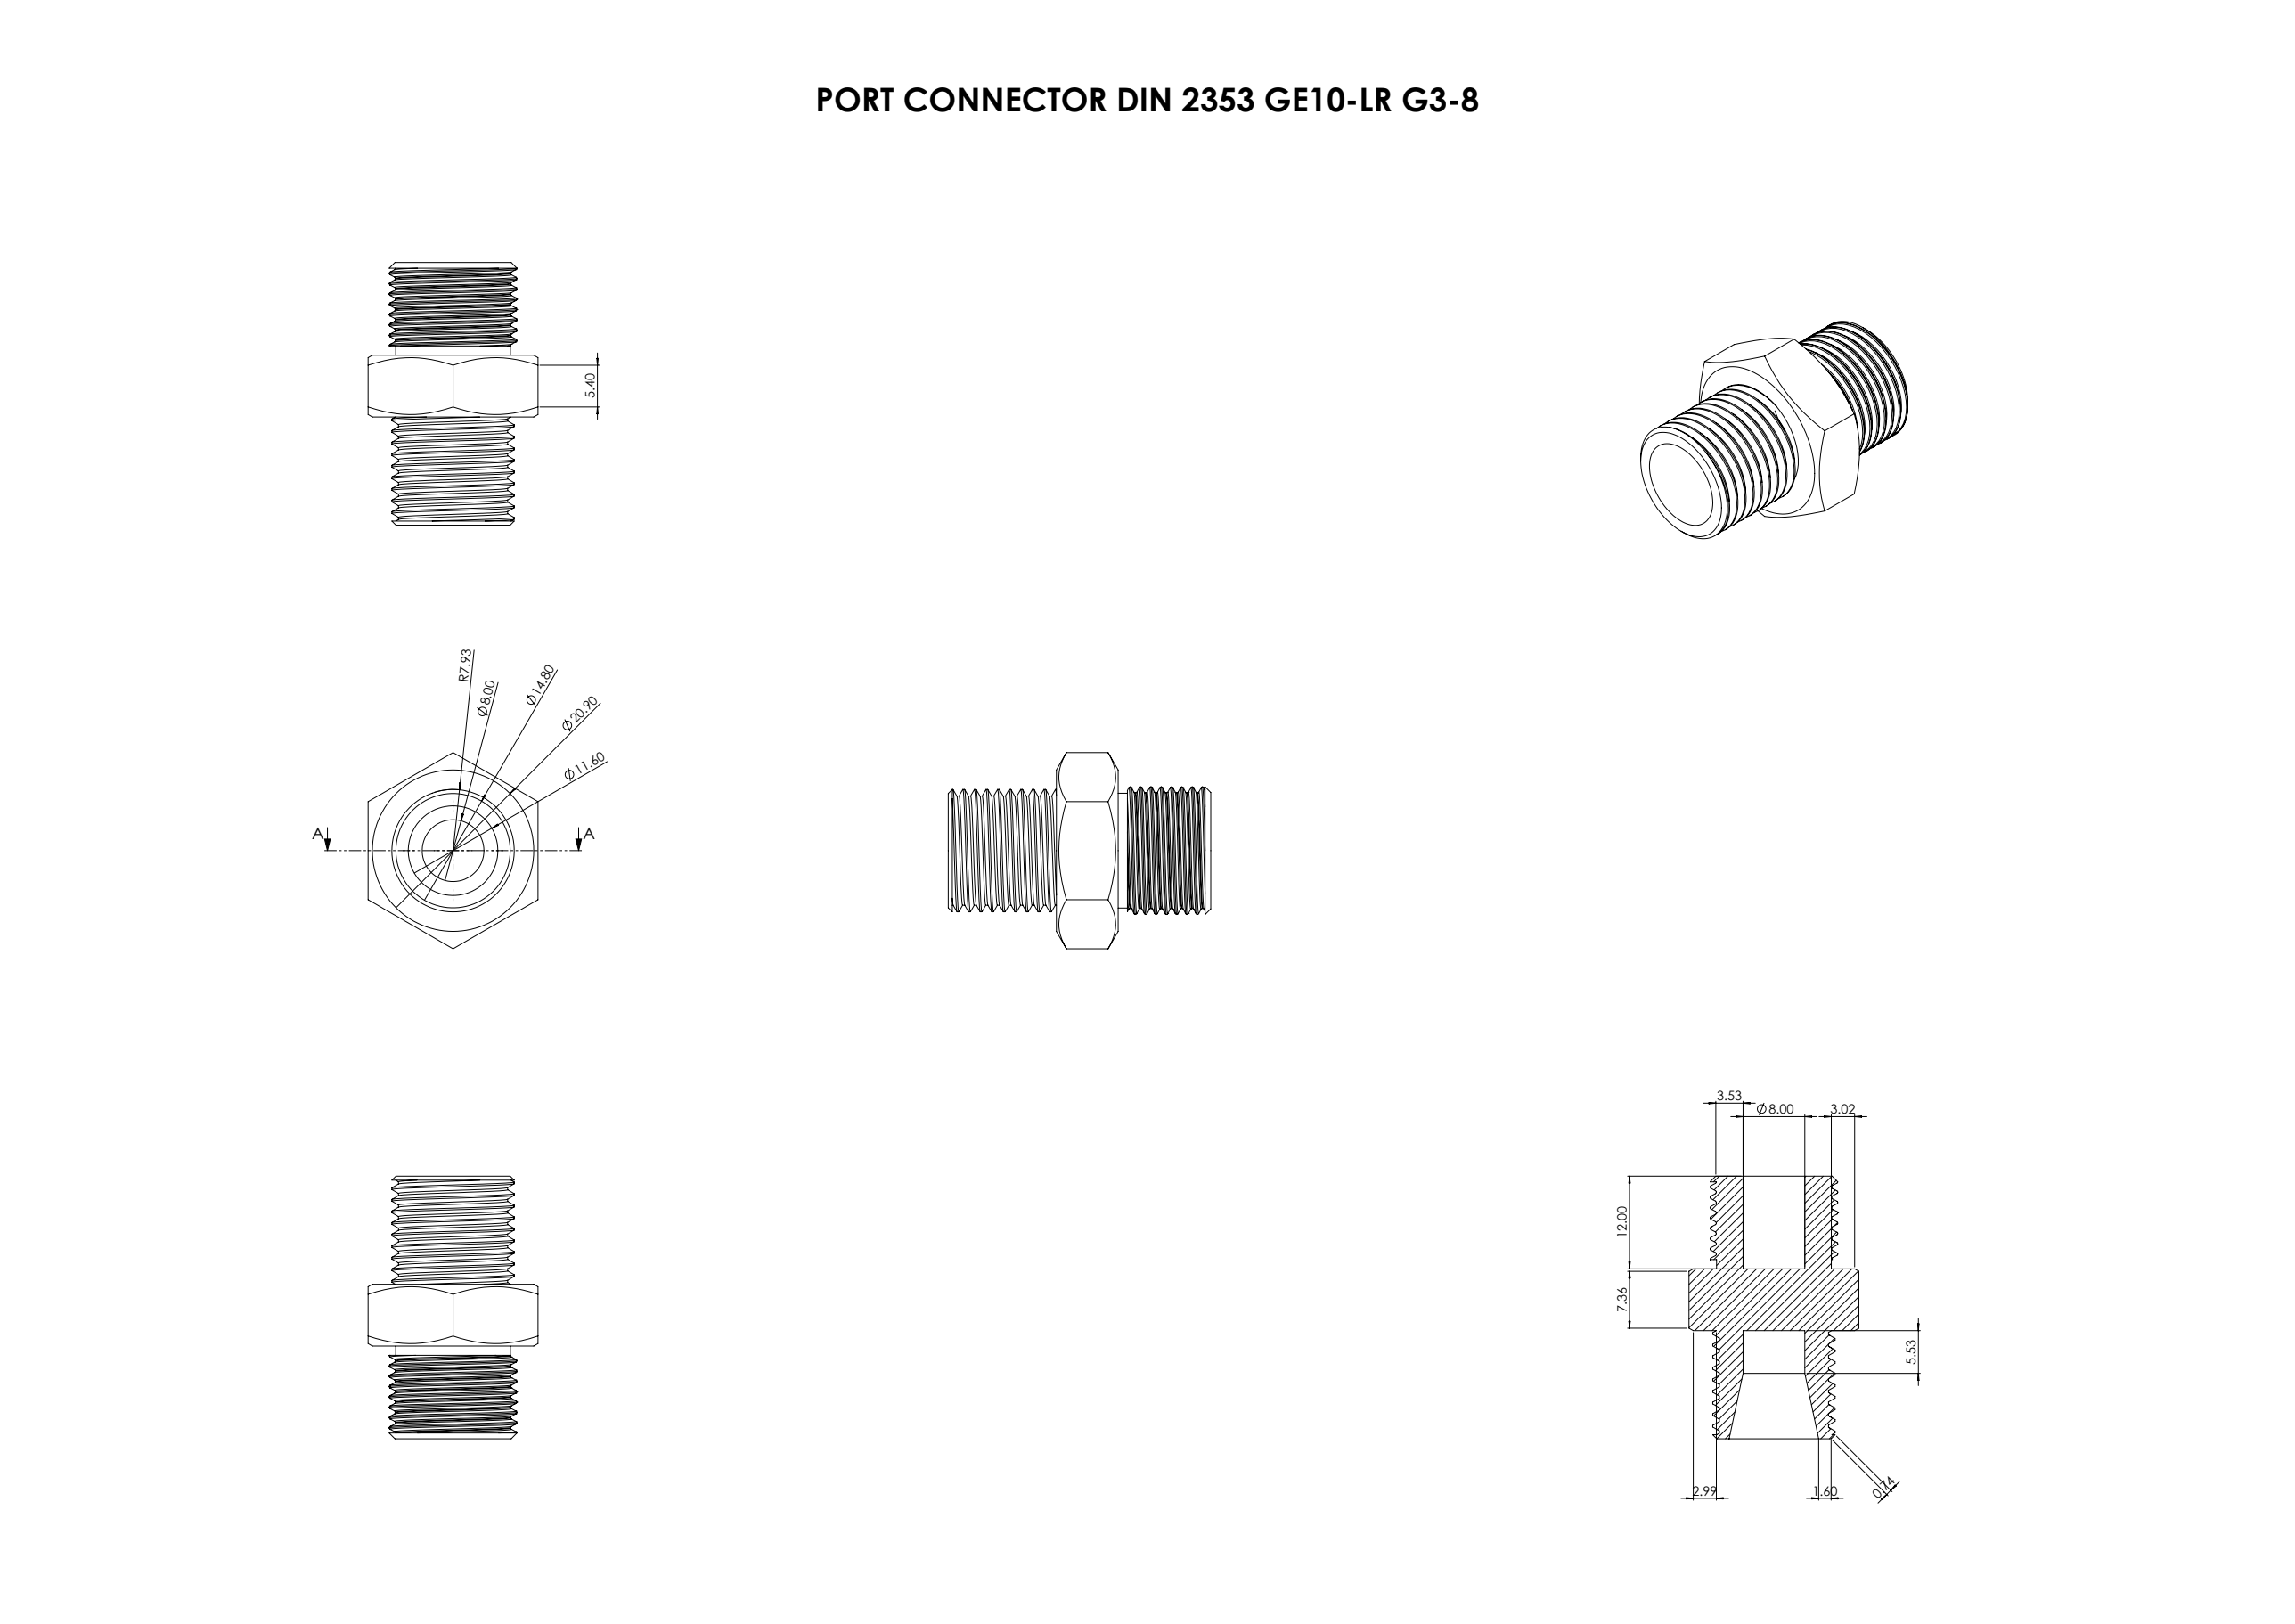
ISO-10303-21;
HEADER;
/* Generated by software containing ST-Developer
 * from STEP Tools, Inc. (www.steptools.com) 
 */

FILE_DESCRIPTION(
/* description */ (''),
/* implementation_level */ '2;1');

FILE_NAME(
/* name */ '20_Port_Connector_DIN_2353_GE10-LR_G3-8.step',
/* time_stamp */ '2026-10-23T00:52:27+05:00',
/* author */ (''),
/* organization */ (''),
/* preprocessor_version */ 'ST-DEVELOPER v20.2',
/* originating_system */ 'Autodesk Translation Framework v15.15.0.0',
/* authorisation */ '');

FILE_SCHEMA (('AUTOMOTIVE_DESIGN { 1 0 10303 214 3 1 1 }'));
ENDSEC;

DATA;
#10=MECHANICAL_DESIGN_GEOMETRIC_PRESENTATION_REPRESENTATION('',(#1574),#59204);
#561=B_SPLINE_SURFACE_WITH_KNOTS('',3,3,((#53988,#53989,#53990,#53991,#53992,
#53993,#53994,#53995,#53996,#53997,#53998,#53999,#54000,#54001,#54002,#54003,
#54004,#54005,#54006,#54007,#54008,#54009,#54010,#54011,#54012,#54013,#54014,
#54015,#54016,#54017,#54018,#54019,#54020,#54021,#54022,#54023,#54024,#54025,
#54026,#54027,#54028,#54029,#54030,#54031,#54032,#54033,#54034,#54035,#54036,
#54037,#54038,#54039,#54040,#54041,#54042,#54043,#54044,#54045,#54046,#54047,
#54048,#54049,#54050,#54051,#54052,#54053,#54054,#54055,#54056,#54057,#54058,
#54059,#54060,#54061,#54062,#54063,#54064,#54065,#54066,#54067,#54068,#54069,
#54070,#54071,#54072,#54073,#54074,#54075,#54076,#54077,#54078,#54079,#54080,
#54081,#54082,#54083,#54084,#54085,#54086,#54087,#54088,#54089,#54090,#54091,
#54092,#54093,#54094,#54095,#54096,#54097,#54098,#54099,#54100,#54101,#54102,
#54103,#54104,#54105,#54106,#54107,#54108),(#54109,#54110,#54111,#54112,
#54113,#54114,#54115,#54116,#54117,#54118,#54119,#54120,#54121,#54122,#54123,
#54124,#54125,#54126,#54127,#54128,#54129,#54130,#54131,#54132,#54133,#54134,
#54135,#54136,#54137,#54138,#54139,#54140,#54141,#54142,#54143,#54144,#54145,
#54146,#54147,#54148,#54149,#54150,#54151,#54152,#54153,#54154,#54155,#54156,
#54157,#54158,#54159,#54160,#54161,#54162,#54163,#54164,#54165,#54166,#54167,
#54168,#54169,#54170,#54171,#54172,#54173,#54174,#54175,#54176,#54177,#54178,
#54179,#54180,#54181,#54182,#54183,#54184,#54185,#54186,#54187,#54188,#54189,
#54190,#54191,#54192,#54193,#54194,#54195,#54196,#54197,#54198,#54199,#54200,
#54201,#54202,#54203,#54204,#54205,#54206,#54207,#54208,#54209,#54210,#54211,
#54212,#54213,#54214,#54215,#54216,#54217,#54218,#54219,#54220,#54221,#54222,
#54223,#54224,#54225,#54226,#54227,#54228,#54229),(#54230,#54231,#54232,
#54233,#54234,#54235,#54236,#54237,#54238,#54239,#54240,#54241,#54242,#54243,
#54244,#54245,#54246,#54247,#54248,#54249,#54250,#54251,#54252,#54253,#54254,
#54255,#54256,#54257,#54258,#54259,#54260,#54261,#54262,#54263,#54264,#54265,
#54266,#54267,#54268,#54269,#54270,#54271,#54272,#54273,#54274,#54275,#54276,
#54277,#54278,#54279,#54280,#54281,#54282,#54283,#54284,#54285,#54286,#54287,
#54288,#54289,#54290,#54291,#54292,#54293,#54294,#54295,#54296,#54297,#54298,
#54299,#54300,#54301,#54302,#54303,#54304,#54305,#54306,#54307,#54308,#54309,
#54310,#54311,#54312,#54313,#54314,#54315,#54316,#54317,#54318,#54319,#54320,
#54321,#54322,#54323,#54324,#54325,#54326,#54327,#54328,#54329,#54330,#54331,
#54332,#54333,#54334,#54335,#54336,#54337,#54338,#54339,#54340,#54341,#54342,
#54343,#54344,#54345,#54346,#54347,#54348,#54349,#54350),(#54351,#54352,
#54353,#54354,#54355,#54356,#54357,#54358,#54359,#54360,#54361,#54362,#54363,
#54364,#54365,#54366,#54367,#54368,#54369,#54370,#54371,#54372,#54373,#54374,
#54375,#54376,#54377,#54378,#54379,#54380,#54381,#54382,#54383,#54384,#54385,
#54386,#54387,#54388,#54389,#54390,#54391,#54392,#54393,#54394,#54395,#54396,
#54397,#54398,#54399,#54400,#54401,#54402,#54403,#54404,#54405,#54406,#54407,
#54408,#54409,#54410,#54411,#54412,#54413,#54414,#54415,#54416,#54417,#54418,
#54419,#54420,#54421,#54422,#54423,#54424,#54425,#54426,#54427,#54428,#54429,
#54430,#54431,#54432,#54433,#54434,#54435,#54436,#54437,#54438,#54439,#54440,
#54441,#54442,#54443,#54444,#54445,#54446,#54447,#54448,#54449,#54450,#54451,
#54452,#54453,#54454,#54455,#54456,#54457,#54458,#54459,#54460,#54461,#54462,
#54463,#54464,#54465,#54466,#54467,#54468,#54469,#54470,#54471)),
 .UNSPECIFIED.,.F.,.F.,.F.,(4,4),(4,1,1,1,1,1,1,1,1,1,1,1,1,1,1,1,1,1,1,
1,1,1,1,1,1,1,1,1,1,1,1,1,1,1,1,1,1,1,1,1,1,1,1,1,1,1,1,1,1,1,1,1,1,1,1,
1,1,1,1,1,1,1,1,1,1,1,1,1,1,1,1,1,1,1,1,1,1,1,1,1,1,1,1,1,1,1,1,1,1,1,1,
1,1,1,1,1,1,1,1,1,1,1,1,1,1,1,1,1,1,1,1,1,1,1,1,1,1,1,4),(0.,0.0989001011121828),
(8.30505915324875,8.80095158446445,9.29684401568014,9.79273644689584,10.2886288781115,
10.7845213093272,11.2804137405429,11.7763061717586,12.2721986029743,12.76809103419,
13.2639834654057,13.7598758966214,14.2557683278371,14.7516607590528,15.2475531902685,
15.7434456214842,16.2393380526999,16.7352304839156,17.2311229151313,17.727015346347,
18.2229077775627,18.7188002087784,19.2146926399941,19.7105850712098,20.2064775024255,
20.7023699336412,21.1982623648568,21.6941547960725,22.1900472272882,22.6859396585039,
23.1818320897196,23.6777245209353,24.173616952151,24.6695093833667,25.1654018145824,
25.6612942457981,26.1571866770138,26.6530791082295,27.1489715394452,27.6448639706609,
28.1407564018766,28.6366488330923,29.132541264308,29.6284336955237,30.1243261267394,
30.6202185579551,31.1161109891708,31.6120034203865,32.1078958516022,32.6037882828178,
33.0996807140335,33.5955731452492,34.0914655764649,34.5873580076806,35.0832504388963,
35.579142870112,36.0750353013277,36.5709277325434,37.0668201637591,37.5627125949748,
38.0586050261905,38.5544974574062,39.0503898886219,39.5462823198376,40.0421747510533,
40.538067182269,41.0339596134847,41.5298520447004,42.0257444759161,42.5216369071318,
43.0175293383475,43.5134217695632,44.0093142007789,44.5052066319946,45.0010990632102,
45.4969914944259,45.9928839256416,46.4887763568573,46.984668788073,47.4805612192887,
47.9764536505044,48.4723460817201,48.9682385129358,49.4641309441515,49.9600233753672,
50.4559158065829,50.9518082377986,51.4477006690143,51.94359310023,52.4394855314457,
52.9353779626614,53.4312703938771,53.9271628250928,54.4230552563085,54.9189476875242,
55.4148401187399,55.9107325499556,56.4066249811712,56.9025174123869,57.3984098436026,
57.8943022748183,58.390194706034,58.8860871372497,59.3819795684654,59.8778719996811,
60.3737644308968,60.8696568621125,61.3655492933282,61.8614417245439,62.3573341557596,
62.8532265869753,63.349119018191,63.8450114494067,64.3409038806224,64.8367963118381,
65.3326887430538,65.8285811742695,66.3244736054852,66.8203660367009),
 .UNSPECIFIED.);
#562=B_SPLINE_SURFACE_WITH_KNOTS('',3,3,((#54612,#54613,#54614,#54615,#54616,
#54617,#54618,#54619,#54620,#54621,#54622,#54623,#54624,#54625,#54626,#54627,
#54628,#54629,#54630,#54631,#54632,#54633,#54634,#54635,#54636,#54637,#54638,
#54639,#54640,#54641,#54642,#54643,#54644,#54645,#54646,#54647,#54648,#54649,
#54650,#54651,#54652,#54653,#54654,#54655,#54656,#54657,#54658,#54659,#54660,
#54661,#54662,#54663,#54664,#54665,#54666,#54667,#54668,#54669,#54670,#54671,
#54672,#54673,#54674,#54675,#54676,#54677,#54678,#54679,#54680,#54681,#54682,
#54683,#54684,#54685,#54686,#54687,#54688,#54689,#54690,#54691,#54692,#54693,
#54694,#54695,#54696,#54697,#54698,#54699,#54700,#54701,#54702,#54703,#54704,
#54705,#54706,#54707,#54708,#54709,#54710,#54711,#54712,#54713,#54714,#54715,
#54716,#54717,#54718,#54719,#54720,#54721,#54722,#54723,#54724,#54725,#54726,
#54727,#54728,#54729,#54730,#54731,#54732),(#54733,#54734,#54735,#54736,
#54737,#54738,#54739,#54740,#54741,#54742,#54743,#54744,#54745,#54746,#54747,
#54748,#54749,#54750,#54751,#54752,#54753,#54754,#54755,#54756,#54757,#54758,
#54759,#54760,#54761,#54762,#54763,#54764,#54765,#54766,#54767,#54768,#54769,
#54770,#54771,#54772,#54773,#54774,#54775,#54776,#54777,#54778,#54779,#54780,
#54781,#54782,#54783,#54784,#54785,#54786,#54787,#54788,#54789,#54790,#54791,
#54792,#54793,#54794,#54795,#54796,#54797,#54798,#54799,#54800,#54801,#54802,
#54803,#54804,#54805,#54806,#54807,#54808,#54809,#54810,#54811,#54812,#54813,
#54814,#54815,#54816,#54817,#54818,#54819,#54820,#54821,#54822,#54823,#54824,
#54825,#54826,#54827,#54828,#54829,#54830,#54831,#54832,#54833,#54834,#54835,
#54836,#54837,#54838,#54839,#54840,#54841,#54842,#54843,#54844,#54845,#54846,
#54847,#54848,#54849,#54850,#54851,#54852,#54853),(#54854,#54855,#54856,
#54857,#54858,#54859,#54860,#54861,#54862,#54863,#54864,#54865,#54866,#54867,
#54868,#54869,#54870,#54871,#54872,#54873,#54874,#54875,#54876,#54877,#54878,
#54879,#54880,#54881,#54882,#54883,#54884,#54885,#54886,#54887,#54888,#54889,
#54890,#54891,#54892,#54893,#54894,#54895,#54896,#54897,#54898,#54899,#54900,
#54901,#54902,#54903,#54904,#54905,#54906,#54907,#54908,#54909,#54910,#54911,
#54912,#54913,#54914,#54915,#54916,#54917,#54918,#54919,#54920,#54921,#54922,
#54923,#54924,#54925,#54926,#54927,#54928,#54929,#54930,#54931,#54932,#54933,
#54934,#54935,#54936,#54937,#54938,#54939,#54940,#54941,#54942,#54943,#54944,
#54945,#54946,#54947,#54948,#54949,#54950,#54951,#54952,#54953,#54954,#54955,
#54956,#54957,#54958,#54959,#54960,#54961,#54962,#54963,#54964,#54965,#54966,
#54967,#54968,#54969,#54970,#54971,#54972,#54973,#54974),(#54975,#54976,
#54977,#54978,#54979,#54980,#54981,#54982,#54983,#54984,#54985,#54986,#54987,
#54988,#54989,#54990,#54991,#54992,#54993,#54994,#54995,#54996,#54997,#54998,
#54999,#55000,#55001,#55002,#55003,#55004,#55005,#55006,#55007,#55008,#55009,
#55010,#55011,#55012,#55013,#55014,#55015,#55016,#55017,#55018,#55019,#55020,
#55021,#55022,#55023,#55024,#55025,#55026,#55027,#55028,#55029,#55030,#55031,
#55032,#55033,#55034,#55035,#55036,#55037,#55038,#55039,#55040,#55041,#55042,
#55043,#55044,#55045,#55046,#55047,#55048,#55049,#55050,#55051,#55052,#55053,
#55054,#55055,#55056,#55057,#55058,#55059,#55060,#55061,#55062,#55063,#55064,
#55065,#55066,#55067,#55068,#55069,#55070,#55071,#55072,#55073,#55074,#55075,
#55076,#55077,#55078,#55079,#55080,#55081,#55082,#55083,#55084,#55085,#55086,
#55087,#55088,#55089,#55090,#55091,#55092,#55093,#55094,#55095)),
 .UNSPECIFIED.,.F.,.F.,.F.,(4,4),(4,1,1,1,1,1,1,1,1,1,1,1,1,1,1,1,1,1,1,
1,1,1,1,1,1,1,1,1,1,1,1,1,1,1,1,1,1,1,1,1,1,1,1,1,1,1,1,1,1,1,1,1,1,1,1,
1,1,1,1,1,1,1,1,1,1,1,1,1,1,1,1,1,1,1,1,1,1,1,1,1,1,1,1,1,1,1,1,1,1,1,1,
1,1,1,1,1,1,1,1,1,1,1,1,1,1,1,1,1,1,1,1,1,1,1,1,1,1,1,4),(0.,0.0989001011121828),
(11.6147305479242,12.1106229791399,12.6065154103556,13.1024078415713,13.598300272787,
14.0941927040027,14.5900851352184,15.0859775664341,15.5818699976498,16.0777624288655,
16.5736548600812,17.0695472912969,17.5654397225126,18.0613321537283,18.557224584944,
19.0531170161597,19.5490094473754,20.0449018785911,20.5407943098068,21.0366867410225,
21.5325791722382,22.0284716034539,22.5243640346695,23.0202564658852,23.5161488971009,
24.0120413283166,24.5079337595323,25.003826190748,25.4997186219637,25.9956110531794,
26.4915034843951,26.9873959156108,27.4832883468265,27.9791807780422,28.4750732092579,
28.9709656404736,29.4668580716893,29.962750502905,30.4586429341207,30.9545353653364,
31.4504277965521,31.9463202277678,32.4422126589835,32.9381050901992,33.4339975214149,
33.9298899526305,34.4257823838462,34.9216748150619,35.4175672462776,35.9134596774933,
36.409352108709,36.9052445399247,37.4011369711404,37.8970294023561,38.3929218335718,
38.8888142647875,39.3847066960032,39.8805991272189,40.3764915584346,40.8723839896503,
41.368276420866,41.8641688520817,42.3600612832974,42.8559537145131,43.3518461457288,
43.8477385769445,44.3436310081602,44.8395234393758,45.3354158705915,45.8313083018072,
46.3272007330229,46.8230931642386,47.3189855954543,47.81487802667,48.3107704578857,
48.8066628891014,49.3025553203171,49.7984477515328,50.2943401827485,50.7902326139642,
51.2861250451799,51.7820174763956,52.2779099076113,52.773802338827,53.2696947700427,
53.7655872012584,54.2614796324741,54.7573720636898,55.2532644949055,55.7491569261211,
56.2450493573368,56.7409417885525,57.2368342197682,57.7327266509839,58.2286190821996,
58.7245115134153,59.220403944631,59.7162963758467,60.2121888070624,60.7080812382781,
61.2039736694938,61.6998661007095,62.1957585319252,62.6916509631409,63.1875433943566,
63.6834358255723,64.179328256788,64.6752206880037,65.1711131192194,65.6670055504351,
66.1628979816508,66.6587904128665,67.1546828440821,67.6505752752978,68.1464677065135,
68.6423601377292,69.1382525689449,69.6341450001606,70.1300374313763),
 .UNSPECIFIED.);
#563=B_SPLINE_SURFACE_WITH_KNOTS('',3,3,((#55202,#55203,#55204,#55205,#55206,
#55207,#55208,#55209,#55210,#55211,#55212,#55213,#55214,#55215,#55216,#55217,
#55218,#55219,#55220,#55221,#55222,#55223,#55224,#55225,#55226,#55227,#55228,
#55229,#55230,#55231,#55232,#55233,#55234,#55235,#55236,#55237,#55238,#55239,
#55240,#55241,#55242,#55243,#55244,#55245,#55246,#55247,#55248,#55249,#55250,
#55251,#55252,#55253,#55254,#55255,#55256,#55257,#55258,#55259,#55260,#55261,
#55262,#55263,#55264,#55265,#55266,#55267,#55268,#55269,#55270,#55271,#55272,
#55273,#55274,#55275,#55276,#55277,#55278,#55279,#55280,#55281,#55282,#55283,
#55284,#55285,#55286,#55287,#55288,#55289,#55290,#55291,#55292,#55293,#55294,
#55295,#55296,#55297,#55298,#55299,#55300,#55301,#55302),(#55303,#55304,
#55305,#55306,#55307,#55308,#55309,#55310,#55311,#55312,#55313,#55314,#55315,
#55316,#55317,#55318,#55319,#55320,#55321,#55322,#55323,#55324,#55325,#55326,
#55327,#55328,#55329,#55330,#55331,#55332,#55333,#55334,#55335,#55336,#55337,
#55338,#55339,#55340,#55341,#55342,#55343,#55344,#55345,#55346,#55347,#55348,
#55349,#55350,#55351,#55352,#55353,#55354,#55355,#55356,#55357,#55358,#55359,
#55360,#55361,#55362,#55363,#55364,#55365,#55366,#55367,#55368,#55369,#55370,
#55371,#55372,#55373,#55374,#55375,#55376,#55377,#55378,#55379,#55380,#55381,
#55382,#55383,#55384,#55385,#55386,#55387,#55388,#55389,#55390,#55391,#55392,
#55393,#55394,#55395,#55396,#55397,#55398,#55399,#55400,#55401,#55402,#55403),
(#55404,#55405,#55406,#55407,#55408,#55409,#55410,#55411,#55412,#55413,
#55414,#55415,#55416,#55417,#55418,#55419,#55420,#55421,#55422,#55423,#55424,
#55425,#55426,#55427,#55428,#55429,#55430,#55431,#55432,#55433,#55434,#55435,
#55436,#55437,#55438,#55439,#55440,#55441,#55442,#55443,#55444,#55445,#55446,
#55447,#55448,#55449,#55450,#55451,#55452,#55453,#55454,#55455,#55456,#55457,
#55458,#55459,#55460,#55461,#55462,#55463,#55464,#55465,#55466,#55467,#55468,
#55469,#55470,#55471,#55472,#55473,#55474,#55475,#55476,#55477,#55478,#55479,
#55480,#55481,#55482,#55483,#55484,#55485,#55486,#55487,#55488,#55489,#55490,
#55491,#55492,#55493,#55494,#55495,#55496,#55497,#55498,#55499,#55500,#55501,
#55502,#55503,#55504),(#55505,#55506,#55507,#55508,#55509,#55510,#55511,
#55512,#55513,#55514,#55515,#55516,#55517,#55518,#55519,#55520,#55521,#55522,
#55523,#55524,#55525,#55526,#55527,#55528,#55529,#55530,#55531,#55532,#55533,
#55534,#55535,#55536,#55537,#55538,#55539,#55540,#55541,#55542,#55543,#55544,
#55545,#55546,#55547,#55548,#55549,#55550,#55551,#55552,#55553,#55554,#55555,
#55556,#55557,#55558,#55559,#55560,#55561,#55562,#55563,#55564,#55565,#55566,
#55567,#55568,#55569,#55570,#55571,#55572,#55573,#55574,#55575,#55576,#55577,
#55578,#55579,#55580,#55581,#55582,#55583,#55584,#55585,#55586,#55587,#55588,
#55589,#55590,#55591,#55592,#55593,#55594,#55595,#55596,#55597,#55598,#55599,
#55600,#55601,#55602,#55603,#55604,#55605),(#55606,#55607,#55608,#55609,
#55610,#55611,#55612,#55613,#55614,#55615,#55616,#55617,#55618,#55619,#55620,
#55621,#55622,#55623,#55624,#55625,#55626,#55627,#55628,#55629,#55630,#55631,
#55632,#55633,#55634,#55635,#55636,#55637,#55638,#55639,#55640,#55641,#55642,
#55643,#55644,#55645,#55646,#55647,#55648,#55649,#55650,#55651,#55652,#55653,
#55654,#55655,#55656,#55657,#55658,#55659,#55660,#55661,#55662,#55663,#55664,
#55665,#55666,#55667,#55668,#55669,#55670,#55671,#55672,#55673,#55674,#55675,
#55676,#55677,#55678,#55679,#55680,#55681,#55682,#55683,#55684,#55685,#55686,
#55687,#55688,#55689,#55690,#55691,#55692,#55693,#55694,#55695,#55696,#55697,
#55698,#55699,#55700,#55701,#55702,#55703,#55704,#55705,#55706)),
 .UNSPECIFIED.,.F.,.F.,.F.,(4,1,4),(4,1,1,1,1,1,1,1,1,1,1,1,1,1,1,1,1,1,
1,1,1,1,1,1,1,1,1,1,1,1,1,1,1,1,1,1,1,1,1,1,1,1,1,1,1,1,1,1,1,1,1,1,1,1,
1,1,1,1,1,1,1,1,1,1,1,1,1,1,1,1,1,1,1,1,1,1,1,1,1,1,1,1,1,1,1,1,1,1,1,1,
1,1,1,1,1,1,1,1,4),(0.,0.467498906784196,1.09083078249646),(6.28318530717955,
6.77358368901883,7.26398207085812,7.7543804526974,8.24477883453668,8.73517721637597,
9.22557559821525,9.71597398005454,10.2063723618938,10.6967707437331,11.1871691255724,
11.6775675074117,12.167965889251,12.6583642710902,13.1487626529295,13.6391610347688,
14.1295594166081,14.6199577984474,15.1103561802867,15.6007545621259,16.0911529439652,
16.5815513258045,17.0719497076438,17.5623480894831,18.0527464713224,18.5431448531616,
19.0335432350009,19.5239416168402,20.0143399986795,20.5047383805188,20.9951367623581,
21.4855351441973,21.9759335260366,22.4663319078759,22.9567302897152,23.4471286715545,
23.9375270533938,24.427925435233,24.9183238170723,25.4087221989116,25.8991205807509,
26.3895189625902,26.8799173444295,27.3703157262687,27.860714108108,28.3511124899473,
28.8415108717866,29.3319092536259,29.8223076354652,30.3127060173044,30.8031043991437,
31.293502780983,31.7839011628223,32.2742995446616,32.7646979265009,33.2550963083402,
33.7454946901794,34.2358930720187,34.726291453858,35.2166898356973,35.7070882175366,
36.1974865993759,36.6878849812151,37.1782833630544,37.6686817448937,38.159080126733,
38.6494785085723,39.1398768904116,39.6302752722508,40.1206736540901,40.6110720359294,
41.1014704177687,41.591868799608,42.0822671814473,42.5726655632865,43.0630639451258,
43.5534623269651,44.0438607088044,44.5342590906437,45.024657472483,45.5150558543222,
46.0054542361615,46.4958526180008,46.9862509998401,47.4766493816794,47.9670477635187,
48.457446145358,48.9478445271972,49.4382429090365,49.9286412908758,50.4190396727151,
50.9094380545544,51.3998364363937,51.8902348182329,52.3806332000722,52.8710315819115,
53.3614299637508,53.8518283455901,54.3422267274294),.UNSPECIFIED.);
#564=B_SPLINE_SURFACE_WITH_KNOTS('',3,3,((#56119,#56120,#56121,#56122,#56123,
#56124,#56125,#56126,#56127,#56128,#56129,#56130,#56131,#56132,#56133,#56134,
#56135,#56136,#56137,#56138,#56139,#56140,#56141,#56142,#56143,#56144,#56145,
#56146,#56147,#56148,#56149,#56150,#56151,#56152,#56153,#56154,#56155,#56156,
#56157,#56158,#56159,#56160,#56161,#56162,#56163,#56164,#56165,#56166,#56167,
#56168,#56169,#56170,#56171,#56172,#56173,#56174,#56175,#56176,#56177,#56178,
#56179,#56180,#56181,#56182,#56183,#56184,#56185,#56186,#56187,#56188,#56189,
#56190,#56191,#56192,#56193,#56194,#56195,#56196,#56197,#56198,#56199,#56200,
#56201,#56202,#56203,#56204,#56205,#56206,#56207,#56208,#56209,#56210,#56211,
#56212,#56213,#56214,#56215,#56216,#56217,#56218,#56219),(#56220,#56221,
#56222,#56223,#56224,#56225,#56226,#56227,#56228,#56229,#56230,#56231,#56232,
#56233,#56234,#56235,#56236,#56237,#56238,#56239,#56240,#56241,#56242,#56243,
#56244,#56245,#56246,#56247,#56248,#56249,#56250,#56251,#56252,#56253,#56254,
#56255,#56256,#56257,#56258,#56259,#56260,#56261,#56262,#56263,#56264,#56265,
#56266,#56267,#56268,#56269,#56270,#56271,#56272,#56273,#56274,#56275,#56276,
#56277,#56278,#56279,#56280,#56281,#56282,#56283,#56284,#56285,#56286,#56287,
#56288,#56289,#56290,#56291,#56292,#56293,#56294,#56295,#56296,#56297,#56298,
#56299,#56300,#56301,#56302,#56303,#56304,#56305,#56306,#56307,#56308,#56309,
#56310,#56311,#56312,#56313,#56314,#56315,#56316,#56317,#56318,#56319,#56320),
(#56321,#56322,#56323,#56324,#56325,#56326,#56327,#56328,#56329,#56330,
#56331,#56332,#56333,#56334,#56335,#56336,#56337,#56338,#56339,#56340,#56341,
#56342,#56343,#56344,#56345,#56346,#56347,#56348,#56349,#56350,#56351,#56352,
#56353,#56354,#56355,#56356,#56357,#56358,#56359,#56360,#56361,#56362,#56363,
#56364,#56365,#56366,#56367,#56368,#56369,#56370,#56371,#56372,#56373,#56374,
#56375,#56376,#56377,#56378,#56379,#56380,#56381,#56382,#56383,#56384,#56385,
#56386,#56387,#56388,#56389,#56390,#56391,#56392,#56393,#56394,#56395,#56396,
#56397,#56398,#56399,#56400,#56401,#56402,#56403,#56404,#56405,#56406,#56407,
#56408,#56409,#56410,#56411,#56412,#56413,#56414,#56415,#56416,#56417,#56418,
#56419,#56420,#56421),(#56422,#56423,#56424,#56425,#56426,#56427,#56428,
#56429,#56430,#56431,#56432,#56433,#56434,#56435,#56436,#56437,#56438,#56439,
#56440,#56441,#56442,#56443,#56444,#56445,#56446,#56447,#56448,#56449,#56450,
#56451,#56452,#56453,#56454,#56455,#56456,#56457,#56458,#56459,#56460,#56461,
#56462,#56463,#56464,#56465,#56466,#56467,#56468,#56469,#56470,#56471,#56472,
#56473,#56474,#56475,#56476,#56477,#56478,#56479,#56480,#56481,#56482,#56483,
#56484,#56485,#56486,#56487,#56488,#56489,#56490,#56491,#56492,#56493,#56494,
#56495,#56496,#56497,#56498,#56499,#56500,#56501,#56502,#56503,#56504,#56505,
#56506,#56507,#56508,#56509,#56510,#56511,#56512,#56513,#56514,#56515,#56516,
#56517,#56518,#56519,#56520,#56521,#56522)),.UNSPECIFIED.,.F.,.F.,.F.,(4,
4),(4,1,1,1,1,1,1,1,1,1,1,1,1,1,1,1,1,1,1,1,1,1,1,1,1,1,1,1,1,1,1,1,1,1,
1,1,1,1,1,1,1,1,1,1,1,1,1,1,1,1,1,1,1,1,1,1,1,1,1,1,1,1,1,1,1,1,1,1,1,1,
1,1,1,1,1,1,1,1,1,1,1,1,1,1,1,1,1,1,1,1,1,1,1,1,1,1,1,1,4),(0.,0.0671853436149873),
(7.04827039213812,7.54574010072061,8.0432098093031,8.54067951788559,9.03814922646808,
9.53561893505058,10.0330886436331,10.5305583522156,11.028028060798,11.5254977693805,
12.022967477963,12.5204371865455,13.017906895128,13.5153766037105,14.012846312293,
14.5103160208755,15.007785729458,15.5052554380405,16.002725146623,16.5001948552054,
16.9976645637879,17.4951342723704,17.9926039809529,18.4900736895354,18.9875433981179,
19.4850131067004,19.9824828152829,20.4799525238654,20.9774222324479,21.4748919410303,
21.9723616496128,22.4698313581953,22.9673010667778,23.4647707753603,23.9622404839428,
24.4597101925253,24.9571799011078,25.4546496096903,25.9521193182728,26.4495890268552,
26.9470587354377,27.4445284440202,27.9419981526027,28.4394678611852,28.9369375697677,
29.4344072783502,29.9318769869327,30.4293466955152,30.9268164040977,31.4242861126801,
31.9217558212626,32.4192255298451,32.9166952384276,33.4141649470101,33.9116346555926,
34.4091043641751,34.9065740727576,35.4040437813401,35.9015134899226,36.3989831985051,
36.8964529070875,37.39392261567,37.8913923242525,38.388862032835,38.8863317414175,
39.38380145,39.8812711585825,40.378740867165,40.8762105757475,41.37368028433,
41.8711499929124,42.3686197014949,42.8660894100774,43.3635591186599,43.8610288272424,
44.3584985358249,44.8559682444074,45.3534379529899,45.8509076615724,46.3483773701549,
46.8458470787373,47.3433167873198,47.8407864959023,48.3382562044848,48.8357259130673,
49.3331956216498,49.8306653302323,50.3281350388148,50.8256047473973,51.3230744559798,
51.8205441645622,52.3180138731447,52.8154835817272,53.3129532903097,53.8104229988922,
54.3078927074747,54.8053624160572,55.3028321246397,55.8003018332222),
 .UNSPECIFIED.);
#565=B_SPLINE_SURFACE_WITH_KNOTS('',3,3,((#56725,#56726,#56727,#56728,#56729,
#56730,#56731,#56732,#56733,#56734,#56735,#56736,#56737,#56738,#56739,#56740,
#56741,#56742,#56743,#56744,#56745,#56746,#56747,#56748,#56749,#56750,#56751,
#56752,#56753,#56754,#56755,#56756,#56757,#56758,#56759,#56760,#56761,#56762,
#56763,#56764,#56765,#56766,#56767,#56768,#56769,#56770,#56771,#56772,#56773,
#56774,#56775,#56776,#56777,#56778,#56779,#56780,#56781,#56782,#56783,#56784,
#56785,#56786,#56787,#56788,#56789,#56790,#56791,#56792,#56793,#56794,#56795,
#56796,#56797,#56798,#56799,#56800,#56801,#56802,#56803,#56804,#56805,#56806,
#56807,#56808,#56809,#56810,#56811,#56812,#56813,#56814,#56815,#56816,#56817,
#56818,#56819,#56820,#56821,#56822,#56823,#56824,#56825),(#56826,#56827,
#56828,#56829,#56830,#56831,#56832,#56833,#56834,#56835,#56836,#56837,#56838,
#56839,#56840,#56841,#56842,#56843,#56844,#56845,#56846,#56847,#56848,#56849,
#56850,#56851,#56852,#56853,#56854,#56855,#56856,#56857,#56858,#56859,#56860,
#56861,#56862,#56863,#56864,#56865,#56866,#56867,#56868,#56869,#56870,#56871,
#56872,#56873,#56874,#56875,#56876,#56877,#56878,#56879,#56880,#56881,#56882,
#56883,#56884,#56885,#56886,#56887,#56888,#56889,#56890,#56891,#56892,#56893,
#56894,#56895,#56896,#56897,#56898,#56899,#56900,#56901,#56902,#56903,#56904,
#56905,#56906,#56907,#56908,#56909,#56910,#56911,#56912,#56913,#56914,#56915,
#56916,#56917,#56918,#56919,#56920,#56921,#56922,#56923,#56924,#56925,#56926),
(#56927,#56928,#56929,#56930,#56931,#56932,#56933,#56934,#56935,#56936,
#56937,#56938,#56939,#56940,#56941,#56942,#56943,#56944,#56945,#56946,#56947,
#56948,#56949,#56950,#56951,#56952,#56953,#56954,#56955,#56956,#56957,#56958,
#56959,#56960,#56961,#56962,#56963,#56964,#56965,#56966,#56967,#56968,#56969,
#56970,#56971,#56972,#56973,#56974,#56975,#56976,#56977,#56978,#56979,#56980,
#56981,#56982,#56983,#56984,#56985,#56986,#56987,#56988,#56989,#56990,#56991,
#56992,#56993,#56994,#56995,#56996,#56997,#56998,#56999,#57000,#57001,#57002,
#57003,#57004,#57005,#57006,#57007,#57008,#57009,#57010,#57011,#57012,#57013,
#57014,#57015,#57016,#57017,#57018,#57019,#57020,#57021,#57022,#57023,#57024,
#57025,#57026,#57027),(#57028,#57029,#57030,#57031,#57032,#57033,#57034,
#57035,#57036,#57037,#57038,#57039,#57040,#57041,#57042,#57043,#57044,#57045,
#57046,#57047,#57048,#57049,#57050,#57051,#57052,#57053,#57054,#57055,#57056,
#57057,#57058,#57059,#57060,#57061,#57062,#57063,#57064,#57065,#57066,#57067,
#57068,#57069,#57070,#57071,#57072,#57073,#57074,#57075,#57076,#57077,#57078,
#57079,#57080,#57081,#57082,#57083,#57084,#57085,#57086,#57087,#57088,#57089,
#57090,#57091,#57092,#57093,#57094,#57095,#57096,#57097,#57098,#57099,#57100,
#57101,#57102,#57103,#57104,#57105,#57106,#57107,#57108,#57109,#57110,#57111,
#57112,#57113,#57114,#57115,#57116,#57117,#57118,#57119,#57120,#57121,#57122,
#57123,#57124,#57125,#57126,#57127,#57128),(#57129,#57130,#57131,#57132,
#57133,#57134,#57135,#57136,#57137,#57138,#57139,#57140,#57141,#57142,#57143,
#57144,#57145,#57146,#57147,#57148,#57149,#57150,#57151,#57152,#57153,#57154,
#57155,#57156,#57157,#57158,#57159,#57160,#57161,#57162,#57163,#57164,#57165,
#57166,#57167,#57168,#57169,#57170,#57171,#57172,#57173,#57174,#57175,#57176,
#57177,#57178,#57179,#57180,#57181,#57182,#57183,#57184,#57185,#57186,#57187,
#57188,#57189,#57190,#57191,#57192,#57193,#57194,#57195,#57196,#57197,#57198,
#57199,#57200,#57201,#57202,#57203,#57204,#57205,#57206,#57207,#57208,#57209,
#57210,#57211,#57212,#57213,#57214,#57215,#57216,#57217,#57218,#57219,#57220,
#57221,#57222,#57223,#57224,#57225,#57226,#57227,#57228,#57229)),
 .UNSPECIFIED.,.F.,.F.,.F.,(4,1,4),(4,1,1,1,1,1,1,1,1,1,1,1,1,1,1,1,1,1,
1,1,1,1,1,1,1,1,1,1,1,1,1,1,1,1,1,1,1,1,1,1,1,1,1,1,1,1,1,1,1,1,1,1,1,1,
1,1,1,1,1,1,1,1,1,1,1,1,1,1,1,1,1,1,1,1,1,1,1,1,1,1,1,1,1,1,1,1,1,1,1,1,
1,1,1,1,1,1,1,1,4),(0.,0.467498906784196,1.09083078249646),(8.50634549793093,
8.99674387977021,9.4871422616095,9.97754064344878,10.4679390252881,10.9583374071273,
11.4487357889666,11.9391341708059,12.4295325526452,12.9199309344845,13.4103293163238,
13.9007276981631,14.3911260800023,14.8815244618416,15.3719228436809,15.8623212255202,
16.3527196073595,16.8431179891988,17.333516371038,17.8239147528773,18.3143131347166,
18.8047115165559,19.2951098983952,19.7855082802345,20.2759066620737,20.766305043913,
21.2567034257523,21.7471018075916,22.2375001894309,22.7278985712702,23.2182969531094,
23.7086953349487,24.199093716788,24.6894920986273,25.1798904804666,25.6702888623059,
26.1606872441451,26.6510856259844,27.1414840078237,27.631882389663,28.1222807715023,
28.6126791533416,29.1030775351808,29.5934759170201,30.0838742988594,30.5742726806987,
31.064671062538,31.5550694443773,32.0454678262166,32.5358662080558,33.0262645898951,
33.5166629717344,34.0070613535737,34.497459735413,34.9878581172523,35.4782564990915,
35.9686548809308,36.4590532627701,36.9494516446094,37.4398500264487,37.930248408288,
38.4206467901272,38.9110451719665,39.4014435538058,39.8918419356451,40.3822403174844,
40.8726386993237,41.3630370811629,41.8534354630022,42.3438338448415,42.8342322266808,
43.3246306085201,43.8150289903594,44.3054273721986,44.7958257540379,45.2862241358772,
45.7766225177165,46.2670208995558,46.7574192813951,47.2478176632343,47.7382160450736,
48.2286144269129,48.7190128087522,49.2094111905915,49.6998095724308,50.1902079542701,
50.6806063361093,51.1710047179486,51.6614030997879,52.1518014816272,52.6421998634665,
53.1325982453058,53.622996627145,54.1133950089843,54.6037933908236,55.0941917726629,
55.5845901545022,56.0749885363415,56.5653869181807),.UNSPECIFIED.);
#566=B_SPLINE_SURFACE_WITH_KNOTS('',3,3,((#57322,#57323,#57324,#57325,#57326,
#57327,#57328,#57329,#57330,#57331,#57332,#57333,#57334,#57335,#57336,#57337,
#57338,#57339,#57340,#57341,#57342,#57343,#57344,#57345,#57346,#57347,#57348,
#57349,#57350,#57351,#57352,#57353,#57354,#57355,#57356,#57357,#57358,#57359,
#57360,#57361,#57362,#57363,#57364,#57365,#57366,#57367,#57368,#57369,#57370,
#57371,#57372,#57373,#57374,#57375,#57376,#57377,#57378,#57379,#57380,#57381,
#57382,#57383,#57384,#57385,#57386,#57387,#57388,#57389,#57390,#57391,#57392,
#57393,#57394,#57395,#57396,#57397,#57398,#57399,#57400,#57401,#57402,#57403,
#57404,#57405,#57406,#57407,#57408,#57409,#57410,#57411,#57412,#57413,#57414,
#57415,#57416,#57417,#57418,#57419,#57420,#57421,#57422),(#57423,#57424,
#57425,#57426,#57427,#57428,#57429,#57430,#57431,#57432,#57433,#57434,#57435,
#57436,#57437,#57438,#57439,#57440,#57441,#57442,#57443,#57444,#57445,#57446,
#57447,#57448,#57449,#57450,#57451,#57452,#57453,#57454,#57455,#57456,#57457,
#57458,#57459,#57460,#57461,#57462,#57463,#57464,#57465,#57466,#57467,#57468,
#57469,#57470,#57471,#57472,#57473,#57474,#57475,#57476,#57477,#57478,#57479,
#57480,#57481,#57482,#57483,#57484,#57485,#57486,#57487,#57488,#57489,#57490,
#57491,#57492,#57493,#57494,#57495,#57496,#57497,#57498,#57499,#57500,#57501,
#57502,#57503,#57504,#57505,#57506,#57507,#57508,#57509,#57510,#57511,#57512,
#57513,#57514,#57515,#57516,#57517,#57518,#57519,#57520,#57521,#57522,#57523),
(#57524,#57525,#57526,#57527,#57528,#57529,#57530,#57531,#57532,#57533,
#57534,#57535,#57536,#57537,#57538,#57539,#57540,#57541,#57542,#57543,#57544,
#57545,#57546,#57547,#57548,#57549,#57550,#57551,#57552,#57553,#57554,#57555,
#57556,#57557,#57558,#57559,#57560,#57561,#57562,#57563,#57564,#57565,#57566,
#57567,#57568,#57569,#57570,#57571,#57572,#57573,#57574,#57575,#57576,#57577,
#57578,#57579,#57580,#57581,#57582,#57583,#57584,#57585,#57586,#57587,#57588,
#57589,#57590,#57591,#57592,#57593,#57594,#57595,#57596,#57597,#57598,#57599,
#57600,#57601,#57602,#57603,#57604,#57605,#57606,#57607,#57608,#57609,#57610,
#57611,#57612,#57613,#57614,#57615,#57616,#57617,#57618,#57619,#57620,#57621,
#57622,#57623,#57624),(#57625,#57626,#57627,#57628,#57629,#57630,#57631,
#57632,#57633,#57634,#57635,#57636,#57637,#57638,#57639,#57640,#57641,#57642,
#57643,#57644,#57645,#57646,#57647,#57648,#57649,#57650,#57651,#57652,#57653,
#57654,#57655,#57656,#57657,#57658,#57659,#57660,#57661,#57662,#57663,#57664,
#57665,#57666,#57667,#57668,#57669,#57670,#57671,#57672,#57673,#57674,#57675,
#57676,#57677,#57678,#57679,#57680,#57681,#57682,#57683,#57684,#57685,#57686,
#57687,#57688,#57689,#57690,#57691,#57692,#57693,#57694,#57695,#57696,#57697,
#57698,#57699,#57700,#57701,#57702,#57703,#57704,#57705,#57706,#57707,#57708,
#57709,#57710,#57711,#57712,#57713,#57714,#57715,#57716,#57717,#57718,#57719,
#57720,#57721,#57722,#57723,#57724,#57725),(#57726,#57727,#57728,#57729,
#57730,#57731,#57732,#57733,#57734,#57735,#57736,#57737,#57738,#57739,#57740,
#57741,#57742,#57743,#57744,#57745,#57746,#57747,#57748,#57749,#57750,#57751,
#57752,#57753,#57754,#57755,#57756,#57757,#57758,#57759,#57760,#57761,#57762,
#57763,#57764,#57765,#57766,#57767,#57768,#57769,#57770,#57771,#57772,#57773,
#57774,#57775,#57776,#57777,#57778,#57779,#57780,#57781,#57782,#57783,#57784,
#57785,#57786,#57787,#57788,#57789,#57790,#57791,#57792,#57793,#57794,#57795,
#57796,#57797,#57798,#57799,#57800,#57801,#57802,#57803,#57804,#57805,#57806,
#57807,#57808,#57809,#57810,#57811,#57812,#57813,#57814,#57815,#57816,#57817,
#57818,#57819,#57820,#57821,#57822,#57823,#57824,#57825,#57826)),
 .UNSPECIFIED.,.F.,.F.,.F.,(4,1,4),(4,1,1,1,1,1,1,1,1,1,1,1,1,1,1,1,1,1,
1,1,1,1,1,1,1,1,1,1,1,1,1,1,1,1,1,1,1,1,1,1,1,1,1,1,1,1,1,1,1,1,1,1,1,1,
1,1,1,1,1,1,1,1,1,1,1,1,1,1,1,1,1,1,1,1,1,1,1,1,1,1,1,1,1,1,1,1,1,1,1,1,
1,1,1,1,1,1,1,1,4),(-1.09083078249646,-0.623331875712262,0.),(9.57812533864917,
10.0685237204885,10.5589221023277,11.049320484167,11.5397188660063,12.0301172478456,
12.5205156296849,13.0109140115242,13.5013123933634,13.9917107752027,14.482109157042,
14.9725075388813,15.4629059207206,15.9533043025599,16.4437026843991,16.9341010662384,
17.4244994480777,17.914897829917,18.4052962117563,18.8956945935956,19.3860929754348,
19.8764913572741,20.3668897391134,20.8572881209527,21.347686502792,21.8380848846313,
22.3284832664706,22.8188816483098,23.3092800301491,23.7996784119884,24.2900767938277,
24.780475175667,25.2708735575063,25.7612719393455,26.2516703211848,26.7420687030241,
27.2324670848634,27.7228654667027,28.213263848542,28.7036622303812,29.1940606122205,
29.6844589940598,30.1748573758991,30.6652557577384,31.1556541395777,31.6460525214169,
32.1364509032562,32.6268492850955,33.1172476669348,33.6076460487741,34.0980444306134,
34.5884428124527,35.0788411942919,35.5692395761312,36.0596379579705,36.5500363398098,
37.0404347216491,37.5308331034883,38.0212314853276,38.5116298671669,39.0020282490062,
39.4924266308455,39.9828250126848,40.4732233945241,40.9636217763633,41.4540201582026,
41.9444185400419,42.4348169218812,42.9252153037205,43.4156136855598,43.906012067399,
44.3964104492383,44.8868088310776,45.3772072129169,45.8676055947562,46.3580039765955,
46.8484023584347,47.338800740274,47.8291991221133,48.3195975039526,48.8099958857919,
49.3003942676312,49.7907926494704,50.2811910313097,50.771589413149,51.2619877949883,
51.7523861768276,52.2427845586669,52.7331829405062,53.2235813223454,53.7139797041847,
54.204378086024,54.6947764678633,55.1851748497026,55.6755732315419,56.1659716133811,
56.6563699952204,57.1467683770597,57.637166758899),.UNSPECIFIED.);
#567=B_SPLINE_SURFACE_WITH_KNOTS('',3,3,((#57934,#57935,#57936,#57937,#57938,
#57939,#57940,#57941,#57942,#57943,#57944,#57945,#57946,#57947,#57948,#57949,
#57950,#57951,#57952,#57953,#57954,#57955,#57956,#57957,#57958,#57959,#57960,
#57961,#57962,#57963,#57964,#57965,#57966,#57967,#57968,#57969,#57970,#57971,
#57972,#57973,#57974,#57975,#57976,#57977,#57978,#57979,#57980,#57981,#57982,
#57983,#57984,#57985,#57986,#57987,#57988,#57989,#57990,#57991,#57992,#57993,
#57994,#57995,#57996,#57997,#57998,#57999,#58000,#58001,#58002,#58003,#58004,
#58005,#58006,#58007,#58008,#58009,#58010,#58011,#58012,#58013,#58014,#58015,
#58016,#58017,#58018,#58019,#58020,#58021,#58022,#58023,#58024,#58025,#58026,
#58027,#58028,#58029,#58030,#58031,#58032,#58033,#58034),(#58035,#58036,
#58037,#58038,#58039,#58040,#58041,#58042,#58043,#58044,#58045,#58046,#58047,
#58048,#58049,#58050,#58051,#58052,#58053,#58054,#58055,#58056,#58057,#58058,
#58059,#58060,#58061,#58062,#58063,#58064,#58065,#58066,#58067,#58068,#58069,
#58070,#58071,#58072,#58073,#58074,#58075,#58076,#58077,#58078,#58079,#58080,
#58081,#58082,#58083,#58084,#58085,#58086,#58087,#58088,#58089,#58090,#58091,
#58092,#58093,#58094,#58095,#58096,#58097,#58098,#58099,#58100,#58101,#58102,
#58103,#58104,#58105,#58106,#58107,#58108,#58109,#58110,#58111,#58112,#58113,
#58114,#58115,#58116,#58117,#58118,#58119,#58120,#58121,#58122,#58123,#58124,
#58125,#58126,#58127,#58128,#58129,#58130,#58131,#58132,#58133,#58134,#58135),
(#58136,#58137,#58138,#58139,#58140,#58141,#58142,#58143,#58144,#58145,
#58146,#58147,#58148,#58149,#58150,#58151,#58152,#58153,#58154,#58155,#58156,
#58157,#58158,#58159,#58160,#58161,#58162,#58163,#58164,#58165,#58166,#58167,
#58168,#58169,#58170,#58171,#58172,#58173,#58174,#58175,#58176,#58177,#58178,
#58179,#58180,#58181,#58182,#58183,#58184,#58185,#58186,#58187,#58188,#58189,
#58190,#58191,#58192,#58193,#58194,#58195,#58196,#58197,#58198,#58199,#58200,
#58201,#58202,#58203,#58204,#58205,#58206,#58207,#58208,#58209,#58210,#58211,
#58212,#58213,#58214,#58215,#58216,#58217,#58218,#58219,#58220,#58221,#58222,
#58223,#58224,#58225,#58226,#58227,#58228,#58229,#58230,#58231,#58232,#58233,
#58234,#58235,#58236),(#58237,#58238,#58239,#58240,#58241,#58242,#58243,
#58244,#58245,#58246,#58247,#58248,#58249,#58250,#58251,#58252,#58253,#58254,
#58255,#58256,#58257,#58258,#58259,#58260,#58261,#58262,#58263,#58264,#58265,
#58266,#58267,#58268,#58269,#58270,#58271,#58272,#58273,#58274,#58275,#58276,
#58277,#58278,#58279,#58280,#58281,#58282,#58283,#58284,#58285,#58286,#58287,
#58288,#58289,#58290,#58291,#58292,#58293,#58294,#58295,#58296,#58297,#58298,
#58299,#58300,#58301,#58302,#58303,#58304,#58305,#58306,#58307,#58308,#58309,
#58310,#58311,#58312,#58313,#58314,#58315,#58316,#58317,#58318,#58319,#58320,
#58321,#58322,#58323,#58324,#58325,#58326,#58327,#58328,#58329,#58330,#58331,
#58332,#58333,#58334,#58335,#58336,#58337)),.UNSPECIFIED.,.F.,.F.,.F.,(4,
4),(4,1,1,1,1,1,1,1,1,1,1,1,1,1,1,1,1,1,1,1,1,1,1,1,1,1,1,1,1,1,1,1,1,1,
1,1,1,1,1,1,1,1,1,1,1,1,1,1,1,1,1,1,1,1,1,1,1,1,1,1,1,1,1,1,1,1,1,1,1,1,
1,1,1,1,1,1,1,1,1,1,1,1,1,1,1,1,1,1,1,1,1,1,1,1,1,1,1,1,4),(0.,0.0671853436149873),
(10.3432104236078,10.8406801321902,11.3381498407727,11.8356195493552,12.3330892579377,
12.8305589665202,13.3280286751027,13.8254983836852,14.3229680922677,14.8204378008502,
15.3179075094327,15.8153772180151,16.3128469265976,16.8103166351801,17.3077863437626,
17.8052560523451,18.3027257609276,18.8001954695101,19.2976651780926,19.7951348866751,
20.2926045952576,20.79007430384,21.2875440124225,21.785013721005,22.2824834295875,
22.77995313817,23.2774228467525,23.774892555335,24.2723622639175,24.7698319725,
25.2673016810825,25.7647713896649,26.2622410982474,26.7597108068299,27.2571805154124,
27.7546502239949,28.2521199325774,28.7495896411599,29.2470593497424,29.7445290583249,
30.2419987669074,30.7394684754899,31.2369381840723,31.7344078926548,32.2318776012373,
32.7293473098198,33.2268170184023,33.7242867269848,34.2217564355673,34.7192261441498,
35.2166958527323,35.7141655613148,36.2116352698972,36.7091049784797,37.2065746870622,
37.7040443956447,38.2015141042272,38.6989838128097,39.1964535213922,39.6939232299747,
40.1913929385572,40.6888626471397,41.1863323557221,41.6838020643046,42.1812717728871,
42.6787414814696,43.1762111900521,43.6736808986346,44.1711506072171,44.6686203157996,
45.1660900243821,45.6635597329646,46.1610294415471,46.6584991501295,47.155968858712,
47.6534385672945,48.150908275877,48.6483779844595,49.145847693042,49.6433174016245,
50.140787110207,50.6382568187895,51.135726527372,51.6331962359544,52.1306659445369,
52.6281356531194,53.1256053617019,53.6230750702844,54.1205447788669,54.6180144874494,
55.1154841960319,55.6129539046144,56.1104236131969,56.6078933217793,57.1053630303618,
57.6028327389443,58.1003024475268,58.5977721561093,59.0952418646918),
 .UNSPECIFIED.);
#568=B_SPLINE_SURFACE_WITH_KNOTS('',3,3,((#58490,#58491,#58492,#58493,#58494,
#58495,#58496,#58497,#58498,#58499,#58500,#58501,#58502,#58503,#58504,#58505,
#58506,#58507,#58508,#58509,#58510,#58511,#58512,#58513,#58514,#58515,#58516,
#58517,#58518,#58519,#58520,#58521,#58522,#58523,#58524,#58525,#58526,#58527,
#58528,#58529,#58530,#58531,#58532,#58533,#58534,#58535,#58536,#58537,#58538,
#58539,#58540,#58541,#58542,#58543,#58544,#58545,#58546,#58547,#58548,#58549,
#58550,#58551,#58552,#58553,#58554,#58555,#58556,#58557,#58558,#58559,#58560,
#58561,#58562,#58563,#58564,#58565,#58566,#58567,#58568,#58569,#58570,#58571,
#58572,#58573,#58574,#58575,#58576,#58577,#58578,#58579,#58580,#58581,#58582,
#58583,#58584,#58585,#58586,#58587,#58588,#58589,#58590),(#58591,#58592,
#58593,#58594,#58595,#58596,#58597,#58598,#58599,#58600,#58601,#58602,#58603,
#58604,#58605,#58606,#58607,#58608,#58609,#58610,#58611,#58612,#58613,#58614,
#58615,#58616,#58617,#58618,#58619,#58620,#58621,#58622,#58623,#58624,#58625,
#58626,#58627,#58628,#58629,#58630,#58631,#58632,#58633,#58634,#58635,#58636,
#58637,#58638,#58639,#58640,#58641,#58642,#58643,#58644,#58645,#58646,#58647,
#58648,#58649,#58650,#58651,#58652,#58653,#58654,#58655,#58656,#58657,#58658,
#58659,#58660,#58661,#58662,#58663,#58664,#58665,#58666,#58667,#58668,#58669,
#58670,#58671,#58672,#58673,#58674,#58675,#58676,#58677,#58678,#58679,#58680,
#58681,#58682,#58683,#58684,#58685,#58686,#58687,#58688,#58689,#58690,#58691),
(#58692,#58693,#58694,#58695,#58696,#58697,#58698,#58699,#58700,#58701,
#58702,#58703,#58704,#58705,#58706,#58707,#58708,#58709,#58710,#58711,#58712,
#58713,#58714,#58715,#58716,#58717,#58718,#58719,#58720,#58721,#58722,#58723,
#58724,#58725,#58726,#58727,#58728,#58729,#58730,#58731,#58732,#58733,#58734,
#58735,#58736,#58737,#58738,#58739,#58740,#58741,#58742,#58743,#58744,#58745,
#58746,#58747,#58748,#58749,#58750,#58751,#58752,#58753,#58754,#58755,#58756,
#58757,#58758,#58759,#58760,#58761,#58762,#58763,#58764,#58765,#58766,#58767,
#58768,#58769,#58770,#58771,#58772,#58773,#58774,#58775,#58776,#58777,#58778,
#58779,#58780,#58781,#58782,#58783,#58784,#58785,#58786,#58787,#58788,#58789,
#58790,#58791,#58792),(#58793,#58794,#58795,#58796,#58797,#58798,#58799,
#58800,#58801,#58802,#58803,#58804,#58805,#58806,#58807,#58808,#58809,#58810,
#58811,#58812,#58813,#58814,#58815,#58816,#58817,#58818,#58819,#58820,#58821,
#58822,#58823,#58824,#58825,#58826,#58827,#58828,#58829,#58830,#58831,#58832,
#58833,#58834,#58835,#58836,#58837,#58838,#58839,#58840,#58841,#58842,#58843,
#58844,#58845,#58846,#58847,#58848,#58849,#58850,#58851,#58852,#58853,#58854,
#58855,#58856,#58857,#58858,#58859,#58860,#58861,#58862,#58863,#58864,#58865,
#58866,#58867,#58868,#58869,#58870,#58871,#58872,#58873,#58874,#58875,#58876,
#58877,#58878,#58879,#58880,#58881,#58882,#58883,#58884,#58885,#58886,#58887,
#58888,#58889,#58890,#58891,#58892,#58893),(#58894,#58895,#58896,#58897,
#58898,#58899,#58900,#58901,#58902,#58903,#58904,#58905,#58906,#58907,#58908,
#58909,#58910,#58911,#58912,#58913,#58914,#58915,#58916,#58917,#58918,#58919,
#58920,#58921,#58922,#58923,#58924,#58925,#58926,#58927,#58928,#58929,#58930,
#58931,#58932,#58933,#58934,#58935,#58936,#58937,#58938,#58939,#58940,#58941,
#58942,#58943,#58944,#58945,#58946,#58947,#58948,#58949,#58950,#58951,#58952,
#58953,#58954,#58955,#58956,#58957,#58958,#58959,#58960,#58961,#58962,#58963,
#58964,#58965,#58966,#58967,#58968,#58969,#58970,#58971,#58972,#58973,#58974,
#58975,#58976,#58977,#58978,#58979,#58980,#58981,#58982,#58983,#58984,#58985,
#58986,#58987,#58988,#58989,#58990,#58991,#58992,#58993,#58994)),
 .UNSPECIFIED.,.F.,.F.,.F.,(4,1,4),(4,1,1,1,1,1,1,1,1,1,1,1,1,1,1,1,1,1,
1,1,1,1,1,1,1,1,1,1,1,1,1,1,1,1,1,1,1,1,1,1,1,1,1,1,1,1,1,1,1,1,1,1,1,1,
1,1,1,1,1,1,1,1,1,1,1,1,1,1,1,1,1,1,1,1,1,1,1,1,1,1,1,1,1,1,1,1,1,1,1,1,
1,1,1,1,1,1,1,1,4),(-1.09083078249646,-0.623331875712262,0.),(11.8012855294006,
12.2916839112398,12.7820822930791,13.2724806749184,13.7628790567577,14.253277438597,
14.7436758204363,15.2340742022755,15.7244725841148,16.2148709659541,16.7052693477934,
17.1956677296327,17.686066111472,18.1764644933112,18.6668628751505,19.1572612569898,
19.6476596388291,20.1380580206684,20.6284564025077,21.118854784347,21.6092531661862,
22.0996515480255,22.5900499298648,23.0804483117041,23.5708466935434,24.0612450753827,
24.5516434572219,25.0420418390612,25.5324402209005,26.0228386027398,26.5132369845791,
27.0036353664184,27.4940337482576,27.9844321300969,28.4748305119362,28.9652288937755,
29.4556272756148,29.9460256574541,30.4364240392933,30.9268224211326,31.4172208029719,
31.9076191848112,32.3980175666505,32.8884159484898,33.378814330329,33.8692127121683,
34.3596110940076,34.8500094758469,35.3404078576862,35.8308062395255,36.3212046213647,
36.811603003204,37.3020013850433,37.7923997668826,38.2827981487219,38.7731965305612,
39.2635949124004,39.7539932942397,40.244391676079,40.7347900579183,41.2251884397576,
41.7155868215969,42.2059852034361,42.6963835852754,43.1867819671147,43.677180348954,
44.1675787307933,44.6579771126326,45.1483754944719,45.6387738763111,46.1291722581504,
46.6195706399897,47.109969021829,47.6003674036683,48.0907657855076,48.5811641673468,
49.0715625491861,49.5619609310254,50.0523593128647,50.542757694704,51.0331560765433,
51.5235544583825,52.0139528402218,52.5043512220611,52.9947496039004,53.4851479857397,
53.975546367579,54.4659447494182,54.9563431312575,55.4467415130968,55.9371398949361,
56.4275382767754,56.9179366586147,57.4083350404539,57.8987334222932,58.3891318041325,
58.8795301859718,59.3699285678111,59.8603269496504),.UNSPECIFIED.);
#1374=B_SPLINE_CURVE_WITH_KNOTS('',3,(#52488,#52489,#52490,#52491,#52492,
#52493,#52494,#52495,#52496,#52497,#52498),.UNSPECIFIED.,.F.,.F.,(4,1,1,
1,1,1,1,1,4),(53.4070751110265,53.7139797041847,54.204378086024,54.6947764678633,
55.1851748497026,55.6755732315419,56.1659716133811,56.6563699952204,56.8720816739404),
 .UNSPECIFIED.);
#1375=B_SPLINE_CURVE_WITH_KNOTS('',3,(#52501,#52502,#52503,#52504,#52505,
#52506,#52507,#52508,#52509,#52510),.UNSPECIFIED.,.F.,.F.,(4,1,1,1,1,1,
1,4),(53.4070751110265,53.622996627145,54.1133950089843,54.6037933908236,
55.0941917726629,55.5845901545022,56.0749885363415,56.5653869181807),
 .UNSPECIFIED.);
#1376=B_SPLINE_CURVE_WITH_KNOTS('',3,(#52515,#52516,#52517,#52518,#52519,
#52520,#52521,#52522,#52523,#52524,#52525,#52526,#52527,#52528,#52529,#52530,
#52531),.UNSPECIFIED.,.F.,.F.,(4,1,1,1,1,1,1,1,1,1,1,1,1,1,4),(47.1238898038469,
47.338800740274,47.8291991221133,48.3195975039526,48.8099958857919,49.3003942676312,
49.7907926494704,50.2811910313097,50.771589413149,51.2619877949883,51.7523861768276,
52.2427845586669,52.7331829405062,53.2235813223454,53.4070751110265),
 .UNSPECIFIED.);
#1377=B_SPLINE_CURVE_WITH_KNOTS('',3,(#52532,#52533,#52534,#52535,#52536,
#52537,#52538,#52539,#52540,#52541,#52542,#52543,#52544,#52545,#52546,#52547,
#52548),.UNSPECIFIED.,.F.,.F.,(4,1,1,1,1,1,1,1,1,1,1,1,1,1,4),(47.1238898038469,
47.2478176632343,47.7382160450736,48.2286144269129,48.7190128087522,49.2094111905915,
49.6998095724308,50.1902079542701,50.6806063361093,51.1710047179486,51.6614030997879,
52.1518014816272,52.6421998634665,53.1325982453058,53.4070751110265),
 .UNSPECIFIED.);
#1378=B_SPLINE_CURVE_WITH_KNOTS('',3,(#52553,#52554,#52555,#52556,#52557,
#52558,#52559,#52560,#52561,#52562,#52563,#52564,#52565,#52566,#52567,#52568,
#52569),.UNSPECIFIED.,.F.,.F.,(4,1,1,1,1,1,1,1,1,1,1,1,1,1,4),(40.8407044966673,
40.9636217763633,41.4540201582026,41.9444185400419,42.4348169218812,42.9252153037205,
43.4156136855598,43.906012067399,44.3964104492383,44.8868088310776,45.3772072129169,
45.8676055947562,46.3580039765955,46.8484023584347,47.1238898038469),
 .UNSPECIFIED.);
#1379=B_SPLINE_CURVE_WITH_KNOTS('',3,(#52570,#52571,#52572,#52573,#52574,
#52575,#52576,#52577,#52578,#52579,#52580,#52581,#52582,#52583,#52584,#52585,
#52586),.UNSPECIFIED.,.F.,.F.,(4,1,1,1,1,1,1,1,1,1,1,1,1,1,4),(40.8407044966673,
40.8726386993237,41.3630370811629,41.8534354630022,42.3438338448415,42.8342322266808,
43.3246306085201,43.8150289903594,44.3054273721986,44.7958257540379,45.2862241358772,
45.7766225177165,46.2670208995558,46.7574192813951,47.1238898038469),
 .UNSPECIFIED.);
#1380=B_SPLINE_CURVE_WITH_KNOTS('',3,(#52591,#52592,#52593,#52594,#52595,
#52596,#52597,#52598,#52599,#52600,#52601,#52602,#52603,#52604,#52605,#52606,
#52607),.UNSPECIFIED.,.F.,.F.,(4,1,1,1,1,1,1,1,1,1,1,1,1,1,4),(34.5575191894877,
34.5884428124527,35.0788411942919,35.5692395761312,36.0596379579705,36.5500363398098,
37.0404347216491,37.5308331034883,38.0212314853276,38.5116298671669,39.0020282490062,
39.4924266308455,39.9828250126848,40.4732233945241,40.8407044966673),
 .UNSPECIFIED.);
#1381=B_SPLINE_CURVE_WITH_KNOTS('',3,(#52608,#52609,#52610,#52611,#52612,
#52613,#52614,#52615,#52616,#52617,#52618,#52619,#52620,#52621,#52622,#52623),
 .UNSPECIFIED.,.F.,.F.,(4,1,1,1,1,1,1,1,1,1,1,1,1,4),(34.5575191894877,
34.9878581172523,35.4782564990915,35.9686548809308,36.4590532627701,36.9494516446094,
37.4398500264487,37.930248408288,38.4206467901272,38.9110451719665,39.4014435538058,
39.8918419356451,40.3822403174844,40.8407044966673),.UNSPECIFIED.);
#1382=B_SPLINE_CURVE_WITH_KNOTS('',3,(#52628,#52629,#52630,#52631,#52632,
#52633,#52634,#52635,#52636,#52637,#52638,#52639,#52640,#52641,#52642,#52643),
 .UNSPECIFIED.,.F.,.F.,(4,1,1,1,1,1,1,1,1,1,1,1,1,4),(28.2743338823081,
28.7036622303812,29.1940606122205,29.6844589940598,30.1748573758991,30.6652557577384,
31.1556541395777,31.6460525214169,32.1364509032562,32.6268492850955,33.1172476669348,
33.6076460487741,34.0980444306134,34.5575191894877),.UNSPECIFIED.);
#1383=B_SPLINE_CURVE_WITH_KNOTS('',3,(#52644,#52645,#52646,#52647,#52648,
#52649,#52650,#52651,#52652,#52653,#52654,#52655,#52656,#52657,#52658,#52659,
#52660),.UNSPECIFIED.,.F.,.F.,(4,1,1,1,1,1,1,1,1,1,1,1,1,1,4),(28.2743338823081,
28.6126791533416,29.1030775351808,29.5934759170201,30.0838742988594,30.5742726806987,
31.064671062538,31.5550694443773,32.0454678262166,32.5358662080558,33.0262645898951,
33.5166629717344,34.0070613535737,34.497459735413,34.5575191894877),
 .UNSPECIFIED.);
#1384=B_SPLINE_CURVE_WITH_KNOTS('',3,(#52665,#52666,#52667,#52668,#52669,
#52670,#52671,#52672,#52673,#52674,#52675,#52676,#52677,#52678,#52679,#52680,
#52681),.UNSPECIFIED.,.F.,.F.,(4,1,1,1,1,1,1,1,1,1,1,1,1,1,4),(21.9911485751285,
22.3284832664706,22.8188816483098,23.3092800301491,23.7996784119884,24.2900767938277,
24.780475175667,25.2708735575063,25.7612719393455,26.2516703211848,26.7420687030241,
27.2324670848634,27.7228654667027,28.213263848542,28.2743338823081),
 .UNSPECIFIED.);
#1385=B_SPLINE_CURVE_WITH_KNOTS('',3,(#52682,#52683,#52684,#52685,#52686,
#52687,#52688,#52689,#52690,#52691,#52692,#52693,#52694,#52695,#52696,#52697,
#52698),.UNSPECIFIED.,.F.,.F.,(4,1,1,1,1,1,1,1,1,1,1,1,1,1,4),(21.9911485751285,
22.2375001894309,22.7278985712702,23.2182969531094,23.7086953349487,24.199093716788,
24.6894920986273,25.1798904804666,25.6702888623059,26.1606872441451,26.6510856259844,
27.1414840078237,27.631882389663,28.1222807715023,28.2743338823081),
 .UNSPECIFIED.);
#1386=B_SPLINE_CURVE_WITH_KNOTS('',3,(#52703,#52704,#52705,#52706,#52707,
#52708,#52709,#52710,#52711,#52712,#52713,#52714,#52715,#52716,#52717,#52718,
#52719),.UNSPECIFIED.,.F.,.F.,(4,1,1,1,1,1,1,1,1,1,1,1,1,1,4),(15.7079632679489,
15.9533043025599,16.4437026843991,16.9341010662384,17.4244994480777,17.914897829917,
18.4052962117563,18.8956945935956,19.3860929754348,19.8764913572741,20.3668897391134,
20.8572881209527,21.347686502792,21.8380848846313,21.9911485751285),
 .UNSPECIFIED.);
#1387=B_SPLINE_CURVE_WITH_KNOTS('',3,(#52720,#52721,#52722,#52723,#52724,
#52725,#52726,#52727,#52728,#52729,#52730,#52731,#52732,#52733,#52734,#52735,
#52736),.UNSPECIFIED.,.F.,.F.,(4,1,1,1,1,1,1,1,1,1,1,1,1,1,4),(15.7079632679489,
15.8623212255202,16.3527196073595,16.8431179891988,17.333516371038,17.8239147528773,
18.3143131347166,18.8047115165559,19.2951098983952,19.7855082802345,20.2759066620737,
20.766305043913,21.2567034257523,21.7471018075916,21.9911485751285),
 .UNSPECIFIED.);
#1388=B_SPLINE_CURVE_WITH_KNOTS('',3,(#52743,#52744,#52745,#52746,#52747,
#52748,#52749,#52750,#52751,#52752,#52753,#52754,#52755,#52756,#52757,#52758),
 .UNSPECIFIED.,.F.,.F.,(4,1,1,1,1,1,1,1,1,1,1,1,1,4),(9.57812533864917,
10.0685237204885,10.5589221023277,11.049320484167,11.5397188660063,12.0301172478456,
12.5205156296849,13.0109140115242,13.5013123933634,13.9917107752027,14.482109157042,
14.9725075388813,15.4629059207206,15.7079632679489),.UNSPECIFIED.);
#1389=B_SPLINE_CURVE_WITH_KNOTS('',3,(#52759,#52760,#52761,#52762,#52763,
#52764,#52765,#52766,#52767,#52768,#52769,#52770,#52771,#52772,#52773,#52774,
#52775),.UNSPECIFIED.,.F.,.F.,(4,1,1,1,1,1,1,1,1,1,1,1,1,1,4),(9.42477796076936,
9.4871422616095,9.97754064344878,10.4679390252881,10.9583374071273,11.4487357889666,
11.9391341708059,12.4295325526452,12.9199309344845,13.4103293163238,13.9007276981631,
14.3911260800023,14.8815244618416,15.3719228436809,15.7079632679489),
 .UNSPECIFIED.);
#1390=B_SPLINE_CURVE_WITH_KNOTS('',3,(#52781,#52782,#52783,#52784,#52785,
#52786,#52787,#52788,#52789,#52790,#52791,#52792,#52793,#52794,#52795,#52796),
 .UNSPECIFIED.,.F.,.F.,(4,3,3,3,3,4),(-4.09323272002469,-3.96713944972556,
-3.47124701850987,-2.97535458729417,-2.47946215607848,-2.07135887395548),
 .UNSPECIFIED.);
#1391=B_SPLINE_CURVE_WITH_KNOTS('',3,(#52799,#52800,#52801,#52802,#52803,
#52804,#52805,#52806,#52807,#52808),.UNSPECIFIED.,.F.,.F.,(4,3,3,4),(0.,
0.495892431215694,0.991784862431392,1.11971880752058),.UNSPECIFIED.);
#1392=B_SPLINE_CURVE_WITH_KNOTS('',3,(#52813,#52814,#52815,#52816,#52817,
#52818,#52819,#52820,#52821,#52822,#52823,#52824,#52825,#52826,#52827,#52828,
#52829,#52830,#52831,#52832,#52833,#52834,#52835,#52836,#52837,#52838,#52839,
#52840,#52841,#52842,#52843,#52844,#52845,#52846,#52847,#52848,#52849,#52850,
#52851,#52852),.UNSPECIFIED.,.F.,.F.,(4,3,3,3,3,3,3,3,3,3,3,3,3,4),(-10.3764180272043,
-9.91784862431391,-9.42195619309822,-8.92606376188252,-8.43017133066683,
-7.93427889945113,-7.43838646823544,-6.94249403701974,-6.44660160580404,
-5.95070917458835,-5.45481674337265,-4.95892431215696,-4.46303188094126,
-4.09323272002469),.UNSPECIFIED.);
#1393=B_SPLINE_CURVE_WITH_KNOTS('',3,(#52853,#52854,#52855,#52856,#52857,
#52858,#52859,#52860,#52861,#52862,#52863,#52864,#52865,#52866,#52867,#52868,
#52869,#52870,#52871,#52872,#52873,#52874,#52875,#52876,#52877,#52878,#52879,
#52880,#52881,#52882,#52883,#52884,#52885,#52886,#52887,#52888,#52889,#52890,
#52891,#52892),.UNSPECIFIED.,.F.,.F.,(4,3,3,3,3,3,3,3,3,3,3,3,3,4),(1.11971880752058,
1.48767729364709,1.98356972486278,2.47946215607848,2.97535458729418,3.47124701850987,
3.96713944972557,4.46303188094126,4.95892431215696,5.45481674337265,5.95070917458835,
6.44660160580405,6.94249403701974,7.40290411470016),.UNSPECIFIED.);
#1394=B_SPLINE_CURVE_WITH_KNOTS('',3,(#52897,#52898,#52899,#52900,#52901,
#52902,#52903,#52904,#52905,#52906,#52907,#52908,#52909,#52910,#52911,#52912,
#52913,#52914,#52915,#52916,#52917,#52918,#52919,#52920,#52921,#52922,#52923,
#52924,#52925,#52926,#52927,#52928,#52929,#52930,#52931,#52932,#52933,#52934,
#52935,#52936,#52937,#52938,#52939),.UNSPECIFIED.,.F.,.F.,(4,3,3,3,3,3,
3,3,3,3,3,3,3,3,4),(-16.6596033343839,-16.364450230118,-15.8685577989023,
-15.3726653676866,-14.8767729364709,-14.3808805052552,-13.8849880740395,
-13.3890956428238,-12.8932032116081,-12.3973107803924,-11.9014183491767,
-11.405525917961,-10.9096334867453,-10.4137410555296,-10.3764180272043),
 .UNSPECIFIED.);
#1395=B_SPLINE_CURVE_WITH_KNOTS('',3,(#52940,#52941,#52942,#52943,#52944,
#52945,#52946,#52947,#52948,#52949,#52950,#52951,#52952,#52953,#52954,#52955,
#52956,#52957,#52958,#52959,#52960,#52961,#52962,#52963,#52964,#52965,#52966,
#52967,#52968,#52969,#52970,#52971,#52972,#52973,#52974,#52975,#52976,#52977,
#52978,#52979,#52980,#52981,#52982),.UNSPECIFIED.,.F.,.F.,(4,3,3,3,3,3,
3,3,3,3,3,3,3,3,4),(7.40290411470016,7.43838646823544,7.93427889945113,
8.43017133066683,8.92606376188253,9.42195619309822,9.91784862431392,10.4137410555296,
10.9096334867453,11.405525917961,11.9014183491767,12.3973107803924,12.8932032116081,
13.3890956428238,13.6860894218797),.UNSPECIFIED.);
#1396=B_SPLINE_CURVE_WITH_KNOTS('',3,(#52987,#52988,#52989,#52990,#52991,
#52992,#52993,#52994,#52995,#52996,#52997,#52998,#52999,#53000,#53001,#53002,
#53003,#53004,#53005,#53006,#53007,#53008,#53009,#53010,#53011,#53012,#53013,
#53014,#53015,#53016,#53017,#53018,#53019,#53020,#53021,#53022,#53023,#53024,
#53025,#53026,#53027,#53028,#53029),.UNSPECIFIED.,.F.,.F.,(4,3,3,3,3,3,
3,3,3,3,3,3,3,3,4),(-22.9427886415634,-22.811051835922,-22.3151594047063,
-21.8192669734906,-21.3233745422749,-20.8274821110592,-20.3315896798435,
-19.8356972486278,-19.3398048174121,-18.8439123861964,-18.3480199549807,
-17.852127523765,-17.3562350925493,-16.8603426613336,-16.6596033343839),
 .UNSPECIFIED.);
#1397=B_SPLINE_CURVE_WITH_KNOTS('',3,(#53030,#53031,#53032,#53033,#53034,
#53035,#53036,#53037,#53038,#53039,#53040,#53041,#53042,#53043,#53044,#53045,
#53046,#53047,#53048,#53049,#53050,#53051,#53052,#53053,#53054,#53055,#53056,
#53057,#53058,#53059,#53060,#53061,#53062,#53063,#53064,#53065,#53066,#53067,
#53068,#53069,#53070,#53071,#53072),.UNSPECIFIED.,.F.,.F.,(4,3,3,3,3,3,
3,3,3,3,3,3,3,3,4),(13.6860894218797,13.8849880740395,14.3808805052552,
14.8767729364709,15.3726653676866,15.8685577989023,16.364450230118,16.8603426613337,
17.3562350925494,17.8521275237651,18.3480199549808,18.8439123861965,19.3398048174122,
19.8356972486278,19.9692747290593),.UNSPECIFIED.);
#1398=B_SPLINE_CURVE_WITH_KNOTS('',3,(#53077,#53078,#53079,#53080,#53081,
#53082,#53083,#53084,#53085,#53086,#53087,#53088,#53089,#53090,#53091,#53092,
#53093,#53094,#53095,#53096,#53097,#53098,#53099,#53100,#53101,#53102,#53103,
#53104,#53105,#53106,#53107,#53108,#53109,#53110,#53111,#53112,#53113,#53114,
#53115,#53116),.UNSPECIFIED.,.F.,.F.,(4,3,3,3,3,3,3,3,3,3,3,3,3,4),(-29.225973948743,
-28.7617610105103,-28.2658685792946,-27.7699761480789,-27.2740837168633,
-26.7781912856476,-26.2822988544319,-25.7864064232162,-25.2905139920005,
-24.7946215607848,-24.2987291295691,-23.8028366983534,-23.3069442671377,
-22.9427886415634),.UNSPECIFIED.);
#1399=B_SPLINE_CURVE_WITH_KNOTS('',3,(#53117,#53118,#53119,#53120,#53121,
#53122,#53123,#53124,#53125,#53126,#53127,#53128,#53129,#53130,#53131,#53132,
#53133,#53134,#53135,#53136,#53137,#53138,#53139,#53140,#53141,#53142,#53143,
#53144,#53145,#53146,#53147,#53148,#53149,#53150,#53151,#53152,#53153,#53154,
#53155,#53156),.UNSPECIFIED.,.F.,.F.,(4,3,3,3,3,3,3,3,3,3,3,3,3,4),(19.9692747290593,
20.3315896798435,20.8274821110592,21.3233745422749,21.8192669734906,22.3151594047063,
22.811051835922,23.3069442671377,23.8028366983534,24.2987291295691,24.7946215607848,
25.2905139920005,25.7864064232162,26.2524600362389),.UNSPECIFIED.);
#1400=B_SPLINE_CURVE_WITH_KNOTS('',3,(#53161,#53162,#53163,#53164,#53165,
#53166,#53167,#53168,#53169,#53170,#53171,#53172,#53173,#53174,#53175,#53176,
#53177,#53178,#53179,#53180,#53181,#53182,#53183,#53184,#53185,#53186,#53187,
#53188,#53189,#53190,#53191,#53192,#53193,#53194,#53195,#53196,#53197,#53198,
#53199,#53200,#53201,#53202,#53203),.UNSPECIFIED.,.F.,.F.,(4,3,3,3,3,3,
3,3,3,3,3,3,3,3,4),(-35.5091592559226,-35.2083626163144,-34.7124701850987,
-34.216577753883,-33.7206853226673,-33.2247928914516,-32.7289004602359,
-32.2330080290202,-31.7371155978045,-31.2412231665888,-30.7453307353731,
-30.2494383041574,-29.7535458729417,-29.2576534417261,-29.225973948743),
 .UNSPECIFIED.);
#1401=B_SPLINE_CURVE_WITH_KNOTS('',3,(#53204,#53205,#53206,#53207,#53208,
#53209,#53210,#53211,#53212,#53213,#53214,#53215,#53216,#53217,#53218,#53219,
#53220,#53221,#53222,#53223,#53224,#53225,#53226,#53227,#53228,#53229,#53230,
#53231,#53232,#53233,#53234,#53235,#53236,#53237,#53238,#53239,#53240,#53241,
#53242,#53243,#53244,#53245,#53246),.UNSPECIFIED.,.F.,.F.,(4,3,3,3,3,3,
3,3,3,3,3,3,3,3,4),(26.2524600362389,26.2822988544319,26.7781912856476,
27.2740837168633,27.769976148079,28.2658685792947,28.7617610105104,29.2576534417261,
29.7535458729418,30.2494383041575,30.7453307353731,31.2412231665888,31.7371155978045,
32.2330080290202,32.5356453434185),.UNSPECIFIED.);
#1402=B_SPLINE_CURVE_WITH_KNOTS('',3,(#53251,#53252,#53253,#53254,#53255,
#53256,#53257,#53258,#53259,#53260,#53261,#53262,#53263,#53264,#53265,#53266,
#53267,#53268,#53269,#53270,#53271,#53272,#53273,#53274,#53275,#53276,#53277,
#53278,#53279,#53280,#53281,#53282,#53283,#53284,#53285,#53286,#53287,#53288,
#53289,#53290,#53291,#53292,#53293),.UNSPECIFIED.,.F.,.F.,(4,3,3,3,3,3,
3,3,3,3,3,3,3,3,4),(-41.7923445631022,-41.6549642221184,-41.1590717909027,
-40.663179359687,-40.1672869284713,-39.6713944972556,-39.1755020660399,
-38.6796096348243,-38.1837172036086,-37.6878247723929,-37.1919323411772,
-36.6960399099615,-36.2001474787458,-35.7042550475301,-35.5091592559226),
 .UNSPECIFIED.);
#1403=B_SPLINE_CURVE_WITH_KNOTS('',3,(#53294,#53295,#53296,#53297,#53298,
#53299,#53300,#53301,#53302,#53303,#53304,#53305,#53306,#53307,#53308,#53309,
#53310,#53311,#53312,#53313,#53314,#53315,#53316,#53317,#53318,#53319,#53320,
#53321,#53322,#53323,#53324,#53325,#53326,#53327,#53328,#53329,#53330,#53331,
#53332,#53333,#53334,#53335,#53336),.UNSPECIFIED.,.F.,.F.,(4,3,3,3,3,3,
3,3,3,3,3,3,3,3,4),(32.5356453434185,32.7289004602359,33.2247928914516,
33.7206853226673,34.216577753883,34.7124701850987,35.2083626163144,35.7042550475301,
36.2001474787458,36.6960399099615,37.1919323411772,37.6878247723929,38.1837172036086,
38.6796096348243,38.8188306505981),.UNSPECIFIED.);
#1404=B_SPLINE_CURVE_WITH_KNOTS('',3,(#53341,#53342,#53343,#53344,#53345,
#53346,#53347,#53348,#53349,#53350,#53351,#53352,#53353,#53354,#53355,#53356,
#53357,#53358,#53359,#53360,#53361,#53362,#53363,#53364,#53365,#53366,#53367,
#53368,#53369,#53370,#53371,#53372,#53373,#53374,#53375,#53376,#53377,#53378,
#53379,#53380),.UNSPECIFIED.,.F.,.F.,(4,3,3,3,3,3,3,3,3,3,3,3,3,4),(-48.0755298702818,
-47.6056733967068,-47.1097809654911,-46.6138885342754,-46.1179961030597,
-45.622103671844,-45.1262112406283,-44.6303188094126,-44.1344263781969,
-43.6385339469812,-43.1426415157655,-42.6467490845498,-42.1508566533341,
-41.7923445631022),.UNSPECIFIED.);
#1405=B_SPLINE_CURVE_WITH_KNOTS('',3,(#53381,#53382,#53383,#53384,#53385,
#53386,#53387,#53388,#53389,#53390,#53391,#53392,#53393,#53394,#53395,#53396,
#53397,#53398,#53399,#53400,#53401,#53402,#53403,#53404,#53405,#53406,#53407,
#53408,#53409,#53410,#53411,#53412,#53413,#53414,#53415,#53416,#53417,#53418,
#53419,#53420),.UNSPECIFIED.,.F.,.F.,(4,3,3,3,3,3,3,3,3,3,3,3,3,4),(38.8188306505981,
39.17550206604,39.6713944972557,40.1672869284714,40.6631793596871,41.1590717909028,
41.6549642221185,42.1508566533342,42.6467490845498,43.1426415157655,43.6385339469812,
44.1344263781969,44.6303188094126,45.1020159577777),.UNSPECIFIED.);
#1406=B_SPLINE_CURVE_WITH_KNOTS('',3,(#53425,#53426,#53427,#53428,#53429,
#53430,#53431,#53432,#53433,#53434,#53435,#53436,#53437,#53438,#53439,#53440,
#53441,#53442,#53443,#53444,#53445,#53446,#53447,#53448,#53449,#53450,#53451,
#53452,#53453,#53454,#53455,#53456,#53457,#53458,#53459,#53460,#53461,#53462,
#53463,#53464,#53465,#53466,#53467),.UNSPECIFIED.,.F.,.F.,(4,3,3,3,3,3,
3,3,3,3,3,3,3,3,4),(-54.3587151774614,-54.0522750025108,-53.5563825712951,
-53.0604901400794,-52.5645977088637,-52.068705277648,-51.5728128464323,
-51.0769204152166,-50.5810279840009,-50.0851355527853,-49.5892431215696,
-49.0933506903539,-48.5974582591382,-48.1015658279225,-48.0755298702818),
 .UNSPECIFIED.);
#1407=B_SPLINE_CURVE_WITH_KNOTS('',3,(#53468,#53469,#53470,#53471,#53472,
#53473,#53474,#53475,#53476,#53477,#53478,#53479,#53480,#53481,#53482,#53483,
#53484,#53485,#53486,#53487,#53488,#53489,#53490,#53491,#53492,#53493,#53494,
#53495,#53496,#53497,#53498,#53499,#53500,#53501,#53502,#53503,#53504,#53505,
#53506,#53507,#53508,#53509,#53510),.UNSPECIFIED.,.F.,.F.,(4,3,3,3,3,3,
3,3,3,3,3,3,3,3,4),(45.1020159577777,45.1262112406283,45.622103671844,46.1179961030597,
46.6138885342754,47.1097809654911,47.6056733967068,48.1015658279225,48.5974582591382,
49.0933506903539,49.5892431215696,50.0851355527853,50.581027984001,51.0769204152167,
51.3852012649573),.UNSPECIFIED.);
#1408=B_SPLINE_CURVE_WITH_KNOTS('',3,(#53516,#53517,#53518,#53519,#53520,
#53521,#53522,#53523),.UNSPECIFIED.,.F.,.F.,(4,1,1,1,1,4),(65.9734457253856,
66.1628979816508,66.6587904128665,67.1546828440821,67.6505752752978,68.0586785574208),
 .UNSPECIFIED.);
#1409=B_SPLINE_CURVE_WITH_KNOTS('',3,(#53526,#53527,#53528,#53529,#53530),
 .UNSPECIFIED.,.F.,.F.,(4,1,4),(65.9734457253857,66.3244736054852,66.8203660367009),
 .UNSPECIFIED.);
#1410=B_SPLINE_CURVE_WITH_KNOTS('',3,(#53535,#53536,#53537,#53538,#53539,
#53540,#53541,#53542,#53543,#53544,#53545,#53546,#53547,#53548,#53549,#53550,
#53551),.UNSPECIFIED.,.F.,.F.,(4,1,1,1,1,1,1,1,1,1,1,1,1,1,4),(59.6902604182061,
59.7162963758467,60.2121888070624,60.7080812382781,61.2039736694938,61.6998661007095,
62.1957585319252,62.6916509631409,63.1875433943566,63.6834358255723,64.179328256788,
64.6752206880037,65.1711131192194,65.6670055504351,65.9734457253856),
 .UNSPECIFIED.);
#1411=B_SPLINE_CURVE_WITH_KNOTS('',3,(#53552,#53553,#53554,#53555,#53556,
#53557,#53558,#53559,#53560,#53561,#53562,#53563,#53564,#53565,#53566,#53567,
#53568),.UNSPECIFIED.,.F.,.F.,(4,1,1,1,1,1,1,1,1,1,1,1,1,1,4),(59.6902604182061,
59.8778719996811,60.3737644308968,60.8696568621125,61.3655492933282,61.8614417245439,
62.3573341557596,62.8532265869753,63.349119018191,63.8450114494067,64.3409038806224,
64.8367963118381,65.3326887430538,65.8285811742695,65.9734457253857),
 .UNSPECIFIED.);
#1412=B_SPLINE_CURVE_WITH_KNOTS('',3,(#53573,#53574,#53575,#53576,#53577,
#53578,#53579,#53580,#53581,#53582,#53583,#53584,#53585,#53586,#53587,#53588),
 .UNSPECIFIED.,.F.,.F.,(4,1,1,1,1,1,1,1,1,1,1,1,1,4),(53.4070751110265,
53.7655872012584,54.2614796324741,54.7573720636898,55.2532644949055,55.7491569261211,
56.2450493573368,56.7409417885525,57.2368342197682,57.7327266509839,58.2286190821996,
58.7245115134153,59.220403944631,59.6902604182061),.UNSPECIFIED.);
#1413=B_SPLINE_CURVE_WITH_KNOTS('',3,(#53589,#53590,#53591,#53592,#53593,
#53594,#53595,#53596,#53597,#53598,#53599,#53600,#53601,#53602,#53603,#53604,
#53605),.UNSPECIFIED.,.F.,.F.,(4,1,1,1,1,1,1,1,1,1,1,1,1,1,4),(53.4070751110265,
53.4312703938771,53.9271628250928,54.4230552563085,54.9189476875242,55.4148401187399,
55.9107325499556,56.4066249811712,56.9025174123869,57.3984098436026,57.8943022748183,
58.390194706034,58.8860871372497,59.3819795684654,59.6902604182061),
 .UNSPECIFIED.);
#1414=B_SPLINE_CURVE_WITH_KNOTS('',3,(#53610,#53611,#53612,#53613,#53614,
#53615,#53616,#53617,#53618,#53619,#53620,#53621,#53622,#53623,#53624,#53625,
#53626),.UNSPECIFIED.,.F.,.F.,(4,1,1,1,1,1,1,1,1,1,1,1,1,1,4),(47.1238898038469,
47.3189855954543,47.81487802667,48.3107704578857,48.8066628891014,49.3025553203171,
49.7984477515328,50.2943401827485,50.7902326139642,51.2861250451799,51.7820174763956,
52.2779099076113,52.773802338827,53.2696947700427,53.4070751110265),
 .UNSPECIFIED.);
#1415=B_SPLINE_CURVE_WITH_KNOTS('',3,(#53627,#53628,#53629,#53630,#53631,
#53632,#53633,#53634,#53635,#53636,#53637,#53638,#53639,#53640,#53641,#53642),
 .UNSPECIFIED.,.F.,.F.,(4,1,1,1,1,1,1,1,1,1,1,1,1,4),(47.1238898038469,
47.4805612192887,47.9764536505044,48.4723460817201,48.9682385129358,49.4641309441515,
49.9600233753672,50.4559158065829,50.9518082377986,51.4477006690143,51.94359310023,
52.4394855314457,52.9353779626614,53.4070751110265),.UNSPECIFIED.);
#1416=B_SPLINE_CURVE_WITH_KNOTS('',3,(#53647,#53648,#53649,#53650,#53651,
#53652,#53653,#53654,#53655,#53656,#53657,#53658,#53659,#53660,#53661,#53662,
#53663),.UNSPECIFIED.,.F.,.F.,(4,1,1,1,1,1,1,1,1,1,1,1,1,1,4),(40.8407044966673,
40.8723839896503,41.368276420866,41.8641688520817,42.3600612832974,42.8559537145131,
43.3518461457288,43.8477385769445,44.3436310081602,44.8395234393758,45.3354158705915,
45.8313083018072,46.3272007330229,46.8230931642386,47.1238898038469),
 .UNSPECIFIED.);
#1417=B_SPLINE_CURVE_WITH_KNOTS('',3,(#53664,#53665,#53666,#53667,#53668,
#53669,#53670,#53671,#53672,#53673,#53674,#53675,#53676,#53677,#53678,#53679,
#53680),.UNSPECIFIED.,.F.,.F.,(4,1,1,1,1,1,1,1,1,1,1,1,1,1,4),(40.8407044966673,
41.0339596134847,41.5298520447004,42.0257444759161,42.5216369071318,43.0175293383475,
43.5134217695632,44.0093142007789,44.5052066319946,45.0010990632102,45.4969914944259,
45.9928839256416,46.4887763568573,46.984668788073,47.1238898038469),
 .UNSPECIFIED.);
#1418=B_SPLINE_CURVE_WITH_KNOTS('',3,(#53685,#53686,#53687,#53688,#53689,
#53690,#53691,#53692,#53693,#53694,#53695,#53696,#53697,#53698,#53699,#53700),
 .UNSPECIFIED.,.F.,.F.,(4,1,1,1,1,1,1,1,1,1,1,1,1,4),(34.5575191894877,
34.9216748150619,35.4175672462776,35.9134596774933,36.409352108709,36.9052445399247,
37.4011369711404,37.8970294023561,38.3929218335718,38.8888142647875,39.3847066960032,
39.8805991272189,40.3764915584346,40.8407044966673),.UNSPECIFIED.);
#1419=B_SPLINE_CURVE_WITH_KNOTS('',3,(#53701,#53702,#53703,#53704,#53705,
#53706,#53707,#53708,#53709,#53710,#53711,#53712,#53713,#53714,#53715,#53716,
#53717),.UNSPECIFIED.,.F.,.F.,(4,1,1,1,1,1,1,1,1,1,1,1,1,1,4),(34.5575191894877,
34.5873580076806,35.0832504388963,35.579142870112,36.0750353013277,36.5709277325434,
37.0668201637591,37.5627125949748,38.0586050261905,38.5544974574062,39.0503898886219,
39.5462823198376,40.0421747510533,40.538067182269,40.8407044966673),
 .UNSPECIFIED.);
#1420=B_SPLINE_CURVE_WITH_KNOTS('',3,(#53722,#53723,#53724,#53725,#53726,
#53727,#53728,#53729,#53730,#53731,#53732,#53733,#53734,#53735,#53736,#53737,
#53738),.UNSPECIFIED.,.F.,.F.,(4,1,1,1,1,1,1,1,1,1,1,1,1,1,4),(28.2743338823081,
28.4750732092579,28.9709656404736,29.4668580716893,29.962750502905,30.4586429341207,
30.9545353653364,31.4504277965521,31.9463202277678,32.4422126589835,32.9381050901992,
33.4339975214149,33.9298899526305,34.4257823838462,34.5575191894877),
 .UNSPECIFIED.);
#1421=B_SPLINE_CURVE_WITH_KNOTS('',3,(#53739,#53740,#53741,#53742,#53743,
#53744,#53745,#53746,#53747,#53748,#53749,#53750,#53751,#53752,#53753,#53754),
 .UNSPECIFIED.,.F.,.F.,(4,1,1,1,1,1,1,1,1,1,1,1,1,4),(28.2743338823081,
28.6366488330923,29.132541264308,29.6284336955237,30.1243261267394,30.6202185579551,
31.1161109891708,31.6120034203865,32.1078958516022,32.6037882828178,33.0996807140335,
33.5955731452492,34.0914655764649,34.5575191894877),.UNSPECIFIED.);
#1422=B_SPLINE_CURVE_WITH_KNOTS('',3,(#53759,#53760,#53761,#53762,#53763,
#53764,#53765,#53766,#53767,#53768,#53769,#53770,#53771,#53772,#53773,#53774,
#53775),.UNSPECIFIED.,.F.,.F.,(4,1,1,1,1,1,1,1,1,1,1,1,1,1,4),(21.9911485751285,
22.0284716034539,22.5243640346695,23.0202564658852,23.5161488971009,24.0120413283166,
24.5079337595323,25.003826190748,25.4997186219637,25.9956110531794,26.4915034843951,
26.9873959156108,27.4832883468265,27.9791807780422,28.2743338823081),
 .UNSPECIFIED.);
#1423=B_SPLINE_CURVE_WITH_KNOTS('',3,(#53776,#53777,#53778,#53779,#53780,
#53781,#53782,#53783,#53784,#53785,#53786,#53787,#53788,#53789,#53790,#53791,
#53792),.UNSPECIFIED.,.F.,.F.,(4,1,1,1,1,1,1,1,1,1,1,1,1,1,4),(21.9911485751285,
22.1900472272882,22.6859396585039,23.1818320897196,23.6777245209353,24.173616952151,
24.6695093833667,25.1654018145824,25.6612942457981,26.1571866770138,26.6530791082295,
27.1489715394452,27.6448639706609,28.1407564018766,28.2743338823081),
 .UNSPECIFIED.);
#1424=B_SPLINE_CURVE_WITH_KNOTS('',3,(#53797,#53798,#53799,#53800,#53801,
#53802,#53803,#53804,#53805,#53806,#53807,#53808,#53809,#53810,#53811,#53812),
 .UNSPECIFIED.,.F.,.F.,(4,1,1,1,1,1,1,1,1,1,1,1,1,4),(15.7079632679489,
16.0777624288655,16.5736548600812,17.0695472912969,17.5654397225126,18.0613321537283,
18.557224584944,19.0531170161597,19.5490094473754,20.0449018785911,20.5407943098068,
21.0366867410225,21.5325791722382,21.9911485751285),.UNSPECIFIED.);
#1425=B_SPLINE_CURVE_WITH_KNOTS('',3,(#53813,#53814,#53815,#53816,#53817,
#53818,#53819,#53820,#53821,#53822,#53823,#53824,#53825,#53826,#53827,#53828,
#53829),.UNSPECIFIED.,.F.,.F.,(4,1,1,1,1,1,1,1,1,1,1,1,1,1,4),(15.7079632679489,
15.7434456214842,16.2393380526999,16.7352304839156,17.2311229151313,17.727015346347,
18.2229077775627,18.7188002087784,19.2146926399941,19.7105850712098,20.2064775024255,
20.7023699336412,21.1982623648568,21.6941547960725,21.9911485751285),
 .UNSPECIFIED.);
#1426=B_SPLINE_CURVE_WITH_KNOTS('',3,(#53832,#53833,#53834,#53835,#53836,
#53837,#53838,#53839,#53840,#53841,#53842,#53843,#53844,#53845,#53846,#53847,
#53848,#53849,#53850,#53851,#53852,#53853,#53854,#53855,#53856,#53857,#53858,
#53859,#53860,#53861,#53862,#53863,#53864,#53865,#53866,#53867,#53868,#53869,
#53870,#53871,#53872,#53873,#53874,#53875,#53876,#53877,#53878,#53879,#53880,
#53881,#53882,#53883,#53884,#53885,#53886,#53887,#53888,#53889,#53890,#53891,
#53892,#53893,#53894,#53895,#53896,#53897,#53898,#53899,#53900,#53901,#53902,
#53903,#53904,#53905,#53906,#53907),.UNSPECIFIED.,.F.,.F.,(4,3,3,3,3,3,
3,3,3,3,3,3,3,3,3,3,3,3,3,3,3,3,3,3,3,4),(-1.56128884155279,-1.49877186936406,
-1.40897117371964,-1.3789451251186,-1.34973794742057,-1.24465351710347,
-1.19072852613426,-1.16409839319326,-1.13956908678638,-1.0343472120063,
-0.958854548039817,-0.923551939224775,-0.900234537445069,-0.87856017707745,
-0.769660548406124,-0.674675099932122,-0.618451862218184,-0.590493256446276,
-0.481235354793128,-0.389718754510115,-0.339912463836043,-0.311813120045921,
-0.289600014462053,-0.179535399263025,-0.0689290207122846,0.),
 .UNSPECIFIED.);
#1427=B_SPLINE_CURVE_WITH_KNOTS('',3,(#53912,#53913,#53914,#53915,#53916,
#53917,#53918,#53919,#53920,#53921,#53922,#53923,#53924,#53925,#53926,#53927,
#53928,#53929,#53930,#53931,#53932,#53933,#53934,#53935,#53936,#53937,#53938,
#53939,#53940,#53941,#53942,#53943,#53944,#53945,#53946,#53947,#53948,#53949,
#53950,#53951,#53952,#53953,#53954,#53955,#53956,#53957,#53958,#53959,#53960,
#53961,#53962,#53963,#53964,#53965,#53966,#53967,#53968,#53969,#53970,#53971,
#53972,#53973,#53974,#53975,#53976,#53977,#53978,#53979,#53980,#53981,#53982,
#53983,#53984,#53985,#53986,#53987),.UNSPECIFIED.,.F.,.F.,(4,3,3,3,3,3,
3,3,3,3,3,3,3,3,3,3,3,3,3,3,3,3,3,3,3,4),(-1.55754822368995,-1.48810779253287,
-1.39149025036148,-1.35765137174339,-1.33135607863307,-1.21649685124019,
-1.16749625285341,-1.1349192461529,-1.10163762384731,-0.993163332584848,
-0.919274261648977,-0.861029472187144,-0.839159851919032,-0.732654366492018,
-0.724432241811757,-0.63260971160265,-0.577457931216515,-0.548301984883685,
-0.443554340183684,-0.35714212097533,-0.309118804342202,-0.283551498142216,
-0.26428345496014,-0.160948967379259,-0.0591655876679145,0.),
 .UNSPECIFIED.);
#1428=B_SPLINE_CURVE_WITH_KNOTS('',3,(#54472,#54473,#54474,#54475,#54476,
#54477,#54478,#54479,#54480,#54481,#54482,#54483,#54484,#54485,#54486,#54487,
#54488,#54489,#54490,#54491,#54492,#54493,#54494,#54495,#54496,#54497,#54498,
#54499,#54500,#54501,#54502,#54503,#54504,#54505),.UNSPECIFIED.,.F.,.F.,
(4,3,3,3,3,3,3,3,3,3,3,4),(51.3852012649573,51.5728128464324,52.0687052776481,
52.5645977088638,53.0604901400795,53.5563825712952,54.0522750025108,54.5481674337265,
55.0440598649422,55.5399522961579,56.0358447273736,56.4439480094966),
 .UNSPECIFIED.);
#1429=B_SPLINE_CURVE_WITH_KNOTS('',3,(#54507,#54508,#54509,#54510,#54511,
#54512,#54513,#54514,#54515,#54516,#54517,#54518,#54519,#54520,#54521,#54522,
#54523,#54524,#54525,#54526,#54527,#54528,#54529,#54530,#54531,#54532,#54533,
#54534,#54535,#54536,#54537,#54538,#54539,#54540,#54541,#54542,#54543,#54544,
#54545,#54546,#54547,#54548,#54549,#54550,#54551,#54552,#54553,#54554,#54555,
#54556,#54557,#54558,#54559,#54560,#54561,#54562,#54563,#54564,#54565,#54566,
#54567,#54568,#54569,#54570,#54571,#54572,#54573,#54574,#54575,#54576,#54577,
#54578,#54579,#54580,#54581,#54582),.UNSPECIFIED.,.F.,.F.,(4,3,3,3,3,3,
3,3,3,3,3,3,3,3,3,3,3,3,3,3,3,3,3,3,3,4),(-1.56128884155278,-1.49877186936405,
-1.40897117371963,-1.37894512088796,-1.34973794578355,-1.24465351628496,
-1.19072853582439,-1.16409839418051,-1.13956908678636,-1.03434721514391,
-0.958854555599736,-0.923551951909299,-0.900234570307523,-0.878560184924177,
-0.76966054840611,-0.674675099932109,-0.618451846751326,-0.590493252166945,
-0.481235352814289,-0.389718754510105,-0.339912466184574,-0.311813126525562,
-0.289600022326692,-0.179535354639491,-0.0689290178359763,0.),
 .UNSPECIFIED.);
#1430=B_SPLINE_CURVE_WITH_KNOTS('',3,(#54583,#54584,#54585,#54586,#54587,
#54588,#54589,#54590,#54591,#54592,#54593,#54594,#54595,#54596),
 .UNSPECIFIED.,.F.,.F.,(4,1,1,1,1,1,1,1,1,1,1,4),(10.3764180272042,10.7845213093272,
11.2804137405429,11.7763061717586,12.2721986029743,12.76809103419,13.2639834654057,
13.7598758966214,14.2557683278371,14.7516607590528,15.2475531902685,15.7079632679489),
 .UNSPECIFIED.);
#1431=B_SPLINE_CURVE_WITH_KNOTS('',3,(#54600,#54601,#54602,#54603,#54604,
#54605,#54606,#54607,#54608,#54609,#54610,#54611),.UNSPECIFIED.,.F.,.F.,
(4,1,1,1,1,1,1,1,1,4),(11.6147305479242,12.1106229791399,12.6065154103556,
13.1024078415713,13.598300272787,14.0941927040027,14.5900851352184,15.0859775664341,
15.5818699976498,15.7079632679489),.UNSPECIFIED.);
#1432=B_SPLINE_CURVE_WITH_KNOTS('',3,(#55096,#55097,#55098,#55099,#55100,
#55101,#55102,#55103,#55104,#55105,#55106,#55107,#55108,#55109,#55110,#55111,
#55112,#55113,#55114,#55115,#55116,#55117,#55118,#55119,#55120,#55121,#55122,
#55123,#55124,#55125,#55126,#55127,#55128,#55129,#55130,#55131,#55132,#55133,
#55134,#55135,#55136,#55137,#55138,#55139,#55140,#55141,#55142,#55143,#55144,
#55145,#55146,#55147,#55148,#55149,#55150,#55151,#55152,#55153,#55154,#55155,
#55156,#55157,#55158,#55159,#55160,#55161,#55162,#55163,#55164,#55165,#55166,
#55167,#55168,#55169,#55170,#55171),.UNSPECIFIED.,.F.,.F.,(4,3,3,3,3,3,
3,3,3,3,3,3,3,3,3,3,3,3,3,3,3,3,3,3,3,4),(-1.55754822368999,-1.48810779253295,
-1.39149025036156,-1.35765138493943,-1.33135610631869,-1.21649686508303,
-1.16749627584831,-1.1349192463022,-1.10163762384737,-0.993163329305883,
-0.919274250510989,-0.861029455716102,-0.839159838745014,-0.732654337878835,
-0.724432241811784,-0.632609711602674,-0.57745792727088,-0.548301986226071,
-0.443554379365538,-0.357142120975343,-0.309118815124666,-0.28355153569308,
-0.264283499949117,-0.160949023485775,-0.0591655579179677,0.),
 .UNSPECIFIED.);
#1433=B_SPLINE_CURVE_WITH_KNOTS('',3,(#55172,#55173,#55174,#55175,#55176,
#55177,#55178,#55179,#55180,#55181,#55182,#55183,#55184,#55185,#55186,#55187,
#55188,#55189,#55190,#55191,#55192,#55193,#55194,#55195,#55196,#55197,#55198,
#55199),.UNSPECIFIED.,.F.,.F.,(4,3,3,3,3,3,3,3,3,4),(-58.5153068834521,
-58.0194144522364,-57.5235220210207,-57.027629589805,-56.5317371585893,
-56.0358447273736,-55.5399522961579,-55.0440598649422,-54.5481674337265,
-54.3587151774614),.UNSPECIFIED.);
#1434=B_SPLINE_CURVE_WITH_KNOTS('',3,(#55709,#55710,#55711,#55712,#55713,
#55714,#55715,#55716),.UNSPECIFIED.,.F.,.F.,(4,2,2,4),(0.,0.303392014531485,
0.493985861454505,0.65589637197807),.UNSPECIFIED.);
#1435=B_SPLINE_CURVE_WITH_KNOTS('',3,(#55718,#55719,#55720,#55721,#55722,
#55723,#55724,#55725,#55726,#55727,#55728,#55729,#55730,#55731,#55732,#55733,
#55734,#55735,#55736,#55737,#55738,#55739,#55740,#55741,#55742,#55743,#55744,
#55745,#55746,#55747,#55748,#55749,#55750,#55751,#55752,#55753,#55754,#55755,
#55756,#55757,#55758,#55759,#55760,#55761,#55762,#55763,#55764,#55765,#55766,
#55767,#55768,#55769,#55770,#55771,#55772,#55773,#55774,#55775,#55776,#55777,
#55778,#55779,#55780,#55781,#55782,#55783,#55784,#55785,#55786,#55787,#55788,
#55789,#55790,#55791,#55792,#55793,#55794,#55795,#55796,#55797,#55798,#55799,
#55800,#55801,#55802,#55803,#55804,#55805,#55806,#55807,#55808,#55809,#55810,
#55811,#55812,#55813,#55814,#55815,#55816,#55817,#55818,#55819,#55820,#55821,
#55822,#55823,#55824,#55825,#55826,#55827,#55828,#55829,#55830,#55831,#55832,
#55833,#55834,#55835,#55836,#55837,#55838,#55839,#55840,#55841,#55842,#55843,
#55844,#55845,#55846,#55847,#55848,#55849,#55850,#55851,#55852,#55853,#55854,
#55855,#55856,#55857,#55858,#55859,#55860,#55861,#55862,#55863,#55864,#55865,
#55866,#55867,#55868,#55869,#55870,#55871,#55872,#55873,#55874,#55875,#55876,
#55877,#55878,#55879,#55880,#55881,#55882,#55883,#55884,#55885,#55886,#55887,
#55888,#55889,#55890,#55891,#55892,#55893,#55894,#55895,#55896,#55897,#55898,
#55899,#55900,#55901,#55902,#55903,#55904,#55905,#55906,#55907,#55908,#55909,
#55910,#55911,#55912,#55913,#55914,#55915,#55916,#55917,#55918,#55919,#55920,
#55921,#55922,#55923,#55924,#55925,#55926,#55927,#55928,#55929,#55930,#55931,
#55932,#55933,#55934,#55935,#55936,#55937,#55938,#55939,#55940,#55941,#55942,
#55943,#55944,#55945,#55946,#55947,#55948,#55949,#55950,#55951,#55952,#55953,
#55954,#55955,#55956,#55957,#55958,#55959,#55960,#55961,#55962,#55963,#55964,
#55965,#55966,#55967,#55968,#55969,#55970,#55971,#55972,#55973,#55974,#55975,
#55976,#55977,#55978,#55979,#55980,#55981,#55982,#55983,#55984,#55985,#55986,
#55987,#55988,#55989,#55990,#55991,#55992,#55993,#55994,#55995,#55996,#55997,
#55998,#55999,#56000,#56001,#56002,#56003,#56004,#56005,#56006,#56007,#56008,
#56009),.UNSPECIFIED.,.F.,.F.,(4,3,3,3,3,3,3,3,3,3,3,3,3,3,3,3,3,3,3,3,
3,3,3,3,3,3,3,3,3,3,3,3,3,3,3,3,3,3,3,3,3,3,3,3,3,3,3,3,3,3,3,3,3,3,3,3,
3,3,3,3,3,3,3,3,3,3,3,3,3,3,3,3,3,3,3,3,3,3,3,3,3,3,3,3,3,3,3,3,3,3,3,3,
3,3,3,3,3,4),(0.,0.490398381839284,0.980796763678567,1.47119514551785,1.96159352735714,
2.45199190919642,2.9423902910357,3.43278867287499,3.92318705471427,4.41358543655355,
4.90398381839284,5.39438220023212,5.88478058207141,6.37517896391069,6.86557734574997,
7.35597572758925,7.84637410942854,8.33677249126782,8.82717087310711,9.31756925494639,
9.80796763678567,10.298366018625,10.7887644004642,11.2791627823035,11.7695611641428,
12.2599595459821,12.7503579278214,13.2407563096607,13.7311546914999,14.2215530733392,
14.7119514551785,15.2023498370178,15.6927482188571,16.1831466006964,16.6735449825356,
17.1639433643749,17.6543417462142,18.1447401280535,18.6351385098928,19.1255368917321,
19.6159352735713,20.1063336554106,20.5967320372499,21.0871304190892,21.5775288009285,
22.0679271827678,22.558325564607,23.0487239464463,23.5391223282856,24.0295207101249,
24.5199190919642,25.0103174738035,25.5007158556428,25.991114237482,26.4815126193213,
26.9719110011606,27.4623093829999,27.9527077648392,28.4431061466785,28.9335045285177,
29.423902910357,29.9143012921963,30.4046996740356,30.8950980558749,31.3854964377142,
31.8758948195534,32.3662932013927,32.856691583232,33.3470899650713,33.8374883469106,
34.3278867287499,34.8182851105891,35.3086834924284,35.7990818742677,36.289480256107,
36.7798786379463,37.2702770197856,37.7606754016249,38.2510737834641,38.7414721653034,
39.2318705471427,39.722268928982,40.2126673108213,40.7030656926605,41.1934640744998,
41.6838624563391,42.1742608381784,42.6646592200177,43.155057601857,43.6454559836963,
44.1358543655355,44.6262527473748,45.1166511292141,45.6070495110534,46.0974478928927,
46.587846274732,47.0782446565712,47.2939563352912),.UNSPECIFIED.);
#1436=B_SPLINE_CURVE_WITH_KNOTS('',3,(#56011,#56012,#56013,#56014,#56015,
#56016,#56017,#56018),.UNSPECIFIED.,.F.,.F.,(4,2,2,4),(-0.655895828583228,
-0.493988108841948,-0.303390394118163,0.),.UNSPECIFIED.);
#1437=B_SPLINE_CURVE_WITH_KNOTS('',3,(#56019,#56020,#56021,#56022,#56023,
#56024,#56025,#56026,#56027,#56028,#56029,#56030,#56031,#56032,#56033,#56034,
#56035,#56036,#56037,#56038,#56039,#56040,#56041,#56042,#56043,#56044,#56045,
#56046,#56047,#56048,#56049,#56050,#56051,#56052,#56053,#56054,#56055,#56056,
#56057,#56058,#56059,#56060,#56061,#56062,#56063,#56064,#56065,#56066,#56067,
#56068,#56069,#56070,#56071,#56072,#56073,#56074,#56075,#56076,#56077,#56078,
#56079,#56080,#56081,#56082,#56083,#56084,#56085,#56086,#56087,#56088,#56089,
#56090,#56091,#56092,#56093,#56094,#56095,#56096,#56097,#56098,#56099,#56100,
#56101,#56102,#56103,#56104,#56105,#56106,#56107,#56108,#56109,#56110,#56111,
#56112,#56113,#56114,#56115,#56116,#56117,#56118),.UNSPECIFIED.,.F.,.F.,
(4,1,1,1,1,1,1,1,1,1,1,1,1,1,1,1,1,1,1,1,1,1,1,1,1,1,1,1,1,1,1,1,1,1,1,
1,1,1,1,1,1,1,1,1,1,1,1,1,1,1,1,1,1,1,1,1,1,1,1,1,1,1,1,1,1,1,1,1,1,1,1,
1,1,1,1,1,1,1,1,1,1,1,1,1,1,1,1,1,1,1,1,1,1,1,1,1,1,4),(7.04827039213812,
7.26398207085812,7.7543804526974,8.24477883453668,8.73517721637597,9.22557559821525,
9.71597398005454,10.2063723618938,10.6967707437331,11.1871691255724,11.6775675074117,
12.167965889251,12.6583642710902,13.1487626529295,13.6391610347688,14.1295594166081,
14.6199577984474,15.1103561802867,15.6007545621259,16.0911529439652,16.5815513258045,
17.0719497076438,17.5623480894831,18.0527464713224,18.5431448531616,19.0335432350009,
19.5239416168402,20.0143399986795,20.5047383805188,20.9951367623581,21.4855351441973,
21.9759335260366,22.4663319078759,22.9567302897152,23.4471286715545,23.9375270533938,
24.427925435233,24.9183238170723,25.4087221989116,25.8991205807509,26.3895189625902,
26.8799173444295,27.3703157262687,27.860714108108,28.3511124899473,28.8415108717866,
29.3319092536259,29.8223076354652,30.3127060173044,30.8031043991437,31.293502780983,
31.7839011628223,32.2742995446616,32.7646979265009,33.2550963083402,33.7454946901794,
34.2358930720187,34.726291453858,35.2166898356973,35.7070882175366,36.1974865993759,
36.6878849812151,37.1782833630544,37.6686817448937,38.159080126733,38.6494785085723,
39.1398768904116,39.6302752722508,40.1206736540901,40.6110720359294,41.1014704177687,
41.591868799608,42.0822671814473,42.5726655632865,43.0630639451258,43.5534623269651,
44.0438607088044,44.5342590906437,45.024657472483,45.5150558543222,46.0054542361615,
46.4958526180008,46.9862509998401,47.4766493816794,47.9670477635187,48.457446145358,
48.9478445271972,49.4382429090365,49.9286412908758,50.4190396727151,50.9094380545544,
51.3998364363937,51.8902348182329,52.3806332000722,52.8710315819115,53.3614299637508,
53.8518283455901,54.3422267274294),.UNSPECIFIED.);
#1438=B_SPLINE_CURVE_WITH_KNOTS('',3,(#56524,#56525,#56526,#56527,#56528,
#56529,#56530,#56531,#56532,#56533,#56534,#56535,#56536,#56537,#56538,#56539,
#56540,#56541,#56542,#56543,#56544,#56545,#56546,#56547,#56548,#56549,#56550,
#56551,#56552,#56553,#56554,#56555,#56556,#56557,#56558,#56559,#56560,#56561,
#56562,#56563,#56564,#56565,#56566,#56567,#56568,#56569,#56570,#56571,#56572,
#56573,#56574,#56575),.UNSPECIFIED.,.F.,.F.,(4,3,3,3,3,3,3,3,3,3,3,3,3,
3,3,3,3,4),(0.,0.113340575159286,0.226679014316618,0.308971226981702,0.331574139310527,
0.375660801919039,0.487626538864782,0.577647057862927,0.619647639303814,
0.642726778605582,0.752674952029806,0.769690750751167,0.865631662359539,
0.890410497302428,0.914699066250878,1.0235933762904,1.13055552817073,1.15345439718465),
 .UNSPECIFIED.);
#1439=B_SPLINE_CURVE_WITH_KNOTS('',3,(#56577,#56578,#56579,#56580,#56581,
#56582,#56583,#56584,#56585,#56586,#56587,#56588,#56589,#56590,#56591,#56592,
#56593,#56594,#56595,#56596,#56597,#56598,#56599,#56600,#56601,#56602,#56603,
#56604,#56605,#56606,#56607,#56608,#56609,#56610,#56611,#56612,#56613,#56614,
#56615,#56616,#56617,#56618,#56619,#56620,#56621,#56622,#56623,#56624,#56625),
 .UNSPECIFIED.,.F.,.F.,(4,3,3,3,3,3,3,3,3,3,3,3,3,3,3,3,4),(-1.15345439718468,
-1.04561219422299,-0.936713145930054,-0.898860433224846,-0.874966557590888,
-0.796527420497185,-0.69819122971956,-0.637686241518252,-0.608878950479122,
-0.496956393343038,-0.403182657386683,-0.351450861948057,-0.31601513468901,
-0.29336187161946,-0.180573976425843,-0.067406475320211,0.),
 .UNSPECIFIED.);
#1440=B_SPLINE_CURVE_WITH_KNOTS('',3,(#56626,#56627,#56628,#56629,#56630,
#56631,#56632,#56633,#56634,#56635,#56636,#56637,#56638,#56639,#56640,#56641,
#56642,#56643,#56644,#56645,#56646,#56647,#56648,#56649,#56650,#56651,#56652,
#56653,#56654,#56655,#56656,#56657,#56658,#56659,#56660,#56661,#56662,#56663,
#56664,#56665,#56666,#56667,#56668,#56669,#56670,#56671,#56672,#56673,#56674,
#56675,#56676,#56677,#56678,#56679,#56680,#56681,#56682,#56683,#56684,#56685,
#56686,#56687,#56688,#56689,#56690,#56691,#56692,#56693,#56694,#56695,#56696,
#56697,#56698,#56699,#56700,#56701,#56702,#56703,#56704,#56705,#56706,#56707,
#56708,#56709,#56710,#56711,#56712,#56713,#56714,#56715,#56716,#56717,#56718,
#56719,#56720,#56721,#56722,#56723,#56724),.UNSPECIFIED.,.F.,.F.,(4,1,1,
1,1,1,1,1,1,1,1,1,1,1,1,1,1,1,1,1,1,1,1,1,1,1,1,1,1,1,1,1,1,1,1,1,1,1,1,
1,1,1,1,1,1,1,1,1,1,1,1,1,1,1,1,1,1,1,1,1,1,1,1,1,1,1,1,1,1,1,1,1,1,1,1,
1,1,1,1,1,1,1,1,1,1,1,1,1,1,1,1,1,1,1,1,1,4),(8.50634549793093,8.54067951788559,
9.03814922646808,9.53561893505058,10.0330886436331,10.5305583522156,11.028028060798,
11.5254977693805,12.022967477963,12.5204371865455,13.017906895128,13.5153766037105,
14.012846312293,14.5103160208755,15.007785729458,15.5052554380405,16.002725146623,
16.5001948552054,16.9976645637879,17.4951342723704,17.9926039809529,18.4900736895354,
18.9875433981179,19.4850131067004,19.9824828152829,20.4799525238654,20.9774222324479,
21.4748919410303,21.9723616496128,22.4698313581953,22.9673010667778,23.4647707753603,
23.9622404839428,24.4597101925253,24.9571799011078,25.4546496096903,25.9521193182728,
26.4495890268552,26.9470587354377,27.4445284440202,27.9419981526027,28.4394678611852,
28.9369375697677,29.4344072783502,29.9318769869327,30.4293466955152,30.9268164040977,
31.4242861126801,31.9217558212626,32.4192255298451,32.9166952384276,33.4141649470101,
33.9116346555926,34.4091043641751,34.9065740727576,35.4040437813401,35.9015134899226,
36.3989831985051,36.8964529070875,37.39392261567,37.8913923242525,38.388862032835,
38.8863317414175,39.38380145,39.8812711585825,40.378740867165,40.8762105757475,
41.37368028433,41.8711499929124,42.3686197014949,42.8660894100774,43.3635591186599,
43.8610288272424,44.3584985358249,44.8559682444074,45.3534379529899,45.8509076615724,
46.3483773701549,46.8458470787373,47.3433167873198,47.8407864959023,48.3382562044848,
48.8357259130673,49.3331956216498,49.8306653302323,50.3281350388148,50.8256047473973,
51.3230744559798,51.8205441645622,52.3180138731447,52.8154835817272,53.3129532903097,
53.8104229988922,54.3078927074747,54.8053624160572,55.3028321246397,55.8003018332222),
 .UNSPECIFIED.);
#1441=B_SPLINE_CURVE_WITH_KNOTS('',3,(#57230,#57231,#57232,#57233,#57234,
#57235,#57236,#57237),.UNSPECIFIED.,.F.,.F.,(4,2,2,4),(0.,0.169060128143182,
0.25966506968926,0.35733520735872),.UNSPECIFIED.);
#1442=B_SPLINE_CURVE_WITH_KNOTS('',3,(#57239,#57240,#57241,#57242,#57243,
#57244,#57245,#57246),.UNSPECIFIED.,.F.,.F.,(4,2,2,4),(-0.357325312875914,
-0.25966481301295,-0.16906915003162,0.),.UNSPECIFIED.);
#1443=B_SPLINE_CURVE_WITH_KNOTS('',3,(#57247,#57248,#57249,#57250),
 .UNSPECIFIED.,.F.,.F.,(4,4),(9.27143058288951,9.42477796076936),
 .UNSPECIFIED.);
#1444=B_SPLINE_CURVE_WITH_KNOTS('',3,(#57256,#57257,#57258,#57259,#57260,
#57261,#57262,#57263),.UNSPECIFIED.,.F.,.F.,(4,2,2,4),(-0.415677006509057,
-0.30010857089105,-0.193253093542049,0.),.UNSPECIFIED.);
#1445=B_SPLINE_CURVE_WITH_KNOTS('',3,(#57265,#57266,#57267,#57268,#57269,
#57270,#57271,#57272,#57273,#57274,#57275,#57276,#57277,#57278,#57279,#57280,
#57281,#57282,#57283,#57284,#57285,#57286,#57287,#57288,#57289,#57290,#57291,
#57292,#57293,#57294,#57295,#57296,#57297,#57298,#57299,#57300,#57301,#57302,
#57303,#57304,#57305,#57306,#57307,#57308,#57309,#57310,#57311,#57312,#57313),
 .UNSPECIFIED.,.F.,.F.,(4,3,3,3,3,3,3,3,3,3,3,3,3,3,3,3,4),(-1.15166532125565,
-1.03829677946551,-0.92526093057982,-0.889798588874102,-0.85795025740414,
-0.776795567921361,-0.678445564828449,-0.620287810074995,-0.586753712344781,
-0.476556476810445,-0.383395555549714,-0.332702788626492,-0.305063279672108,
-0.282851348870515,-0.174044273873872,-0.0667784584837768,0.),
 .UNSPECIFIED.);
#1446=B_SPLINE_CURVE_WITH_KNOTS('',3,(#57314,#57315,#57316,#57317,#57318,
#57319),.UNSPECIFIED.,.F.,.F.,(4,2,4),(-0.659276662925401,-0.291453031942629,
0.),.UNSPECIFIED.);
#1447=B_SPLINE_CURVE_WITH_KNOTS('',3,(#57828,#57829,#57830,#57831,#57832,
#57833),.UNSPECIFIED.,.F.,.F.,(4,2,4),(0.,0.291454760594753,0.659275699695543),
 .UNSPECIFIED.);
#1448=B_SPLINE_CURVE_WITH_KNOTS('',3,(#57834,#57835,#57836,#57837,#57838,
#57839,#57840,#57841,#57842,#57843,#57844,#57845,#57846,#57847,#57848,#57849,
#57850,#57851,#57852,#57853,#57854,#57855,#57856,#57857,#57858,#57859,#57860,
#57861,#57862,#57863,#57864,#57865,#57866,#57867,#57868,#57869,#57870,#57871,
#57872,#57873,#57874,#57875,#57876,#57877,#57878,#57879,#57880,#57881,#57882,
#57883,#57884,#57885,#57886,#57887,#57888,#57889,#57890,#57891,#57892,#57893,
#57894,#57895,#57896,#57897,#57898,#57899,#57900,#57901,#57902,#57903,#57904,
#57905,#57906,#57907,#57908,#57909,#57910,#57911,#57912,#57913,#57914,#57915,
#57916,#57917,#57918,#57919,#57920,#57921,#57922,#57923,#57924,#57925,#57926,
#57927,#57928,#57929,#57930,#57931,#57932,#57933),.UNSPECIFIED.,.F.,.F.,
(4,1,1,1,1,1,1,1,1,1,1,1,1,1,1,1,1,1,1,1,1,1,1,1,1,1,1,1,1,1,1,1,1,1,1,
1,1,1,1,1,1,1,1,1,1,1,1,1,1,1,1,1,1,1,1,1,1,1,1,1,1,1,1,1,1,1,1,1,1,1,1,
1,1,1,1,1,1,1,1,1,1,1,1,1,1,1,1,1,1,1,1,1,1,1,1,1,1,4),(10.3432104236077,
10.5589221023277,11.049320484167,11.5397188660063,12.0301172478456,12.5205156296849,
13.0109140115242,13.5013123933634,13.9917107752027,14.482109157042,14.9725075388813,
15.4629059207206,15.9533043025599,16.4437026843991,16.9341010662384,17.4244994480777,
17.914897829917,18.4052962117563,18.8956945935956,19.3860929754348,19.8764913572741,
20.3668897391134,20.8572881209527,21.347686502792,21.8380848846313,22.3284832664706,
22.8188816483098,23.3092800301491,23.7996784119884,24.2900767938277,24.780475175667,
25.2708735575063,25.7612719393455,26.2516703211848,26.7420687030241,27.2324670848634,
27.7228654667027,28.213263848542,28.7036622303812,29.1940606122205,29.6844589940598,
30.1748573758991,30.6652557577384,31.1556541395777,31.6460525214169,32.1364509032562,
32.6268492850955,33.1172476669348,33.6076460487741,34.0980444306134,34.5884428124527,
35.0788411942919,35.5692395761312,36.0596379579705,36.5500363398098,37.0404347216491,
37.5308331034883,38.0212314853276,38.5116298671669,39.0020282490062,39.4924266308455,
39.9828250126848,40.4732233945241,40.9636217763633,41.4540201582026,41.9444185400419,
42.4348169218812,42.9252153037205,43.4156136855598,43.906012067399,44.3964104492383,
44.8868088310776,45.3772072129169,45.8676055947562,46.3580039765955,46.8484023584347,
47.338800740274,47.8291991221133,48.3195975039526,48.8099958857919,49.3003942676312,
49.7907926494704,50.2811910313097,50.771589413149,51.2619877949883,51.7523861768276,
52.2427845586669,52.7331829405062,53.2235813223454,53.7139797041847,54.204378086024,
54.6947764678633,55.1851748497026,55.6755732315419,56.1659716133811,56.6563699952204,
57.1467683770597,57.637166758899),.UNSPECIFIED.);
#1449=B_SPLINE_CURVE_WITH_KNOTS('',3,(#58339,#58340,#58341,#58342,#58343,
#58344,#58345,#58346,#58347,#58348,#58349,#58350,#58351,#58352,#58353,#58354,
#58355,#58356,#58357,#58358,#58359,#58360,#58361,#58362,#58363,#58364,#58365,
#58366,#58367,#58368,#58369,#58370,#58371,#58372,#58373,#58374,#58375,#58376,
#58377,#58378,#58379,#58380,#58381,#58382,#58383,#58384,#58385,#58386,#58387,
#58388,#58389,#58390),.UNSPECIFIED.,.F.,.F.,(4,3,3,3,3,3,3,3,3,3,3,3,3,
3,3,3,3,4),(0.,0.107536136059347,0.21639745378144,0.296736912823596,0.319843387979014,
0.356604402276687,0.466524670541788,0.54707448357054,0.595815754023213,
0.619047604474437,0.731049962221955,0.749314772119391,0.84990240940345,
0.873496420034821,0.898389588326068,1.01139267283444,1.12432918312036,1.15166532125563),
 .UNSPECIFIED.);
#1450=B_SPLINE_CURVE_WITH_KNOTS('',3,(#58391,#58392,#58393,#58394,#58395,
#58396,#58397,#58398,#58399,#58400,#58401,#58402,#58403,#58404,#58405,#58406,
#58407,#58408,#58409,#58410,#58411,#58412,#58413,#58414,#58415,#58416,#58417,
#58418,#58419,#58420,#58421,#58422,#58423,#58424,#58425,#58426,#58427,#58428,
#58429,#58430,#58431,#58432,#58433,#58434,#58435,#58436,#58437,#58438,#58439,
#58440,#58441,#58442,#58443,#58444,#58445,#58446,#58447,#58448,#58449,#58450,
#58451,#58452,#58453,#58454,#58455,#58456,#58457,#58458,#58459,#58460,#58461,
#58462,#58463,#58464,#58465,#58466,#58467,#58468,#58469,#58470,#58471,#58472,
#58473,#58474,#58475,#58476,#58477,#58478,#58479,#58480,#58481,#58482,#58483,
#58484,#58485,#58486,#58487,#58488,#58489),.UNSPECIFIED.,.F.,.F.,(4,1,1,
1,1,1,1,1,1,1,1,1,1,1,1,1,1,1,1,1,1,1,1,1,1,1,1,1,1,1,1,1,1,1,1,1,1,1,1,
1,1,1,1,1,1,1,1,1,1,1,1,1,1,1,1,1,1,1,1,1,1,1,1,1,1,1,1,1,1,1,1,1,1,1,1,
1,1,1,1,1,1,1,1,1,1,1,1,1,1,1,1,1,1,1,1,1,4),(11.8012855294006,11.8356195493552,
12.3330892579377,12.8305589665202,13.3280286751027,13.8254983836852,14.3229680922677,
14.8204378008502,15.3179075094327,15.8153772180151,16.3128469265976,16.8103166351801,
17.3077863437626,17.8052560523451,18.3027257609276,18.8001954695101,19.2976651780926,
19.7951348866751,20.2926045952576,20.79007430384,21.2875440124225,21.785013721005,
22.2824834295875,22.77995313817,23.2774228467525,23.774892555335,24.2723622639175,
24.7698319725,25.2673016810825,25.7647713896649,26.2622410982474,26.7597108068299,
27.2571805154124,27.7546502239949,28.2521199325774,28.7495896411599,29.2470593497424,
29.7445290583249,30.2419987669074,30.7394684754899,31.2369381840723,31.7344078926548,
32.2318776012373,32.7293473098198,33.2268170184023,33.7242867269848,34.2217564355673,
34.7192261441498,35.2166958527323,35.7141655613148,36.2116352698972,36.7091049784797,
37.2065746870622,37.7040443956447,38.2015141042272,38.6989838128097,39.1964535213922,
39.6939232299747,40.1913929385572,40.6888626471397,41.1863323557221,41.6838020643046,
42.1812717728871,42.6787414814696,43.1762111900521,43.6736808986346,44.1711506072171,
44.6686203157996,45.1660900243821,45.6635597329646,46.1610294415471,46.6584991501295,
47.155968858712,47.6534385672945,48.150908275877,48.6483779844595,49.145847693042,
49.6433174016245,50.140787110207,50.6382568187895,51.135726527372,51.6331962359544,
52.1306659445369,52.6281356531194,53.1256053617019,53.6230750702844,54.1205447788669,
54.6180144874494,55.1154841960319,55.6129539046144,56.1104236131969,56.6078933217793,
57.1053630303618,57.6028327389443,58.1003024475268,58.5977721561093,59.0952418646918),
 .UNSPECIFIED.);
#1451=B_SPLINE_CURVE_WITH_KNOTS('',3,(#58995,#58996,#58997,#58998,#58999,
#59000,#59001,#59002),.UNSPECIFIED.,.F.,.F.,(4,2,2,4),(0.,0.19323696658513,
0.300098749787172,0.415673620383952),.UNSPECIFIED.);
#1494=(
BOUNDED_CURVE()
B_SPLINE_CURVE(2,(#59009,#59010,#59011),.UNSPECIFIED.,.F.,.F.)
B_SPLINE_CURVE_WITH_KNOTS((3,3),(0.0827095041446621,0.74095125061019),
 .UNSPECIFIED.)
CURVE()
GEOMETRIC_REPRESENTATION_ITEM()
RATIONAL_B_SPLINE_CURVE((1.02109552796081,1.1000775419169,1.1000775419169))
REPRESENTATION_ITEM('')
);
#1495=(
BOUNDED_CURVE()
B_SPLINE_CURVE(2,(#59013,#59014,#59015),.UNSPECIFIED.,.F.,.F.)
B_SPLINE_CURVE_WITH_KNOTS((3,3),(0.0827095041446618,1.39919299707572),
 .UNSPECIFIED.)
CURVE()
GEOMETRIC_REPRESENTATION_ITEM()
RATIONAL_B_SPLINE_CURVE((1.02109552796081,1.17905955587299,1.02109552796081))
REPRESENTATION_ITEM('')
);
#1496=(
BOUNDED_CURVE()
B_SPLINE_CURVE(2,(#59017,#59018,#59019),.UNSPECIFIED.,.F.,.F.)
B_SPLINE_CURVE_WITH_KNOTS((3,3),(0.082709504144662,1.39919299707572),
 .UNSPECIFIED.)
CURVE()
GEOMETRIC_REPRESENTATION_ITEM()
RATIONAL_B_SPLINE_CURVE((1.02109552796081,1.17905955587299,1.02109552796081))
REPRESENTATION_ITEM('')
);
#1497=(
BOUNDED_CURVE()
B_SPLINE_CURVE(2,(#59021,#59022,#59023),.UNSPECIFIED.,.F.,.F.)
B_SPLINE_CURVE_WITH_KNOTS((3,3),(0.0827095041446621,1.39919299707572),
 .UNSPECIFIED.)
CURVE()
GEOMETRIC_REPRESENTATION_ITEM()
RATIONAL_B_SPLINE_CURVE((1.02109552796081,1.17905955587299,1.02109552796081))
REPRESENTATION_ITEM('')
);
#1498=(
BOUNDED_CURVE()
B_SPLINE_CURVE(2,(#59025,#59026,#59027),.UNSPECIFIED.,.F.,.F.)
B_SPLINE_CURVE_WITH_KNOTS((3,3),(0.0827095041446625,1.39919299707572),
 .UNSPECIFIED.)
CURVE()
GEOMETRIC_REPRESENTATION_ITEM()
RATIONAL_B_SPLINE_CURVE((1.02109552796081,1.17905955587299,1.02109552796081))
REPRESENTATION_ITEM('')
);
#1499=(
BOUNDED_CURVE()
B_SPLINE_CURVE(2,(#59029,#59030,#59031),.UNSPECIFIED.,.F.,.F.)
B_SPLINE_CURVE_WITH_KNOTS((3,3),(0.0827095041446619,1.39919299707572),
 .UNSPECIFIED.)
CURVE()
GEOMETRIC_REPRESENTATION_ITEM()
RATIONAL_B_SPLINE_CURVE((1.02109552796081,1.17905955587299,1.02109552796081))
REPRESENTATION_ITEM('')
);
#1500=(
BOUNDED_CURVE()
B_SPLINE_CURVE(2,(#59032,#59033,#59034),.UNSPECIFIED.,.F.,.F.)
B_SPLINE_CURVE_WITH_KNOTS((3,3),(0.74095125061019,1.39919299707572),
 .UNSPECIFIED.)
CURVE()
GEOMETRIC_REPRESENTATION_ITEM()
RATIONAL_B_SPLINE_CURVE((1.1000775419169,1.1000775419169,1.02109552796081))
REPRESENTATION_ITEM('')
);
#1501=(
BOUNDED_CURVE()
B_SPLINE_CURVE(2,(#59039,#59040,#59041),.UNSPECIFIED.,.F.,.F.)
B_SPLINE_CURVE_WITH_KNOTS((3,3),(0.0827095041446625,1.39919299707572),
 .UNSPECIFIED.)
CURVE()
GEOMETRIC_REPRESENTATION_ITEM()
RATIONAL_B_SPLINE_CURVE((1.02109552796081,1.17905955587299,1.02109552796081))
REPRESENTATION_ITEM('')
);
#1502=(
BOUNDED_CURVE()
B_SPLINE_CURVE(2,(#59046,#59047,#59048),.UNSPECIFIED.,.F.,.F.)
B_SPLINE_CURVE_WITH_KNOTS((3,3),(0.0827095041446616,1.39919299707572),
 .UNSPECIFIED.)
CURVE()
GEOMETRIC_REPRESENTATION_ITEM()
RATIONAL_B_SPLINE_CURVE((1.02109552796081,1.17905955587299,1.02109552796081))
REPRESENTATION_ITEM('')
);
#1503=(
BOUNDED_CURVE()
B_SPLINE_CURVE(2,(#59052,#59053,#59054),.UNSPECIFIED.,.F.,.F.)
B_SPLINE_CURVE_WITH_KNOTS((3,3),(0.082709504144662,1.39919299707572),
 .UNSPECIFIED.)
CURVE()
GEOMETRIC_REPRESENTATION_ITEM()
RATIONAL_B_SPLINE_CURVE((1.02109552796081,1.17905955587299,1.02109552796081))
REPRESENTATION_ITEM('')
);
#1504=(
BOUNDED_CURVE()
B_SPLINE_CURVE(2,(#59057,#59058,#59059),.UNSPECIFIED.,.F.,.F.)
B_SPLINE_CURVE_WITH_KNOTS((3,3),(0.0827095041446617,1.39919299707572),
 .UNSPECIFIED.)
CURVE()
GEOMETRIC_REPRESENTATION_ITEM()
RATIONAL_B_SPLINE_CURVE((1.02109552796081,1.17905955587299,1.02109552796081))
REPRESENTATION_ITEM('')
);
#1505=(
BOUNDED_CURVE()
B_SPLINE_CURVE(2,(#59061,#59062,#59063),.UNSPECIFIED.,.F.,.F.)
B_SPLINE_CURVE_WITH_KNOTS((3,3),(0.74095125061019,1.39919299707572),
 .UNSPECIFIED.)
CURVE()
GEOMETRIC_REPRESENTATION_ITEM()
RATIONAL_B_SPLINE_CURVE((1.1000775419169,1.1000775419169,1.02109552796081))
REPRESENTATION_ITEM('')
);
#1506=(
BOUNDED_CURVE()
B_SPLINE_CURVE(2,(#59068,#59069,#59070),.UNSPECIFIED.,.F.,.F.)
B_SPLINE_CURVE_WITH_KNOTS((3,3),(0.0827095041446617,0.74095125061019),
 .UNSPECIFIED.)
CURVE()
GEOMETRIC_REPRESENTATION_ITEM()
RATIONAL_B_SPLINE_CURVE((1.02109552796081,1.1000775419169,1.1000775419169))
REPRESENTATION_ITEM('')
);
#1507=(
BOUNDED_CURVE()
B_SPLINE_CURVE(2,(#59071,#59072,#59073),.UNSPECIFIED.,.F.,.F.)
B_SPLINE_CURVE_WITH_KNOTS((3,3),(0.0827095041446618,1.39919299707572),
 .UNSPECIFIED.)
CURVE()
GEOMETRIC_REPRESENTATION_ITEM()
RATIONAL_B_SPLINE_CURVE((1.02109552796081,1.17905955587299,1.02109552796081))
REPRESENTATION_ITEM('')
);
#1527=SHAPE_REPRESENTATION_RELATIONSHIP('SRR','None',#59316,#1547);
#1547=ADVANCED_BREP_SHAPE_REPRESENTATION('',(#1594),#59203);
#1574=STYLED_ITEM('',(#59572),#1594);
#1594=MANIFOLD_SOLID_BREP('Stud body',#22823);
#1805=FACE_BOUND('',#5471,.T.);
#1806=FACE_BOUND('',#5474,.T.);
#1807=FACE_BOUND('',#5481,.T.);
#1808=FACE_BOUND('',#5484,.T.);
#1809=FACE_BOUND('',#5488,.T.);
#2394=PLANE('',#25027);
#2395=PLANE('',#25034);
#2396=PLANE('',#25041);
#2397=PLANE('',#25042);
#2398=PLANE('',#25043);
#2399=PLANE('',#25046);
#2400=PLANE('',#25047);
#2401=PLANE('',#25048);
#2402=PLANE('',#25050);
#2403=PLANE('',#25052);
#2404=PLANE('',#25054);
#2405=PLANE('',#25055);
#2406=PLANE('',#25060);
#2407=PLANE('',#25063);
#2408=PLANE('',#25068);
#2637=CYLINDRICAL_SURFACE('',#24997,0.7475);
#2638=CYLINDRICAL_SURFACE('',#24999,0.7475);
#2639=CYLINDRICAL_SURFACE('',#25000,0.7475);
#2640=CYLINDRICAL_SURFACE('',#25001,0.7475);
#2641=CYLINDRICAL_SURFACE('',#25002,0.7475);
#2642=CYLINDRICAL_SURFACE('',#25003,0.7475);
#2643=CYLINDRICAL_SURFACE('',#25004,0.7475);
#2644=CYLINDRICAL_SURFACE('',#25005,0.7475);
#2645=CYLINDRICAL_SURFACE('',#25007,0.7925);
#2646=CYLINDRICAL_SURFACE('',#25009,0.7925);
#2647=CYLINDRICAL_SURFACE('',#25010,0.7925);
#2648=CYLINDRICAL_SURFACE('',#25011,0.7925);
#2649=CYLINDRICAL_SURFACE('',#25012,0.7925);
#2650=CYLINDRICAL_SURFACE('',#25013,0.7925);
#2651=CYLINDRICAL_SURFACE('',#25014,0.7925);
#2652=CYLINDRICAL_SURFACE('',#25015,0.7925);
#2653=CYLINDRICAL_SURFACE('',#25016,0.7925);
#2654=CYLINDRICAL_SURFACE('',#25017,0.70685);
#2655=CYLINDRICAL_SURFACE('',#25019,0.70685);
#2656=CYLINDRICAL_SURFACE('',#25020,0.70685);
#2657=CYLINDRICAL_SURFACE('',#25021,0.70685);
#2658=CYLINDRICAL_SURFACE('',#25022,0.70685);
#2659=CYLINDRICAL_SURFACE('',#25023,0.70685);
#2660=CYLINDRICAL_SURFACE('',#25024,0.70685);
#2661=CYLINDRICAL_SURFACE('',#25025,0.70685);
#2662=CYLINDRICAL_SURFACE('',#25026,0.70685);
#2663=CYLINDRICAL_SURFACE('',#25030,0.70685);
#2664=CYLINDRICAL_SURFACE('',#25032,0.7925);
#2665=CYLINDRICAL_SURFACE('',#25038,0.7475);
#2666=CYLINDRICAL_SURFACE('',#25056,0.4);
#2667=CYLINDRICAL_SURFACE('',#25058,0.4);
#2668=CYLINDRICAL_SURFACE('',#25065,0.7431);
#3914=FACE_OUTER_BOUND('',#5425,.T.);
#3915=FACE_OUTER_BOUND('',#5426,.T.);
#3916=FACE_OUTER_BOUND('',#5427,.T.);
#3917=FACE_OUTER_BOUND('',#5428,.T.);
#3918=FACE_OUTER_BOUND('',#5429,.T.);
#3919=FACE_OUTER_BOUND('',#5430,.T.);
#3920=FACE_OUTER_BOUND('',#5431,.T.);
#3921=FACE_OUTER_BOUND('',#5432,.T.);
#3922=FACE_OUTER_BOUND('',#5433,.T.);
#3923=FACE_OUTER_BOUND('',#5434,.T.);
#3924=FACE_OUTER_BOUND('',#5435,.T.);
#3925=FACE_OUTER_BOUND('',#5436,.T.);
#3926=FACE_OUTER_BOUND('',#5437,.T.);
#3927=FACE_OUTER_BOUND('',#5438,.T.);
#3928=FACE_OUTER_BOUND('',#5439,.T.);
#3929=FACE_OUTER_BOUND('',#5440,.T.);
#3930=FACE_OUTER_BOUND('',#5441,.T.);
#3931=FACE_OUTER_BOUND('',#5442,.T.);
#3932=FACE_OUTER_BOUND('',#5443,.T.);
#3933=FACE_OUTER_BOUND('',#5444,.T.);
#3934=FACE_OUTER_BOUND('',#5445,.T.);
#3935=FACE_OUTER_BOUND('',#5446,.T.);
#3936=FACE_OUTER_BOUND('',#5447,.T.);
#3937=FACE_OUTER_BOUND('',#5448,.T.);
#3938=FACE_OUTER_BOUND('',#5449,.T.);
#3939=FACE_OUTER_BOUND('',#5450,.T.);
#3940=FACE_OUTER_BOUND('',#5451,.T.);
#3941=FACE_OUTER_BOUND('',#5452,.T.);
#3942=FACE_OUTER_BOUND('',#5453,.T.);
#3943=FACE_OUTER_BOUND('',#5454,.T.);
#3944=FACE_OUTER_BOUND('',#5455,.T.);
#3945=FACE_OUTER_BOUND('',#5456,.T.);
#3946=FACE_OUTER_BOUND('',#5457,.T.);
#3947=FACE_OUTER_BOUND('',#5458,.T.);
#3948=FACE_OUTER_BOUND('',#5459,.T.);
#3949=FACE_OUTER_BOUND('',#5460,.T.);
#3950=FACE_OUTER_BOUND('',#5461,.T.);
#3951=FACE_OUTER_BOUND('',#5462,.T.);
#3952=FACE_OUTER_BOUND('',#5463,.T.);
#3953=FACE_OUTER_BOUND('',#5464,.T.);
#3954=FACE_OUTER_BOUND('',#5465,.T.);
#3955=FACE_OUTER_BOUND('',#5466,.T.);
#3956=FACE_OUTER_BOUND('',#5467,.T.);
#3957=FACE_OUTER_BOUND('',#5468,.T.);
#3958=FACE_OUTER_BOUND('',#5469,.T.);
#3959=FACE_OUTER_BOUND('',#5470,.T.);
#3960=FACE_OUTER_BOUND('',#5472,.T.);
#3961=FACE_OUTER_BOUND('',#5473,.T.);
#3962=FACE_OUTER_BOUND('',#5475,.T.);
#3963=FACE_OUTER_BOUND('',#5476,.T.);
#3964=FACE_OUTER_BOUND('',#5477,.T.);
#3965=FACE_OUTER_BOUND('',#5478,.T.);
#3966=FACE_OUTER_BOUND('',#5479,.T.);
#3967=FACE_OUTER_BOUND('',#5480,.T.);
#3968=FACE_OUTER_BOUND('',#5482,.T.);
#3969=FACE_OUTER_BOUND('',#5483,.T.);
#3970=FACE_OUTER_BOUND('',#5485,.T.);
#3971=FACE_OUTER_BOUND('',#5486,.T.);
#3972=FACE_OUTER_BOUND('',#5487,.T.);
#3973=FACE_OUTER_BOUND('',#5489,.T.);
#5425=EDGE_LOOP('',(#21008,#21009,#21010,#21011));
#5426=EDGE_LOOP('',(#21012,#21013,#21014,#21015));
#5427=EDGE_LOOP('',(#21016,#21017,#21018,#21019));
#5428=EDGE_LOOP('',(#21020,#21021,#21022,#21023));
#5429=EDGE_LOOP('',(#21024,#21025,#21026,#21027));
#5430=EDGE_LOOP('',(#21028,#21029,#21030,#21031));
#5431=EDGE_LOOP('',(#21032,#21033,#21034,#21035));
#5432=EDGE_LOOP('',(#21036,#21037,#21038,#21039,#21040));
#5433=EDGE_LOOP('',(#21041,#21042,#21043,#21044));
#5434=EDGE_LOOP('',(#21045,#21046,#21047,#21048));
#5435=EDGE_LOOP('',(#21049,#21050,#21051,#21052));
#5436=EDGE_LOOP('',(#21053,#21054,#21055,#21056));
#5437=EDGE_LOOP('',(#21057,#21058,#21059,#21060));
#5438=EDGE_LOOP('',(#21061,#21062,#21063,#21064));
#5439=EDGE_LOOP('',(#21065,#21066,#21067,#21068));
#5440=EDGE_LOOP('',(#21069,#21070,#21071,#21072));
#5441=EDGE_LOOP('',(#21073,#21074,#21075,#21076));
#5442=EDGE_LOOP('',(#21077,#21078,#21079,#21080));
#5443=EDGE_LOOP('',(#21081,#21082,#21083,#21084));
#5444=EDGE_LOOP('',(#21085,#21086,#21087,#21088));
#5445=EDGE_LOOP('',(#21089,#21090,#21091,#21092));
#5446=EDGE_LOOP('',(#21093,#21094,#21095,#21096));
#5447=EDGE_LOOP('',(#21097,#21098,#21099,#21100));
#5448=EDGE_LOOP('',(#21101,#21102,#21103,#21104));
#5449=EDGE_LOOP('',(#21105,#21106,#21107,#21108));
#5450=EDGE_LOOP('',(#21109,#21110,#21111,#21112));
#5451=EDGE_LOOP('',(#21113,#21114,#21115,#21116,#21117));
#5452=EDGE_LOOP('',(#21118,#21119,#21120,#21121,#21122,#21123,#21124,#21125,
#21126,#21127,#21128,#21129,#21130,#21131,#21132,#21133,#21134,#21135,#21136,
#21137,#21138,#21139));
#5453=EDGE_LOOP('',(#21140,#21141,#21142,#21143));
#5454=EDGE_LOOP('',(#21144,#21145,#21146,#21147,#21148,#21149,#21150,#21151,
#21152,#21153,#21154,#21155,#21156,#21157,#21158,#21159,#21160,#21161,#21162,
#21163,#21164,#21165));
#5455=EDGE_LOOP('',(#21166,#21167,#21168,#21169));
#5456=EDGE_LOOP('',(#21170,#21171,#21172,#21173));
#5457=EDGE_LOOP('',(#21174,#21175,#21176,#21177));
#5458=EDGE_LOOP('',(#21178,#21179,#21180,#21181,#21182,#21183,#21184,#21185,
#21186,#21187,#21188,#21189));
#5459=EDGE_LOOP('',(#21190,#21191,#21192,#21193,#21194,#21195,#21196,#21197,
#21198,#21199));
#5460=EDGE_LOOP('',(#21200,#21201,#21202));
#5461=EDGE_LOOP('',(#21203,#21204,#21205,#21206,#21207,#21208,#21209,#21210,
#21211,#21212,#21213));
#5462=EDGE_LOOP('',(#21214,#21215,#21216,#21217));
#5463=EDGE_LOOP('',(#21218,#21219,#21220,#21221));
#5464=EDGE_LOOP('',(#21222,#21223,#21224,#21225,#21226,#21227,#21228,#21229,
#21230,#21231));
#5465=EDGE_LOOP('',(#21232,#21233,#21234,#21235));
#5466=EDGE_LOOP('',(#21236,#21237,#21238,#21239));
#5467=EDGE_LOOP('',(#21240,#21241,#21242,#21243));
#5468=EDGE_LOOP('',(#21244,#21245,#21246,#21247,#21248,#21249,#21250,#21251,
#21252,#21253));
#5469=EDGE_LOOP('',(#21254,#21255,#21256,#21257));
#5470=EDGE_LOOP('',(#21258));
#5471=EDGE_LOOP('',(#21259,#21260,#21261,#21262));
#5472=EDGE_LOOP('',(#21263));
#5473=EDGE_LOOP('',(#21264));
#5474=EDGE_LOOP('',(#21265));
#5475=EDGE_LOOP('',(#21266));
#5476=EDGE_LOOP('',(#21267,#21268,#21269,#21270));
#5477=EDGE_LOOP('',(#21271,#21272,#21273,#21274,#21275,#21276));
#5478=EDGE_LOOP('',(#21277,#21278,#21279,#21280));
#5479=EDGE_LOOP('',(#21281,#21282,#21283,#21284));
#5480=EDGE_LOOP('',(#21285));
#5481=EDGE_LOOP('',(#21286));
#5482=EDGE_LOOP('',(#21287,#21288,#21289,#21290,#21291));
#5483=EDGE_LOOP('',(#21292,#21293,#21294,#21295,#21296,#21297,#21298));
#5484=EDGE_LOOP('',(#21299));
#5485=EDGE_LOOP('',(#21300,#21301,#21302,#21303));
#5486=EDGE_LOOP('',(#21304,#21305,#21306,#21307,#21308,#21309));
#5487=EDGE_LOOP('',(#21310));
#5488=EDGE_LOOP('',(#21311));
#5489=EDGE_LOOP('',(#21312,#21313,#21314,#21315));
#6883=LINE('',#52486,#8316);
#6884=LINE('',#52514,#8317);
#6885=LINE('',#52552,#8318);
#6886=LINE('',#52590,#8319);
#6887=LINE('',#52627,#8320);
#6888=LINE('',#52664,#8321);
#6889=LINE('',#52702,#8322);
#6890=LINE('',#52740,#8323);
#6891=LINE('',#52779,#8324);
#6892=LINE('',#52812,#8325);
#6893=LINE('',#52896,#8326);
#6894=LINE('',#52986,#8327);
#6895=LINE('',#53076,#8328);
#6896=LINE('',#53160,#8329);
#6897=LINE('',#53250,#8330);
#6898=LINE('',#53340,#8331);
#6899=LINE('',#53424,#8332);
#6900=LINE('',#53514,#8333);
#6901=LINE('',#53534,#8334);
#6902=LINE('',#53572,#8335);
#6903=LINE('',#53609,#8336);
#6904=LINE('',#53646,#8337);
#6905=LINE('',#53684,#8338);
#6906=LINE('',#53721,#8339);
#6907=LINE('',#53758,#8340);
#6908=LINE('',#53796,#8341);
#6909=LINE('',#59007,#8342);
#6910=LINE('',#59037,#8343);
#6911=LINE('',#59042,#8344);
#6912=LINE('',#59045,#8345);
#6913=LINE('',#59051,#8346);
#6914=LINE('',#59065,#8347);
#6915=LINE('',#59075,#8348);
#6916=LINE('',#59087,#8349);
#6917=LINE('',#59091,#8350);
#6918=LINE('',#59096,#8351);
#6919=LINE('',#59101,#8352);
#6920=LINE('',#59106,#8353);
#6921=LINE('',#59110,#8354);
#6922=LINE('',#59115,#8355);
#8316=VECTOR('',#30415,0.7475);
#8317=VECTOR('',#30420,0.7475);
#8318=VECTOR('',#30423,0.7475);
#8319=VECTOR('',#30426,0.7475);
#8320=VECTOR('',#30429,0.7475);
#8321=VECTOR('',#30432,0.7475);
#8322=VECTOR('',#30435,0.7475);
#8323=VECTOR('',#30438,0.7475);
#8324=VECTOR('',#30443,0.8);
#8325=VECTOR('',#30448,0.8);
#8326=VECTOR('',#30451,0.8);
#8327=VECTOR('',#30454,0.8);
#8328=VECTOR('',#30457,0.8);
#8329=VECTOR('',#30460,0.8);
#8330=VECTOR('',#30463,0.8);
#8331=VECTOR('',#30466,0.8);
#8332=VECTOR('',#30469,0.8);
#8333=VECTOR('',#30472,0.70685);
#8334=VECTOR('',#30477,0.70685);
#8335=VECTOR('',#30480,0.70685);
#8336=VECTOR('',#30483,0.70685);
#8337=VECTOR('',#30486,0.70685);
#8338=VECTOR('',#30489,0.70685);
#8339=VECTOR('',#30492,0.70685);
#8340=VECTOR('',#30495,0.70685);
#8341=VECTOR('',#30498,0.70685);
#8342=VECTOR('',#30527,1.18258529610859);
#8343=VECTOR('',#30530,1.);
#8344=VECTOR('',#30531,1.);
#8345=VECTOR('',#30534,1.);
#8346=VECTOR('',#30537,1.);
#8347=VECTOR('',#30540,1.18258529610859);
#8348=VECTOR('',#30545,1.);
#8349=VECTOR('',#30562,1.);
#8350=VECTOR('',#30567,0.4);
#8351=VECTOR('',#30574,0.4);
#8352=VECTOR('',#30581,0.7931);
#8353=VECTOR('',#30588,0.7431);
#8354=VECTOR('',#30593,0.77);
#8355=VECTOR('',#30600,0.49);
#9170=CIRCLE('',#24998,0.7475);
#9171=CIRCLE('',#25006,0.7475);
#9172=CIRCLE('',#25008,0.7925);
#9173=CIRCLE('',#25018,0.70685);
#9174=CIRCLE('',#25028,0.7925);
#9175=CIRCLE('',#25029,0.7925);
#9176=CIRCLE('',#25031,0.70685);
#9177=CIRCLE('',#25033,0.7925);
#9178=CIRCLE('',#25035,0.82685);
#9179=CIRCLE('',#25036,0.82685);
#9180=CIRCLE('',#25037,0.7475);
#9181=CIRCLE('',#25040,1.045);
#9182=CIRCLE('',#25045,1.045);
#9183=CIRCLE('',#25049,0.4);
#9184=CIRCLE('',#25051,0.7431);
#9185=CIRCLE('',#25053,0.4);
#9186=CIRCLE('',#25057,0.4);
#9187=CIRCLE('',#25059,0.4);
#9188=CIRCLE('',#25061,0.7531);
#9189=CIRCLE('',#25064,0.7431);
#9190=CIRCLE('',#25067,0.74);
#9191=CIRCLE('',#25069,0.58);
#11234=VERTEX_POINT('',#52484);
#11235=VERTEX_POINT('',#52485);
#11236=VERTEX_POINT('',#52487);
#11237=VERTEX_POINT('',#52499);
#11238=VERTEX_POINT('',#52512);
#11239=VERTEX_POINT('',#52513);
#11240=VERTEX_POINT('',#52550);
#11241=VERTEX_POINT('',#52551);
#11242=VERTEX_POINT('',#52588);
#11243=VERTEX_POINT('',#52589);
#11244=VERTEX_POINT('',#52625);
#11245=VERTEX_POINT('',#52626);
#11246=VERTEX_POINT('',#52662);
#11247=VERTEX_POINT('',#52663);
#11248=VERTEX_POINT('',#52700);
#11249=VERTEX_POINT('',#52701);
#11250=VERTEX_POINT('',#52738);
#11251=VERTEX_POINT('',#52739);
#11252=VERTEX_POINT('',#52741);
#11253=VERTEX_POINT('',#52777);
#11254=VERTEX_POINT('',#52778);
#11255=VERTEX_POINT('',#52780);
#11256=VERTEX_POINT('',#52797);
#11257=VERTEX_POINT('',#52810);
#11258=VERTEX_POINT('',#52811);
#11259=VERTEX_POINT('',#52894);
#11260=VERTEX_POINT('',#52895);
#11261=VERTEX_POINT('',#52984);
#11262=VERTEX_POINT('',#52985);
#11263=VERTEX_POINT('',#53074);
#11264=VERTEX_POINT('',#53075);
#11265=VERTEX_POINT('',#53158);
#11266=VERTEX_POINT('',#53159);
#11267=VERTEX_POINT('',#53248);
#11268=VERTEX_POINT('',#53249);
#11269=VERTEX_POINT('',#53338);
#11270=VERTEX_POINT('',#53339);
#11271=VERTEX_POINT('',#53422);
#11272=VERTEX_POINT('',#53423);
#11273=VERTEX_POINT('',#53512);
#11274=VERTEX_POINT('',#53513);
#11275=VERTEX_POINT('',#53515);
#11276=VERTEX_POINT('',#53524);
#11277=VERTEX_POINT('',#53532);
#11278=VERTEX_POINT('',#53533);
#11279=VERTEX_POINT('',#53570);
#11280=VERTEX_POINT('',#53571);
#11281=VERTEX_POINT('',#53607);
#11282=VERTEX_POINT('',#53608);
#11283=VERTEX_POINT('',#53644);
#11284=VERTEX_POINT('',#53645);
#11285=VERTEX_POINT('',#53682);
#11286=VERTEX_POINT('',#53683);
#11287=VERTEX_POINT('',#53719);
#11288=VERTEX_POINT('',#53720);
#11289=VERTEX_POINT('',#53756);
#11290=VERTEX_POINT('',#53757);
#11291=VERTEX_POINT('',#53794);
#11292=VERTEX_POINT('',#53795);
#11293=VERTEX_POINT('',#53831);
#11294=VERTEX_POINT('',#53908);
#11295=VERTEX_POINT('',#53910);
#11296=VERTEX_POINT('',#54506);
#11297=VERTEX_POINT('',#54598);
#11298=VERTEX_POINT('',#55707);
#11299=VERTEX_POINT('',#55708);
#11300=VERTEX_POINT('',#55717);
#11301=VERTEX_POINT('',#56010);
#11302=VERTEX_POINT('',#56523);
#11303=VERTEX_POINT('',#56576);
#11304=VERTEX_POINT('',#57238);
#11305=VERTEX_POINT('',#57252);
#11306=VERTEX_POINT('',#57255);
#11307=VERTEX_POINT('',#57264);
#11308=VERTEX_POINT('',#57827);
#11309=VERTEX_POINT('',#58338);
#11310=VERTEX_POINT('',#59004);
#11311=VERTEX_POINT('',#59006);
#11312=VERTEX_POINT('',#59008);
#11313=VERTEX_POINT('',#59012);
#11314=VERTEX_POINT('',#59016);
#11315=VERTEX_POINT('',#59020);
#11316=VERTEX_POINT('',#59024);
#11317=VERTEX_POINT('',#59028);
#11318=VERTEX_POINT('',#59036);
#11319=VERTEX_POINT('',#59038);
#11320=VERTEX_POINT('',#59044);
#11321=VERTEX_POINT('',#59050);
#11322=VERTEX_POINT('',#59056);
#11323=VERTEX_POINT('',#59060);
#11324=VERTEX_POINT('',#59064);
#11325=VERTEX_POINT('',#59067);
#11326=VERTEX_POINT('',#59078);
#11327=VERTEX_POINT('',#59081);
#11328=VERTEX_POINT('',#59084);
#11329=VERTEX_POINT('',#59090);
#11330=VERTEX_POINT('',#59094);
#11331=VERTEX_POINT('',#59098);
#11332=VERTEX_POINT('',#59103);
#11333=VERTEX_POINT('',#59108);
#11334=VERTEX_POINT('',#59112);
#14508=EDGE_CURVE('',#11234,#11235,#6883,.T.);
#14509=EDGE_CURVE('',#11234,#11236,#1374,.T.);
#14510=EDGE_CURVE('',#11237,#11236,#9170,.T.);
#14511=EDGE_CURVE('',#11235,#11237,#1375,.T.);
#14512=EDGE_CURVE('',#11238,#11239,#6884,.T.);
#14513=EDGE_CURVE('',#11238,#11234,#1376,.T.);
#14514=EDGE_CURVE('',#11239,#11235,#1377,.T.);
#14515=EDGE_CURVE('',#11240,#11241,#6885,.T.);
#14516=EDGE_CURVE('',#11240,#11238,#1378,.T.);
#14517=EDGE_CURVE('',#11241,#11239,#1379,.T.);
#14518=EDGE_CURVE('',#11242,#11243,#6886,.T.);
#14519=EDGE_CURVE('',#11242,#11240,#1380,.T.);
#14520=EDGE_CURVE('',#11243,#11241,#1381,.T.);
#14521=EDGE_CURVE('',#11244,#11245,#6887,.T.);
#14522=EDGE_CURVE('',#11244,#11242,#1382,.T.);
#14523=EDGE_CURVE('',#11245,#11243,#1383,.T.);
#14524=EDGE_CURVE('',#11246,#11247,#6888,.T.);
#14525=EDGE_CURVE('',#11246,#11244,#1384,.T.);
#14526=EDGE_CURVE('',#11247,#11245,#1385,.T.);
#14527=EDGE_CURVE('',#11248,#11249,#6889,.T.);
#14528=EDGE_CURVE('',#11248,#11246,#1386,.T.);
#14529=EDGE_CURVE('',#11249,#11247,#1387,.T.);
#14530=EDGE_CURVE('',#11250,#11251,#6890,.T.);
#14531=EDGE_CURVE('',#11252,#11250,#9171,.T.);
#14532=EDGE_CURVE('',#11252,#11248,#1388,.T.);
#14533=EDGE_CURVE('',#11251,#11249,#1389,.T.);
#14534=EDGE_CURVE('',#11253,#11254,#6891,.T.);
#14535=EDGE_CURVE('',#11253,#11255,#1390,.T.);
#14536=EDGE_CURVE('',#11255,#11256,#9172,.F.);
#14537=EDGE_CURVE('',#11256,#11254,#1391,.T.);
#14538=EDGE_CURVE('',#11257,#11258,#6892,.T.);
#14539=EDGE_CURVE('',#11257,#11253,#1392,.T.);
#14540=EDGE_CURVE('',#11254,#11258,#1393,.T.);
#14541=EDGE_CURVE('',#11259,#11260,#6893,.T.);
#14542=EDGE_CURVE('',#11259,#11257,#1394,.T.);
#14543=EDGE_CURVE('',#11258,#11260,#1395,.T.);
#14544=EDGE_CURVE('',#11261,#11262,#6894,.T.);
#14545=EDGE_CURVE('',#11261,#11259,#1396,.T.);
#14546=EDGE_CURVE('',#11260,#11262,#1397,.T.);
#14547=EDGE_CURVE('',#11263,#11264,#6895,.T.);
#14548=EDGE_CURVE('',#11263,#11261,#1398,.T.);
#14549=EDGE_CURVE('',#11262,#11264,#1399,.T.);
#14550=EDGE_CURVE('',#11265,#11266,#6896,.T.);
#14551=EDGE_CURVE('',#11265,#11263,#1400,.T.);
#14552=EDGE_CURVE('',#11264,#11266,#1401,.T.);
#14553=EDGE_CURVE('',#11267,#11268,#6897,.T.);
#14554=EDGE_CURVE('',#11267,#11265,#1402,.T.);
#14555=EDGE_CURVE('',#11266,#11268,#1403,.T.);
#14556=EDGE_CURVE('',#11269,#11270,#6898,.T.);
#14557=EDGE_CURVE('',#11269,#11267,#1404,.T.);
#14558=EDGE_CURVE('',#11268,#11270,#1405,.T.);
#14559=EDGE_CURVE('',#11271,#11272,#6899,.T.);
#14560=EDGE_CURVE('',#11271,#11269,#1406,.T.);
#14561=EDGE_CURVE('',#11270,#11272,#1407,.T.);
#14562=EDGE_CURVE('',#11273,#11274,#6900,.T.);
#14563=EDGE_CURVE('',#11273,#11275,#1408,.T.);
#14564=EDGE_CURVE('',#11276,#11275,#9173,.T.);
#14565=EDGE_CURVE('',#11274,#11276,#1409,.T.);
#14566=EDGE_CURVE('',#11277,#11278,#6901,.T.);
#14567=EDGE_CURVE('',#11277,#11273,#1410,.T.);
#14568=EDGE_CURVE('',#11278,#11274,#1411,.T.);
#14569=EDGE_CURVE('',#11279,#11280,#6902,.T.);
#14570=EDGE_CURVE('',#11279,#11277,#1412,.T.);
#14571=EDGE_CURVE('',#11280,#11278,#1413,.T.);
#14572=EDGE_CURVE('',#11281,#11282,#6903,.T.);
#14573=EDGE_CURVE('',#11281,#11279,#1414,.T.);
#14574=EDGE_CURVE('',#11282,#11280,#1415,.T.);
#14575=EDGE_CURVE('',#11283,#11284,#6904,.T.);
#14576=EDGE_CURVE('',#11283,#11281,#1416,.T.);
#14577=EDGE_CURVE('',#11284,#11282,#1417,.T.);
#14578=EDGE_CURVE('',#11285,#11286,#6905,.T.);
#14579=EDGE_CURVE('',#11285,#11283,#1418,.T.);
#14580=EDGE_CURVE('',#11286,#11284,#1419,.T.);
#14581=EDGE_CURVE('',#11287,#11288,#6906,.T.);
#14582=EDGE_CURVE('',#11287,#11285,#1420,.T.);
#14583=EDGE_CURVE('',#11288,#11286,#1421,.T.);
#14584=EDGE_CURVE('',#11289,#11290,#6907,.T.);
#14585=EDGE_CURVE('',#11289,#11287,#1422,.T.);
#14586=EDGE_CURVE('',#11290,#11288,#1423,.T.);
#14587=EDGE_CURVE('',#11291,#11292,#6908,.T.);
#14588=EDGE_CURVE('',#11291,#11289,#1424,.T.);
#14589=EDGE_CURVE('',#11292,#11290,#1425,.T.);
#14590=EDGE_CURVE('',#11275,#11293,#1426,.T.);
#14591=EDGE_CURVE('',#11294,#11293,#9174,.F.);
#14592=EDGE_CURVE('',#11295,#11294,#9175,.F.);
#14593=EDGE_CURVE('',#11295,#11276,#1427,.T.);
#14594=EDGE_CURVE('',#11272,#11295,#1428,.T.);
#14595=EDGE_CURVE('',#11296,#11256,#1429,.T.);
#14596=EDGE_CURVE('',#11296,#11292,#1430,.T.);
#14597=EDGE_CURVE('',#11297,#11296,#9176,.T.);
#14598=EDGE_CURVE('',#11297,#11291,#1431,.T.);
#14599=EDGE_CURVE('',#11255,#11297,#1432,.T.);
#14600=EDGE_CURVE('',#11293,#11271,#1433,.T.);
#14601=EDGE_CURVE('',#11293,#11295,#9177,.F.);
#14602=EDGE_CURVE('',#11298,#11299,#1434,.T.);
#14603=EDGE_CURVE('',#11300,#11298,#1435,.T.);
#14604=EDGE_CURVE('',#11301,#11300,#1436,.T.);
#14605=EDGE_CURVE('',#11301,#11299,#1437,.T.);
#14606=EDGE_CURVE('',#11299,#11302,#1438,.T.);
#14607=EDGE_CURVE('',#11303,#11301,#1439,.T.);
#14608=EDGE_CURVE('',#11303,#11302,#1440,.T.);
#14609=EDGE_CURVE('',#11302,#11237,#1441,.T.);
#14610=EDGE_CURVE('',#11304,#11303,#1442,.T.);
#14611=EDGE_CURVE('',#11304,#11251,#1443,.T.);
#14612=EDGE_CURVE('',#11300,#11305,#9178,.T.);
#14613=EDGE_CURVE('',#11305,#11300,#9179,.T.);
#14614=EDGE_CURVE('',#11300,#11306,#1444,.T.);
#14615=EDGE_CURVE('',#11306,#11307,#1445,.T.);
#14616=EDGE_CURVE('',#11307,#11252,#1446,.T.);
#14617=EDGE_CURVE('',#11250,#11304,#9180,.T.);
#14618=EDGE_CURVE('',#11236,#11308,#1447,.T.);
#14619=EDGE_CURVE('',#11307,#11308,#1448,.T.);
#14620=EDGE_CURVE('',#11308,#11309,#1449,.T.);
#14621=EDGE_CURVE('',#11306,#11309,#1450,.T.);
#14622=EDGE_CURVE('',#11309,#11298,#1451,.T.);
#14623=EDGE_CURVE('',#11310,#11310,#9181,.T.);
#14624=EDGE_CURVE('',#11310,#11311,#6909,.T.);
#14625=EDGE_CURVE('',#11312,#11311,#1494,.T.);
#14626=EDGE_CURVE('',#11313,#11312,#1495,.T.);
#14627=EDGE_CURVE('',#11314,#11313,#1496,.T.);
#14628=EDGE_CURVE('',#11315,#11314,#1497,.T.);
#14629=EDGE_CURVE('',#11316,#11315,#1498,.T.);
#14630=EDGE_CURVE('',#11317,#11316,#1499,.T.);
#14631=EDGE_CURVE('',#11311,#11317,#1500,.T.);
#14632=EDGE_CURVE('',#11315,#11318,#6910,.T.);
#14633=EDGE_CURVE('',#11318,#11319,#1501,.T.);
#14634=EDGE_CURVE('',#11316,#11319,#6911,.T.);
#14635=EDGE_CURVE('',#11314,#11320,#6912,.T.);
#14636=EDGE_CURVE('',#11320,#11318,#1502,.T.);
#14637=EDGE_CURVE('',#11313,#11321,#6913,.T.);
#14638=EDGE_CURVE('',#11321,#11320,#1503,.T.);
#14639=EDGE_CURVE('',#11322,#11321,#1504,.T.);
#14640=EDGE_CURVE('',#11323,#11322,#1505,.T.);
#14641=EDGE_CURVE('',#11323,#11324,#6914,.T.);
#14642=EDGE_CURVE('',#11324,#11324,#9182,.T.);
#14643=EDGE_CURVE('',#11325,#11323,#1506,.T.);
#14644=EDGE_CURVE('',#11319,#11325,#1507,.T.);
#14645=EDGE_CURVE('',#11312,#11322,#6915,.T.);
#14646=EDGE_CURVE('',#11326,#11326,#9183,.T.);
#14647=EDGE_CURVE('',#11327,#11327,#9184,.T.);
#14648=EDGE_CURVE('',#11328,#11328,#9185,.T.);
#14649=EDGE_CURVE('',#11317,#11325,#6916,.T.);
#14650=EDGE_CURVE('',#11328,#11329,#6917,.T.);
#14651=EDGE_CURVE('',#11329,#11329,#9186,.T.);
#14652=EDGE_CURVE('',#11330,#11330,#9187,.T.);
#14653=EDGE_CURVE('',#11330,#11326,#6918,.T.);
#14654=EDGE_CURVE('',#11331,#11331,#9188,.T.);
#14655=EDGE_CURVE('',#11305,#11331,#6919,.T.);
#14656=EDGE_CURVE('',#11332,#11332,#9189,.T.);
#14657=EDGE_CURVE('',#11327,#11332,#6920,.T.);
#14658=EDGE_CURVE('',#11333,#11333,#9190,.T.);
#14659=EDGE_CURVE('',#11333,#11294,#6921,.T.);
#14660=EDGE_CURVE('',#11334,#11334,#9191,.T.);
#14661=EDGE_CURVE('',#11334,#11330,#6922,.T.);
#21008=ORIENTED_EDGE('',*,*,#14508,.F.);
#21009=ORIENTED_EDGE('',*,*,#14509,.T.);
#21010=ORIENTED_EDGE('',*,*,#14510,.F.);
#21011=ORIENTED_EDGE('',*,*,#14511,.F.);
#21012=ORIENTED_EDGE('',*,*,#14512,.F.);
#21013=ORIENTED_EDGE('',*,*,#14513,.T.);
#21014=ORIENTED_EDGE('',*,*,#14508,.T.);
#21015=ORIENTED_EDGE('',*,*,#14514,.F.);
#21016=ORIENTED_EDGE('',*,*,#14515,.F.);
#21017=ORIENTED_EDGE('',*,*,#14516,.T.);
#21018=ORIENTED_EDGE('',*,*,#14512,.T.);
#21019=ORIENTED_EDGE('',*,*,#14517,.F.);
#21020=ORIENTED_EDGE('',*,*,#14518,.F.);
#21021=ORIENTED_EDGE('',*,*,#14519,.T.);
#21022=ORIENTED_EDGE('',*,*,#14515,.T.);
#21023=ORIENTED_EDGE('',*,*,#14520,.F.);
#21024=ORIENTED_EDGE('',*,*,#14521,.F.);
#21025=ORIENTED_EDGE('',*,*,#14522,.T.);
#21026=ORIENTED_EDGE('',*,*,#14518,.T.);
#21027=ORIENTED_EDGE('',*,*,#14523,.F.);
#21028=ORIENTED_EDGE('',*,*,#14524,.F.);
#21029=ORIENTED_EDGE('',*,*,#14525,.T.);
#21030=ORIENTED_EDGE('',*,*,#14521,.T.);
#21031=ORIENTED_EDGE('',*,*,#14526,.F.);
#21032=ORIENTED_EDGE('',*,*,#14527,.F.);
#21033=ORIENTED_EDGE('',*,*,#14528,.T.);
#21034=ORIENTED_EDGE('',*,*,#14524,.T.);
#21035=ORIENTED_EDGE('',*,*,#14529,.F.);
#21036=ORIENTED_EDGE('',*,*,#14530,.F.);
#21037=ORIENTED_EDGE('',*,*,#14531,.F.);
#21038=ORIENTED_EDGE('',*,*,#14532,.T.);
#21039=ORIENTED_EDGE('',*,*,#14527,.T.);
#21040=ORIENTED_EDGE('',*,*,#14533,.F.);
#21041=ORIENTED_EDGE('',*,*,#14534,.F.);
#21042=ORIENTED_EDGE('',*,*,#14535,.T.);
#21043=ORIENTED_EDGE('',*,*,#14536,.T.);
#21044=ORIENTED_EDGE('',*,*,#14537,.T.);
#21045=ORIENTED_EDGE('',*,*,#14538,.F.);
#21046=ORIENTED_EDGE('',*,*,#14539,.T.);
#21047=ORIENTED_EDGE('',*,*,#14534,.T.);
#21048=ORIENTED_EDGE('',*,*,#14540,.T.);
#21049=ORIENTED_EDGE('',*,*,#14541,.F.);
#21050=ORIENTED_EDGE('',*,*,#14542,.T.);
#21051=ORIENTED_EDGE('',*,*,#14538,.T.);
#21052=ORIENTED_EDGE('',*,*,#14543,.T.);
#21053=ORIENTED_EDGE('',*,*,#14544,.F.);
#21054=ORIENTED_EDGE('',*,*,#14545,.T.);
#21055=ORIENTED_EDGE('',*,*,#14541,.T.);
#21056=ORIENTED_EDGE('',*,*,#14546,.T.);
#21057=ORIENTED_EDGE('',*,*,#14547,.F.);
#21058=ORIENTED_EDGE('',*,*,#14548,.T.);
#21059=ORIENTED_EDGE('',*,*,#14544,.T.);
#21060=ORIENTED_EDGE('',*,*,#14549,.T.);
#21061=ORIENTED_EDGE('',*,*,#14550,.F.);
#21062=ORIENTED_EDGE('',*,*,#14551,.T.);
#21063=ORIENTED_EDGE('',*,*,#14547,.T.);
#21064=ORIENTED_EDGE('',*,*,#14552,.T.);
#21065=ORIENTED_EDGE('',*,*,#14553,.F.);
#21066=ORIENTED_EDGE('',*,*,#14554,.T.);
#21067=ORIENTED_EDGE('',*,*,#14550,.T.);
#21068=ORIENTED_EDGE('',*,*,#14555,.T.);
#21069=ORIENTED_EDGE('',*,*,#14556,.F.);
#21070=ORIENTED_EDGE('',*,*,#14557,.T.);
#21071=ORIENTED_EDGE('',*,*,#14553,.T.);
#21072=ORIENTED_EDGE('',*,*,#14558,.T.);
#21073=ORIENTED_EDGE('',*,*,#14559,.F.);
#21074=ORIENTED_EDGE('',*,*,#14560,.T.);
#21075=ORIENTED_EDGE('',*,*,#14556,.T.);
#21076=ORIENTED_EDGE('',*,*,#14561,.T.);
#21077=ORIENTED_EDGE('',*,*,#14562,.F.);
#21078=ORIENTED_EDGE('',*,*,#14563,.T.);
#21079=ORIENTED_EDGE('',*,*,#14564,.F.);
#21080=ORIENTED_EDGE('',*,*,#14565,.F.);
#21081=ORIENTED_EDGE('',*,*,#14566,.F.);
#21082=ORIENTED_EDGE('',*,*,#14567,.T.);
#21083=ORIENTED_EDGE('',*,*,#14562,.T.);
#21084=ORIENTED_EDGE('',*,*,#14568,.F.);
#21085=ORIENTED_EDGE('',*,*,#14569,.F.);
#21086=ORIENTED_EDGE('',*,*,#14570,.T.);
#21087=ORIENTED_EDGE('',*,*,#14566,.T.);
#21088=ORIENTED_EDGE('',*,*,#14571,.F.);
#21089=ORIENTED_EDGE('',*,*,#14572,.F.);
#21090=ORIENTED_EDGE('',*,*,#14573,.T.);
#21091=ORIENTED_EDGE('',*,*,#14569,.T.);
#21092=ORIENTED_EDGE('',*,*,#14574,.F.);
#21093=ORIENTED_EDGE('',*,*,#14575,.F.);
#21094=ORIENTED_EDGE('',*,*,#14576,.T.);
#21095=ORIENTED_EDGE('',*,*,#14572,.T.);
#21096=ORIENTED_EDGE('',*,*,#14577,.F.);
#21097=ORIENTED_EDGE('',*,*,#14578,.F.);
#21098=ORIENTED_EDGE('',*,*,#14579,.T.);
#21099=ORIENTED_EDGE('',*,*,#14575,.T.);
#21100=ORIENTED_EDGE('',*,*,#14580,.F.);
#21101=ORIENTED_EDGE('',*,*,#14581,.F.);
#21102=ORIENTED_EDGE('',*,*,#14582,.T.);
#21103=ORIENTED_EDGE('',*,*,#14578,.T.);
#21104=ORIENTED_EDGE('',*,*,#14583,.F.);
#21105=ORIENTED_EDGE('',*,*,#14584,.F.);
#21106=ORIENTED_EDGE('',*,*,#14585,.T.);
#21107=ORIENTED_EDGE('',*,*,#14581,.T.);
#21108=ORIENTED_EDGE('',*,*,#14586,.F.);
#21109=ORIENTED_EDGE('',*,*,#14587,.F.);
#21110=ORIENTED_EDGE('',*,*,#14588,.T.);
#21111=ORIENTED_EDGE('',*,*,#14584,.T.);
#21112=ORIENTED_EDGE('',*,*,#14589,.F.);
#21113=ORIENTED_EDGE('',*,*,#14564,.T.);
#21114=ORIENTED_EDGE('',*,*,#14590,.T.);
#21115=ORIENTED_EDGE('',*,*,#14591,.F.);
#21116=ORIENTED_EDGE('',*,*,#14592,.F.);
#21117=ORIENTED_EDGE('',*,*,#14593,.T.);
#21118=ORIENTED_EDGE('',*,*,#14593,.F.);
#21119=ORIENTED_EDGE('',*,*,#14594,.F.);
#21120=ORIENTED_EDGE('',*,*,#14561,.F.);
#21121=ORIENTED_EDGE('',*,*,#14558,.F.);
#21122=ORIENTED_EDGE('',*,*,#14555,.F.);
#21123=ORIENTED_EDGE('',*,*,#14552,.F.);
#21124=ORIENTED_EDGE('',*,*,#14549,.F.);
#21125=ORIENTED_EDGE('',*,*,#14546,.F.);
#21126=ORIENTED_EDGE('',*,*,#14543,.F.);
#21127=ORIENTED_EDGE('',*,*,#14540,.F.);
#21128=ORIENTED_EDGE('',*,*,#14537,.F.);
#21129=ORIENTED_EDGE('',*,*,#14595,.F.);
#21130=ORIENTED_EDGE('',*,*,#14596,.T.);
#21131=ORIENTED_EDGE('',*,*,#14589,.T.);
#21132=ORIENTED_EDGE('',*,*,#14586,.T.);
#21133=ORIENTED_EDGE('',*,*,#14583,.T.);
#21134=ORIENTED_EDGE('',*,*,#14580,.T.);
#21135=ORIENTED_EDGE('',*,*,#14577,.T.);
#21136=ORIENTED_EDGE('',*,*,#14574,.T.);
#21137=ORIENTED_EDGE('',*,*,#14571,.T.);
#21138=ORIENTED_EDGE('',*,*,#14568,.T.);
#21139=ORIENTED_EDGE('',*,*,#14565,.T.);
#21140=ORIENTED_EDGE('',*,*,#14587,.T.);
#21141=ORIENTED_EDGE('',*,*,#14596,.F.);
#21142=ORIENTED_EDGE('',*,*,#14597,.F.);
#21143=ORIENTED_EDGE('',*,*,#14598,.T.);
#21144=ORIENTED_EDGE('',*,*,#14590,.F.);
#21145=ORIENTED_EDGE('',*,*,#14563,.F.);
#21146=ORIENTED_EDGE('',*,*,#14567,.F.);
#21147=ORIENTED_EDGE('',*,*,#14570,.F.);
#21148=ORIENTED_EDGE('',*,*,#14573,.F.);
#21149=ORIENTED_EDGE('',*,*,#14576,.F.);
#21150=ORIENTED_EDGE('',*,*,#14579,.F.);
#21151=ORIENTED_EDGE('',*,*,#14582,.F.);
#21152=ORIENTED_EDGE('',*,*,#14585,.F.);
#21153=ORIENTED_EDGE('',*,*,#14588,.F.);
#21154=ORIENTED_EDGE('',*,*,#14598,.F.);
#21155=ORIENTED_EDGE('',*,*,#14599,.F.);
#21156=ORIENTED_EDGE('',*,*,#14535,.F.);
#21157=ORIENTED_EDGE('',*,*,#14539,.F.);
#21158=ORIENTED_EDGE('',*,*,#14542,.F.);
#21159=ORIENTED_EDGE('',*,*,#14545,.F.);
#21160=ORIENTED_EDGE('',*,*,#14548,.F.);
#21161=ORIENTED_EDGE('',*,*,#14551,.F.);
#21162=ORIENTED_EDGE('',*,*,#14554,.F.);
#21163=ORIENTED_EDGE('',*,*,#14557,.F.);
#21164=ORIENTED_EDGE('',*,*,#14560,.F.);
#21165=ORIENTED_EDGE('',*,*,#14600,.F.);
#21166=ORIENTED_EDGE('',*,*,#14559,.T.);
#21167=ORIENTED_EDGE('',*,*,#14594,.T.);
#21168=ORIENTED_EDGE('',*,*,#14601,.F.);
#21169=ORIENTED_EDGE('',*,*,#14600,.T.);
#21170=ORIENTED_EDGE('',*,*,#14602,.F.);
#21171=ORIENTED_EDGE('',*,*,#14603,.F.);
#21172=ORIENTED_EDGE('',*,*,#14604,.F.);
#21173=ORIENTED_EDGE('',*,*,#14605,.T.);
#21174=ORIENTED_EDGE('',*,*,#14606,.F.);
#21175=ORIENTED_EDGE('',*,*,#14605,.F.);
#21176=ORIENTED_EDGE('',*,*,#14607,.F.);
#21177=ORIENTED_EDGE('',*,*,#14608,.T.);
#21178=ORIENTED_EDGE('',*,*,#14609,.F.);
#21179=ORIENTED_EDGE('',*,*,#14608,.F.);
#21180=ORIENTED_EDGE('',*,*,#14610,.F.);
#21181=ORIENTED_EDGE('',*,*,#14611,.T.);
#21182=ORIENTED_EDGE('',*,*,#14533,.T.);
#21183=ORIENTED_EDGE('',*,*,#14529,.T.);
#21184=ORIENTED_EDGE('',*,*,#14526,.T.);
#21185=ORIENTED_EDGE('',*,*,#14523,.T.);
#21186=ORIENTED_EDGE('',*,*,#14520,.T.);
#21187=ORIENTED_EDGE('',*,*,#14517,.T.);
#21188=ORIENTED_EDGE('',*,*,#14514,.T.);
#21189=ORIENTED_EDGE('',*,*,#14511,.T.);
#21190=ORIENTED_EDGE('',*,*,#14612,.T.);
#21191=ORIENTED_EDGE('',*,*,#14613,.T.);
#21192=ORIENTED_EDGE('',*,*,#14614,.T.);
#21193=ORIENTED_EDGE('',*,*,#14615,.T.);
#21194=ORIENTED_EDGE('',*,*,#14616,.T.);
#21195=ORIENTED_EDGE('',*,*,#14531,.T.);
#21196=ORIENTED_EDGE('',*,*,#14617,.T.);
#21197=ORIENTED_EDGE('',*,*,#14610,.T.);
#21198=ORIENTED_EDGE('',*,*,#14607,.T.);
#21199=ORIENTED_EDGE('',*,*,#14604,.T.);
#21200=ORIENTED_EDGE('',*,*,#14530,.T.);
#21201=ORIENTED_EDGE('',*,*,#14611,.F.);
#21202=ORIENTED_EDGE('',*,*,#14617,.F.);
#21203=ORIENTED_EDGE('',*,*,#14618,.F.);
#21204=ORIENTED_EDGE('',*,*,#14509,.F.);
#21205=ORIENTED_EDGE('',*,*,#14513,.F.);
#21206=ORIENTED_EDGE('',*,*,#14516,.F.);
#21207=ORIENTED_EDGE('',*,*,#14519,.F.);
#21208=ORIENTED_EDGE('',*,*,#14522,.F.);
#21209=ORIENTED_EDGE('',*,*,#14525,.F.);
#21210=ORIENTED_EDGE('',*,*,#14528,.F.);
#21211=ORIENTED_EDGE('',*,*,#14532,.F.);
#21212=ORIENTED_EDGE('',*,*,#14616,.F.);
#21213=ORIENTED_EDGE('',*,*,#14619,.T.);
#21214=ORIENTED_EDGE('',*,*,#14620,.F.);
#21215=ORIENTED_EDGE('',*,*,#14619,.F.);
#21216=ORIENTED_EDGE('',*,*,#14615,.F.);
#21217=ORIENTED_EDGE('',*,*,#14621,.T.);
#21218=ORIENTED_EDGE('',*,*,#14622,.F.);
#21219=ORIENTED_EDGE('',*,*,#14621,.F.);
#21220=ORIENTED_EDGE('',*,*,#14614,.F.);
#21221=ORIENTED_EDGE('',*,*,#14603,.T.);
#21222=ORIENTED_EDGE('',*,*,#14623,.F.);
#21223=ORIENTED_EDGE('',*,*,#14624,.T.);
#21224=ORIENTED_EDGE('',*,*,#14625,.F.);
#21225=ORIENTED_EDGE('',*,*,#14626,.F.);
#21226=ORIENTED_EDGE('',*,*,#14627,.F.);
#21227=ORIENTED_EDGE('',*,*,#14628,.F.);
#21228=ORIENTED_EDGE('',*,*,#14629,.F.);
#21229=ORIENTED_EDGE('',*,*,#14630,.F.);
#21230=ORIENTED_EDGE('',*,*,#14631,.F.);
#21231=ORIENTED_EDGE('',*,*,#14624,.F.);
#21232=ORIENTED_EDGE('',*,*,#14629,.T.);
#21233=ORIENTED_EDGE('',*,*,#14632,.T.);
#21234=ORIENTED_EDGE('',*,*,#14633,.T.);
#21235=ORIENTED_EDGE('',*,*,#14634,.F.);
#21236=ORIENTED_EDGE('',*,*,#14628,.T.);
#21237=ORIENTED_EDGE('',*,*,#14635,.T.);
#21238=ORIENTED_EDGE('',*,*,#14636,.T.);
#21239=ORIENTED_EDGE('',*,*,#14632,.F.);
#21240=ORIENTED_EDGE('',*,*,#14627,.T.);
#21241=ORIENTED_EDGE('',*,*,#14637,.T.);
#21242=ORIENTED_EDGE('',*,*,#14638,.T.);
#21243=ORIENTED_EDGE('',*,*,#14635,.F.);
#21244=ORIENTED_EDGE('',*,*,#14633,.F.);
#21245=ORIENTED_EDGE('',*,*,#14636,.F.);
#21246=ORIENTED_EDGE('',*,*,#14638,.F.);
#21247=ORIENTED_EDGE('',*,*,#14639,.F.);
#21248=ORIENTED_EDGE('',*,*,#14640,.F.);
#21249=ORIENTED_EDGE('',*,*,#14641,.T.);
#21250=ORIENTED_EDGE('',*,*,#14642,.F.);
#21251=ORIENTED_EDGE('',*,*,#14641,.F.);
#21252=ORIENTED_EDGE('',*,*,#14643,.F.);
#21253=ORIENTED_EDGE('',*,*,#14644,.F.);
#21254=ORIENTED_EDGE('',*,*,#14626,.T.);
#21255=ORIENTED_EDGE('',*,*,#14645,.T.);
#21256=ORIENTED_EDGE('',*,*,#14639,.T.);
#21257=ORIENTED_EDGE('',*,*,#14637,.F.);
#21258=ORIENTED_EDGE('',*,*,#14642,.T.);
#21259=ORIENTED_EDGE('',*,*,#14599,.T.);
#21260=ORIENTED_EDGE('',*,*,#14597,.T.);
#21261=ORIENTED_EDGE('',*,*,#14595,.T.);
#21262=ORIENTED_EDGE('',*,*,#14536,.F.);
#21263=ORIENTED_EDGE('',*,*,#14646,.F.);
#21264=ORIENTED_EDGE('',*,*,#14623,.T.);
#21265=ORIENTED_EDGE('',*,*,#14647,.F.);
#21266=ORIENTED_EDGE('',*,*,#14648,.F.);
#21267=ORIENTED_EDGE('',*,*,#14630,.T.);
#21268=ORIENTED_EDGE('',*,*,#14634,.T.);
#21269=ORIENTED_EDGE('',*,*,#14644,.T.);
#21270=ORIENTED_EDGE('',*,*,#14649,.F.);
#21271=ORIENTED_EDGE('',*,*,#14625,.T.);
#21272=ORIENTED_EDGE('',*,*,#14631,.T.);
#21273=ORIENTED_EDGE('',*,*,#14649,.T.);
#21274=ORIENTED_EDGE('',*,*,#14643,.T.);
#21275=ORIENTED_EDGE('',*,*,#14640,.T.);
#21276=ORIENTED_EDGE('',*,*,#14645,.F.);
#21277=ORIENTED_EDGE('',*,*,#14648,.T.);
#21278=ORIENTED_EDGE('',*,*,#14650,.T.);
#21279=ORIENTED_EDGE('',*,*,#14651,.F.);
#21280=ORIENTED_EDGE('',*,*,#14650,.F.);
#21281=ORIENTED_EDGE('',*,*,#14652,.T.);
#21282=ORIENTED_EDGE('',*,*,#14653,.T.);
#21283=ORIENTED_EDGE('',*,*,#14646,.T.);
#21284=ORIENTED_EDGE('',*,*,#14653,.F.);
#21285=ORIENTED_EDGE('',*,*,#14654,.F.);
#21286=ORIENTED_EDGE('',*,*,#14651,.T.);
#21287=ORIENTED_EDGE('',*,*,#14612,.F.);
#21288=ORIENTED_EDGE('',*,*,#14613,.F.);
#21289=ORIENTED_EDGE('',*,*,#14655,.T.);
#21290=ORIENTED_EDGE('',*,*,#14654,.T.);
#21291=ORIENTED_EDGE('',*,*,#14655,.F.);
#21292=ORIENTED_EDGE('',*,*,#14602,.T.);
#21293=ORIENTED_EDGE('',*,*,#14606,.T.);
#21294=ORIENTED_EDGE('',*,*,#14609,.T.);
#21295=ORIENTED_EDGE('',*,*,#14510,.T.);
#21296=ORIENTED_EDGE('',*,*,#14618,.T.);
#21297=ORIENTED_EDGE('',*,*,#14620,.T.);
#21298=ORIENTED_EDGE('',*,*,#14622,.T.);
#21299=ORIENTED_EDGE('',*,*,#14656,.F.);
#21300=ORIENTED_EDGE('',*,*,#14647,.T.);
#21301=ORIENTED_EDGE('',*,*,#14657,.T.);
#21302=ORIENTED_EDGE('',*,*,#14656,.T.);
#21303=ORIENTED_EDGE('',*,*,#14657,.F.);
#21304=ORIENTED_EDGE('',*,*,#14658,.F.);
#21305=ORIENTED_EDGE('',*,*,#14659,.T.);
#21306=ORIENTED_EDGE('',*,*,#14591,.T.);
#21307=ORIENTED_EDGE('',*,*,#14601,.T.);
#21308=ORIENTED_EDGE('',*,*,#14592,.T.);
#21309=ORIENTED_EDGE('',*,*,#14659,.F.);
#21310=ORIENTED_EDGE('',*,*,#14658,.T.);
#21311=ORIENTED_EDGE('',*,*,#14660,.F.);
#21312=ORIENTED_EDGE('',*,*,#14660,.T.);
#21313=ORIENTED_EDGE('',*,*,#14661,.T.);
#21314=ORIENTED_EDGE('',*,*,#14652,.F.);
#21315=ORIENTED_EDGE('',*,*,#14661,.F.);
#21494=CONICAL_SURFACE('',#25039,1.18258529610859,1.0471975511966);
#21495=CONICAL_SURFACE('',#25044,1.18258529610859,1.0471975511966);
#21496=CONICAL_SURFACE('',#25062,0.7931,0.785398163397448);
#21497=CONICAL_SURFACE('',#25066,0.77,0.785398163397445);
#21498=CONICAL_SURFACE('',#25070,0.49,0.209439510239319);
#22744=ADVANCED_FACE('',(#3914),#2637,.T.);
#22745=ADVANCED_FACE('',(#3915),#2638,.T.);
#22746=ADVANCED_FACE('',(#3916),#2639,.T.);
#22747=ADVANCED_FACE('',(#3917),#2640,.T.);
#22748=ADVANCED_FACE('',(#3918),#2641,.T.);
#22749=ADVANCED_FACE('',(#3919),#2642,.T.);
#22750=ADVANCED_FACE('',(#3920),#2643,.T.);
#22751=ADVANCED_FACE('',(#3921),#2644,.T.);
#22752=ADVANCED_FACE('',(#3922),#2645,.T.);
#22753=ADVANCED_FACE('',(#3923),#2646,.T.);
#22754=ADVANCED_FACE('',(#3924),#2647,.T.);
#22755=ADVANCED_FACE('',(#3925),#2648,.T.);
#22756=ADVANCED_FACE('',(#3926),#2649,.T.);
#22757=ADVANCED_FACE('',(#3927),#2650,.T.);
#22758=ADVANCED_FACE('',(#3928),#2651,.T.);
#22759=ADVANCED_FACE('',(#3929),#2652,.T.);
#22760=ADVANCED_FACE('',(#3930),#2653,.T.);
#22761=ADVANCED_FACE('',(#3931),#2654,.T.);
#22762=ADVANCED_FACE('',(#3932),#2655,.T.);
#22763=ADVANCED_FACE('',(#3933),#2656,.T.);
#22764=ADVANCED_FACE('',(#3934),#2657,.T.);
#22765=ADVANCED_FACE('',(#3935),#2658,.T.);
#22766=ADVANCED_FACE('',(#3936),#2659,.T.);
#22767=ADVANCED_FACE('',(#3937),#2660,.T.);
#22768=ADVANCED_FACE('',(#3938),#2661,.T.);
#22769=ADVANCED_FACE('',(#3939),#2662,.T.);
#22770=ADVANCED_FACE('',(#3940),#2394,.F.);
#22771=ADVANCED_FACE('',(#3941),#561,.F.);
#22772=ADVANCED_FACE('',(#3942),#2663,.T.);
#22773=ADVANCED_FACE('',(#3943),#562,.F.);
#22774=ADVANCED_FACE('',(#3944),#2664,.T.);
#22775=ADVANCED_FACE('',(#3945),#563,.T.);
#22776=ADVANCED_FACE('',(#3946),#564,.F.);
#22777=ADVANCED_FACE('',(#3947),#565,.F.);
#22778=ADVANCED_FACE('',(#3948),#2395,.T.);
#22779=ADVANCED_FACE('',(#3949),#2665,.T.);
#22780=ADVANCED_FACE('',(#3950),#566,.F.);
#22781=ADVANCED_FACE('',(#3951),#567,.F.);
#22782=ADVANCED_FACE('',(#3952),#568,.T.);
#22783=ADVANCED_FACE('',(#3953),#21494,.T.);
#22784=ADVANCED_FACE('',(#3954),#2396,.T.);
#22785=ADVANCED_FACE('',(#3955),#2397,.T.);
#22786=ADVANCED_FACE('',(#3956),#2398,.T.);
#22787=ADVANCED_FACE('',(#3957),#21495,.T.);
#22788=ADVANCED_FACE('',(#3958),#2399,.T.);
#22789=ADVANCED_FACE('',(#3959,#1805),#2400,.T.);
#22790=ADVANCED_FACE('',(#3960),#2401,.T.);
#22791=ADVANCED_FACE('',(#3961,#1806),#2402,.F.);
#22792=ADVANCED_FACE('',(#3962),#2403,.F.);
#22793=ADVANCED_FACE('',(#3963),#2404,.T.);
#22794=ADVANCED_FACE('',(#3964),#2405,.T.);
#22795=ADVANCED_FACE('',(#3965),#2666,.F.);
#22796=ADVANCED_FACE('',(#3966),#2667,.F.);
#22797=ADVANCED_FACE('',(#3967,#1807),#2406,.T.);
#22798=ADVANCED_FACE('',(#3968),#21496,.T.);
#22799=ADVANCED_FACE('',(#3969,#1808),#2407,.T.);
#22800=ADVANCED_FACE('',(#3970),#2668,.T.);
#22801=ADVANCED_FACE('',(#3971),#21497,.T.);
#22802=ADVANCED_FACE('',(#3972,#1809),#2408,.T.);
#22803=ADVANCED_FACE('',(#3973),#21498,.F.);
#22823=CLOSED_SHELL('',(#22744,#22745,#22746,#22747,#22748,#22749,#22750,
#22751,#22752,#22753,#22754,#22755,#22756,#22757,#22758,#22759,#22760,#22761,
#22762,#22763,#22764,#22765,#22766,#22767,#22768,#22769,#22770,#22771,#22772,
#22773,#22774,#22775,#22776,#22777,#22778,#22779,#22780,#22781,#22782,#22783,
#22784,#22785,#22786,#22787,#22788,#22789,#22790,#22791,#22792,#22793,#22794,
#22795,#22796,#22797,#22798,#22799,#22800,#22801,#22802,#22803));
#24996=AXIS2_PLACEMENT_3D('',#52482,#30411,#30412);
#24997=AXIS2_PLACEMENT_3D('',#52483,#30413,#30414);
#24998=AXIS2_PLACEMENT_3D('',#52500,#30416,#30417);
#24999=AXIS2_PLACEMENT_3D('',#52511,#30418,#30419);
#25000=AXIS2_PLACEMENT_3D('',#52549,#30421,#30422);
#25001=AXIS2_PLACEMENT_3D('',#52587,#30424,#30425);
#25002=AXIS2_PLACEMENT_3D('',#52624,#30427,#30428);
#25003=AXIS2_PLACEMENT_3D('',#52661,#30430,#30431);
#25004=AXIS2_PLACEMENT_3D('',#52699,#30433,#30434);
#25005=AXIS2_PLACEMENT_3D('',#52737,#30436,#30437);
#25006=AXIS2_PLACEMENT_3D('',#52742,#30439,#30440);
#25007=AXIS2_PLACEMENT_3D('',#52776,#30441,#30442);
#25008=AXIS2_PLACEMENT_3D('',#52798,#30444,#30445);
#25009=AXIS2_PLACEMENT_3D('',#52809,#30446,#30447);
#25010=AXIS2_PLACEMENT_3D('',#52893,#30449,#30450);
#25011=AXIS2_PLACEMENT_3D('',#52983,#30452,#30453);
#25012=AXIS2_PLACEMENT_3D('',#53073,#30455,#30456);
#25013=AXIS2_PLACEMENT_3D('',#53157,#30458,#30459);
#25014=AXIS2_PLACEMENT_3D('',#53247,#30461,#30462);
#25015=AXIS2_PLACEMENT_3D('',#53337,#30464,#30465);
#25016=AXIS2_PLACEMENT_3D('',#53421,#30467,#30468);
#25017=AXIS2_PLACEMENT_3D('',#53511,#30470,#30471);
#25018=AXIS2_PLACEMENT_3D('',#53525,#30473,#30474);
#25019=AXIS2_PLACEMENT_3D('',#53531,#30475,#30476);
#25020=AXIS2_PLACEMENT_3D('',#53569,#30478,#30479);
#25021=AXIS2_PLACEMENT_3D('',#53606,#30481,#30482);
#25022=AXIS2_PLACEMENT_3D('',#53643,#30484,#30485);
#25023=AXIS2_PLACEMENT_3D('',#53681,#30487,#30488);
#25024=AXIS2_PLACEMENT_3D('',#53718,#30490,#30491);
#25025=AXIS2_PLACEMENT_3D('',#53755,#30493,#30494);
#25026=AXIS2_PLACEMENT_3D('',#53793,#30496,#30497);
#25027=AXIS2_PLACEMENT_3D('',#53830,#30499,#30500);
#25028=AXIS2_PLACEMENT_3D('',#53909,#30501,#30502);
#25029=AXIS2_PLACEMENT_3D('',#53911,#30503,#30504);
#25030=AXIS2_PLACEMENT_3D('',#54597,#30505,#30506);
#25031=AXIS2_PLACEMENT_3D('',#54599,#30507,#30508);
#25032=AXIS2_PLACEMENT_3D('',#55200,#30509,#30510);
#25033=AXIS2_PLACEMENT_3D('',#55201,#30511,#30512);
#25034=AXIS2_PLACEMENT_3D('',#57251,#30513,#30514);
#25035=AXIS2_PLACEMENT_3D('',#57253,#30515,#30516);
#25036=AXIS2_PLACEMENT_3D('',#57254,#30517,#30518);
#25037=AXIS2_PLACEMENT_3D('',#57320,#30519,#30520);
#25038=AXIS2_PLACEMENT_3D('',#57321,#30521,#30522);
#25039=AXIS2_PLACEMENT_3D('',#59003,#30523,#30524);
#25040=AXIS2_PLACEMENT_3D('',#59005,#30525,#30526);
#25041=AXIS2_PLACEMENT_3D('',#59035,#30528,#30529);
#25042=AXIS2_PLACEMENT_3D('',#59043,#30532,#30533);
#25043=AXIS2_PLACEMENT_3D('',#59049,#30535,#30536);
#25044=AXIS2_PLACEMENT_3D('',#59055,#30538,#30539);
#25045=AXIS2_PLACEMENT_3D('',#59066,#30541,#30542);
#25046=AXIS2_PLACEMENT_3D('',#59074,#30543,#30544);
#25047=AXIS2_PLACEMENT_3D('',#59076,#30546,#30547);
#25048=AXIS2_PLACEMENT_3D('',#59077,#30548,#30549);
#25049=AXIS2_PLACEMENT_3D('',#59079,#30550,#30551);
#25050=AXIS2_PLACEMENT_3D('',#59080,#30552,#30553);
#25051=AXIS2_PLACEMENT_3D('',#59082,#30554,#30555);
#25052=AXIS2_PLACEMENT_3D('',#59083,#30556,#30557);
#25053=AXIS2_PLACEMENT_3D('',#59085,#30558,#30559);
#25054=AXIS2_PLACEMENT_3D('',#59086,#30560,#30561);
#25055=AXIS2_PLACEMENT_3D('',#59088,#30563,#30564);
#25056=AXIS2_PLACEMENT_3D('',#59089,#30565,#30566);
#25057=AXIS2_PLACEMENT_3D('',#59092,#30568,#30569);
#25058=AXIS2_PLACEMENT_3D('',#59093,#30570,#30571);
#25059=AXIS2_PLACEMENT_3D('',#59095,#30572,#30573);
#25060=AXIS2_PLACEMENT_3D('',#59097,#30575,#30576);
#25061=AXIS2_PLACEMENT_3D('',#59099,#30577,#30578);
#25062=AXIS2_PLACEMENT_3D('',#59100,#30579,#30580);
#25063=AXIS2_PLACEMENT_3D('',#59102,#30582,#30583);
#25064=AXIS2_PLACEMENT_3D('',#59104,#30584,#30585);
#25065=AXIS2_PLACEMENT_3D('',#59105,#30586,#30587);
#25066=AXIS2_PLACEMENT_3D('',#59107,#30589,#30590);
#25067=AXIS2_PLACEMENT_3D('',#59109,#30591,#30592);
#25068=AXIS2_PLACEMENT_3D('',#59111,#30594,#30595);
#25069=AXIS2_PLACEMENT_3D('',#59113,#30596,#30597);
#25070=AXIS2_PLACEMENT_3D('',#59114,#30598,#30599);
#30411=DIRECTION('axis',(0.,0.,1.));
#30412=DIRECTION('refdir',(1.,0.,0.));
#30413=DIRECTION('center_axis',(0.,0.,1.));
#30414=DIRECTION('ref_axis',(0.16099551660105,-0.986955137599659,0.));
#30415=DIRECTION('',(0.,0.,1.));
#30416=DIRECTION('center_axis',(0.,0.,1.));
#30417=DIRECTION('ref_axis',(1.,2.60858704573983E-14,0.));
#30418=DIRECTION('center_axis',(0.,0.,1.));
#30419=DIRECTION('ref_axis',(1.,2.60858704573983E-14,0.));
#30420=DIRECTION('',(0.,0.,1.));
#30421=DIRECTION('center_axis',(0.,0.,1.));
#30422=DIRECTION('ref_axis',(1.,2.60858704573983E-14,0.));
#30423=DIRECTION('',(0.,0.,1.));
#30424=DIRECTION('center_axis',(0.,0.,1.));
#30425=DIRECTION('ref_axis',(1.,2.60858704573983E-14,0.));
#30426=DIRECTION('',(0.,0.,1.));
#30427=DIRECTION('center_axis',(0.,0.,1.));
#30428=DIRECTION('ref_axis',(1.,2.60858704573983E-14,0.));
#30429=DIRECTION('',(0.,0.,1.));
#30430=DIRECTION('center_axis',(0.,0.,1.));
#30431=DIRECTION('ref_axis',(1.,2.60858704573983E-14,0.));
#30432=DIRECTION('',(0.,0.,1.));
#30433=DIRECTION('center_axis',(0.,0.,1.));
#30434=DIRECTION('ref_axis',(1.,2.60858704573983E-14,0.));
#30435=DIRECTION('',(0.,0.,1.));
#30436=DIRECTION('center_axis',(0.,0.,1.));
#30437=DIRECTION('ref_axis',(1.,2.60858704573983E-14,0.));
#30438=DIRECTION('',(0.,0.,1.));
#30439=DIRECTION('center_axis',(0.,0.,-1.));
#30440=DIRECTION('ref_axis',(1.,2.60858704573983E-14,0.));
#30441=DIRECTION('center_axis',(0.,0.,1.));
#30442=DIRECTION('ref_axis',(1.,0.,0.));
#30443=DIRECTION('',(0.,0.,-1.));
#30444=DIRECTION('center_axis',(0.,0.,-1.));
#30445=DIRECTION('ref_axis',(1.,0.,0.));
#30446=DIRECTION('center_axis',(0.,0.,1.));
#30447=DIRECTION('ref_axis',(1.,0.,0.));
#30448=DIRECTION('',(0.,0.,-1.));
#30449=DIRECTION('center_axis',(0.,0.,1.));
#30450=DIRECTION('ref_axis',(1.,0.,0.));
#30451=DIRECTION('',(0.,0.,-1.));
#30452=DIRECTION('center_axis',(0.,0.,1.));
#30453=DIRECTION('ref_axis',(1.,0.,0.));
#30454=DIRECTION('',(0.,0.,-1.));
#30455=DIRECTION('center_axis',(0.,0.,1.));
#30456=DIRECTION('ref_axis',(1.,0.,0.));
#30457=DIRECTION('',(0.,0.,-1.));
#30458=DIRECTION('center_axis',(0.,0.,1.));
#30459=DIRECTION('ref_axis',(1.,0.,0.));
#30460=DIRECTION('',(0.,0.,-1.));
#30461=DIRECTION('center_axis',(0.,0.,1.));
#30462=DIRECTION('ref_axis',(1.,0.,0.));
#30463=DIRECTION('',(0.,0.,-1.));
#30464=DIRECTION('center_axis',(0.,0.,1.));
#30465=DIRECTION('ref_axis',(1.,0.,0.));
#30466=DIRECTION('',(0.,0.,-1.));
#30467=DIRECTION('center_axis',(0.,0.,1.));
#30468=DIRECTION('ref_axis',(1.,0.,0.));
#30469=DIRECTION('',(0.,0.,-1.));
#30470=DIRECTION('center_axis',(0.,0.,1.));
#30471=DIRECTION('ref_axis',(-0.503961258530209,-0.863726258661069,0.));
#30472=DIRECTION('',(0.,0.,1.));
#30473=DIRECTION('center_axis',(0.,0.,1.));
#30474=DIRECTION('ref_axis',(1.,3.61234163283715E-14,0.));
#30475=DIRECTION('center_axis',(0.,0.,1.));
#30476=DIRECTION('ref_axis',(1.,3.61234163283715E-14,0.));
#30477=DIRECTION('',(0.,0.,1.));
#30478=DIRECTION('center_axis',(0.,0.,1.));
#30479=DIRECTION('ref_axis',(1.,3.61234163283715E-14,0.));
#30480=DIRECTION('',(0.,0.,1.));
#30481=DIRECTION('center_axis',(0.,0.,1.));
#30482=DIRECTION('ref_axis',(1.,3.61234163283715E-14,0.));
#30483=DIRECTION('',(0.,0.,1.));
#30484=DIRECTION('center_axis',(0.,0.,1.));
#30485=DIRECTION('ref_axis',(1.,3.61234163283715E-14,0.));
#30486=DIRECTION('',(0.,0.,1.));
#30487=DIRECTION('center_axis',(0.,0.,1.));
#30488=DIRECTION('ref_axis',(1.,3.61234163283715E-14,0.));
#30489=DIRECTION('',(0.,0.,1.));
#30490=DIRECTION('center_axis',(0.,0.,1.));
#30491=DIRECTION('ref_axis',(1.,3.61234163283715E-14,0.));
#30492=DIRECTION('',(0.,0.,1.));
#30493=DIRECTION('center_axis',(0.,0.,1.));
#30494=DIRECTION('ref_axis',(1.,3.61234163283715E-14,0.));
#30495=DIRECTION('',(0.,0.,1.));
#30496=DIRECTION('center_axis',(0.,0.,1.));
#30497=DIRECTION('ref_axis',(1.,3.61234163283715E-14,0.));
#30498=DIRECTION('',(0.,0.,1.));
#30499=DIRECTION('center_axis',(0.,0.,1.));
#30500=DIRECTION('ref_axis',(1.,0.,0.));
#30501=DIRECTION('center_axis',(0.,0.,-1.));
#30502=DIRECTION('ref_axis',(1.,0.,0.));
#30503=DIRECTION('center_axis',(0.,0.,-1.));
#30504=DIRECTION('ref_axis',(1.,0.,0.));
#30505=DIRECTION('center_axis',(0.,0.,1.));
#30506=DIRECTION('ref_axis',(0.888919796417206,0.458062872908941,0.));
#30507=DIRECTION('center_axis',(0.,0.,-1.));
#30508=DIRECTION('ref_axis',(1.,3.61234163283715E-14,0.));
#30509=DIRECTION('center_axis',(0.,0.,1.));
#30510=DIRECTION('ref_axis',(1.,0.,0.));
#30511=DIRECTION('center_axis',(0.,0.,-1.));
#30512=DIRECTION('ref_axis',(1.,0.,0.));
#30513=DIRECTION('center_axis',(0.,0.,1.));
#30514=DIRECTION('ref_axis',(1.,0.,0.));
#30515=DIRECTION('center_axis',(0.,0.,1.));
#30516=DIRECTION('ref_axis',(1.,0.,0.));
#30517=DIRECTION('center_axis',(0.,0.,1.));
#30518=DIRECTION('ref_axis',(1.,0.,0.));
#30519=DIRECTION('center_axis',(0.,0.,-1.));
#30520=DIRECTION('ref_axis',(1.,2.60858704573983E-14,0.));
#30521=DIRECTION('center_axis',(0.,0.,1.));
#30522=DIRECTION('ref_axis',(-0.997062769070685,0.0765887363330772,0.));
#30523=DIRECTION('center_axis',(0.,0.,1.));
#30524=DIRECTION('ref_axis',(1.,0.,0.));
#30525=DIRECTION('center_axis',(0.,0.,-1.));
#30526=DIRECTION('ref_axis',(1.,0.,0.));
#30527=DIRECTION('',(-0.866025403784439,-1.06057523872491E-16,0.5));
#30528=DIRECTION('center_axis',(0.5,-0.866025403784439,0.));
#30529=DIRECTION('ref_axis',(0.866025403784439,0.5,0.));
#30530=DIRECTION('',(0.,0.,1.));
#30531=DIRECTION('',(0.,0.,1.));
#30532=DIRECTION('center_axis',(1.,-3.49629579342466E-16,0.));
#30533=DIRECTION('ref_axis',(3.49629579342466E-16,1.,0.));
#30534=DIRECTION('',(0.,0.,1.));
#30535=DIRECTION('center_axis',(0.5,0.866025403784439,0.));
#30536=DIRECTION('ref_axis',(-0.866025403784439,0.5,0.));
#30537=DIRECTION('',(0.,0.,1.));
#30538=DIRECTION('center_axis',(0.,0.,-1.));
#30539=DIRECTION('ref_axis',(1.,0.,0.));
#30540=DIRECTION('',(0.866025403784439,1.06057523872491E-16,0.5));
#30541=DIRECTION('center_axis',(0.,0.,1.));
#30542=DIRECTION('ref_axis',(1.,0.,0.));
#30543=DIRECTION('center_axis',(-0.5,0.866025403784439,0.));
#30544=DIRECTION('ref_axis',(-0.866025403784439,-0.5,0.));
#30545=DIRECTION('',(0.,0.,1.));
#30546=DIRECTION('center_axis',(0.,0.,1.));
#30547=DIRECTION('ref_axis',(1.,0.,0.));
#30548=DIRECTION('center_axis',(0.,0.,1.));
#30549=DIRECTION('ref_axis',(1.,0.,0.));
#30550=DIRECTION('center_axis',(0.,0.,-1.));
#30551=DIRECTION('ref_axis',(1.,0.,0.));
#30552=DIRECTION('center_axis',(0.,0.,1.));
#30553=DIRECTION('ref_axis',(1.,0.,0.));
#30554=DIRECTION('center_axis',(0.,0.,-1.));
#30555=DIRECTION('ref_axis',(1.,0.,0.));
#30556=DIRECTION('center_axis',(0.,0.,1.));
#30557=DIRECTION('ref_axis',(1.,0.,0.));
#30558=DIRECTION('center_axis',(0.,0.,1.));
#30559=DIRECTION('ref_axis',(1.,0.,0.));
#30560=DIRECTION('center_axis',(-0.5,-0.866025403784439,0.));
#30561=DIRECTION('ref_axis',(0.866025403784439,-0.5,0.));
#30562=DIRECTION('',(0.,0.,1.));
#30563=DIRECTION('center_axis',(-1.,0.,0.));
#30564=DIRECTION('ref_axis',(0.,-1.,0.));
#30565=DIRECTION('center_axis',(0.,0.,1.));
#30566=DIRECTION('ref_axis',(1.,0.,0.));
#30567=DIRECTION('',(0.,0.,-1.));
#30568=DIRECTION('center_axis',(0.,0.,1.));
#30569=DIRECTION('ref_axis',(1.,0.,0.));
#30570=DIRECTION('center_axis',(0.,0.,1.));
#30571=DIRECTION('ref_axis',(1.,0.,0.));
#30572=DIRECTION('center_axis',(0.,0.,1.));
#30573=DIRECTION('ref_axis',(1.,0.,0.));
#30574=DIRECTION('',(0.,0.,-1.));
#30575=DIRECTION('center_axis',(0.,0.,-1.));
#30576=DIRECTION('ref_axis',(-1.,0.,0.));
#30577=DIRECTION('center_axis',(0.,0.,1.));
#30578=DIRECTION('ref_axis',(1.,0.,0.));
#30579=DIRECTION('center_axis',(0.,0.,1.));
#30580=DIRECTION('ref_axis',(1.,0.,0.));
#30581=DIRECTION('',(0.707106781186547,8.65956056235493E-17,-0.707106781186548));
#30582=DIRECTION('center_axis',(0.,0.,1.));
#30583=DIRECTION('ref_axis',(1.,0.,0.));
#30584=DIRECTION('center_axis',(0.,0.,1.));
#30585=DIRECTION('ref_axis',(1.,0.,0.));
#30586=DIRECTION('center_axis',(0.,0.,1.));
#30587=DIRECTION('ref_axis',(1.,0.,0.));
#30588=DIRECTION('',(0.,0.,-1.));
#30589=DIRECTION('center_axis',(0.,0.,-1.));
#30590=DIRECTION('ref_axis',(1.,0.,0.));
#30591=DIRECTION('center_axis',(0.,0.,1.));
#30592=DIRECTION('ref_axis',(1.,0.,0.));
#30593=DIRECTION('',(-0.707106781186545,-8.6595605623549E-17,-0.70710678118655));
#30594=DIRECTION('center_axis',(0.,0.,1.));
#30595=DIRECTION('ref_axis',(1.,0.,0.));
#30596=DIRECTION('center_axis',(0.,0.,1.));
#30597=DIRECTION('ref_axis',(1.,0.,0.));
#30598=DIRECTION('center_axis',(0.,0.,1.));
#30599=DIRECTION('ref_axis',(1.,0.,0.));
#30600=DIRECTION('',(0.207911690817759,2.54618386665283E-17,-0.978147600733806));
#52482=CARTESIAN_POINT('',(0.,0.,0.));
#52483=CARTESIAN_POINT('Origin',(0.,0.,-1.33003901172249));
#52484=CARTESIAN_POINT('',(-0.747455179358203,1.21560254385408E-5,-0.193723222248809));
#52485=CARTESIAN_POINT('',(-0.747444078220075,-6.40459137768446E-6,-0.187197830382769));
#52486=CARTESIAN_POINT('',(-0.7475,-1.95907305151415E-14,-1.33003901172249));
#52487=CARTESIAN_POINT('',(0.708694801171171,0.237542783106672,-0.12));
#52488=CARTESIAN_POINT('Ctrl Pts',(-0.747455179358203,1.21560254385013E-5,
-0.193723222248809));
#52489=CARTESIAN_POINT('Ctrl Pts',(-0.747409043365026,-0.0764700511820665,
-0.191546603424788));
#52490=CARTESIAN_POINT('Ctrl Pts',(-0.717056524628226,-0.275197846725086,
-0.185891997066607));
#52491=CARTESIAN_POINT('Ctrl Pts',(-0.543630981761295,-0.556730447339991,
-0.176759403174265));
#52492=CARTESIAN_POINT('Ctrl Pts',(-0.217353554555276,-0.747156946739449,
-0.166325440571785));
#52493=CARTESIAN_POINT('Ctrl Pts',(0.160155550638935,-0.76146581913925,
-0.155891477969304));
#52494=CARTESIAN_POINT('Ctrl Pts',(0.499915663487163,-0.596301280456369,
-0.145457515366823));
#52495=CARTESIAN_POINT('Ctrl Pts',(0.721838643854927,-0.290560778341026,
-0.135023552764342));
#52496=CARTESIAN_POINT('Ctrl Pts',(0.763953513632067,0.0137597889773751,
-0.126537714308735));
#52497=CARTESIAN_POINT('Ctrl Pts',(0.725795582116321,0.186572354342488,
-0.121529863387288));
#52498=CARTESIAN_POINT('Ctrl Pts',(0.708694801171171,0.237542783106672,
-0.12));
#52499=CARTESIAN_POINT('',(0.747395528060274,0.0124969850565577,-0.12));
#52500=CARTESIAN_POINT('Origin',(0.,0.,-0.12));
#52501=CARTESIAN_POINT('Ctrl Pts',(-0.747444078220075,-6.40459137771915E-6,
-0.187197830382769));
#52502=CARTESIAN_POINT('Ctrl Pts',(-0.747460394071194,-0.0538175344429418,
-0.185666478793474));
#52503=CARTESIAN_POINT('Ctrl Pts',(-0.728699568742348,-0.229832596850165,
-0.180657139670018));
#52504=CARTESIAN_POINT('Ctrl Pts',(-0.591963456523637,-0.50503391867701,
-0.172169813012403));
#52505=CARTESIAN_POINT('Ctrl Pts',(-0.284343786563672,-0.724320025643111,
-0.161735850409922));
#52506=CARTESIAN_POINT('Ctrl Pts',(0.0903167314019248,-0.772864465068914,
-0.151301887807442));
#52507=CARTESIAN_POINT('Ctrl Pts',(0.443652359236502,-0.639262442637615,
-0.140867925204961));
#52508=CARTESIAN_POINT('Ctrl Pts',(0.692489824641793,-0.354929918130671,
-0.130433962602481));
#52509=CARTESIAN_POINT('Ctrl Pts',(0.749438361810143,-0.109676867461668,
-0.12347798753416));
#52510=CARTESIAN_POINT('Ctrl Pts',(0.747395528060274,0.0124969850565577,
-0.12));
#52511=CARTESIAN_POINT('Origin',(0.,0.,-1.33003901172249));
#52512=CARTESIAN_POINT('',(-0.747444051384665,-6.42748184076532E-6,-0.327407432775125));
#52513=CARTESIAN_POINT('',(-0.747492032740272,-1.77696257386839E-5,-0.320882040909085));
#52514=CARTESIAN_POINT('',(-0.7475,-1.95907305151415E-14,-1.33003901172249));
#52515=CARTESIAN_POINT('Ctrl Pts',(-0.747444051384665,-6.42748184076503E-6,
-0.327407432775125));
#52516=CARTESIAN_POINT('Ctrl Pts',(-0.747460735268479,-0.0535655898421423,
-0.325883248386414));
#52517=CARTESIAN_POINT('Ctrl Pts',(-0.728815731862444,-0.229328242581179,
-0.320881076463544));
#52518=CARTESIAN_POINT('Ctrl Pts',(-0.592475727944838,-0.504436944883217,
-0.312400917006513));
#52519=CARTESIAN_POINT('Ctrl Pts',(-0.285071300054302,-0.724029331642761,
-0.301966954404033));
#52520=CARTESIAN_POINT('Ctrl Pts',(0.0895271131383138,-0.772961199617316,
-0.291532991801552));
#52521=CARTESIAN_POINT('Ctrl Pts',(0.443023143994609,-0.639698844990302,
-0.281099029199071));
#52522=CARTESIAN_POINT('Ctrl Pts',(0.692094455558162,-0.355653462496763,
-0.270665066596591));
#52523=CARTESIAN_POINT('Ctrl Pts',(0.778032597283113,0.0122227909580791,
-0.26023110399411));
#52524=CARTESIAN_POINT('Ctrl Pts',(0.68058114334938,0.377218004776167,-0.249797141391629));
#52525=CARTESIAN_POINT('Ctrl Pts',(0.42271031352139,0.65329941426342,-0.239363178789149));
#52526=CARTESIAN_POINT('Ctrl Pts',(0.0652026943778764,0.775391960536891,
-0.228929216186668));
#52527=CARTESIAN_POINT('Ctrl Pts',(-0.307673823063886,0.714717431064047,
-0.218495253584187));
#52528=CARTESIAN_POINT('Ctrl Pts',(-0.608028707877244,0.485577090895009,
-0.208061290981707));
#52529=CARTESIAN_POINT('Ctrl Pts',(-0.732306246915873,0.213659075752667,
-0.199803947203247));
#52530=CARTESIAN_POINT('Ctrl Pts',(-0.747482763396928,0.045739754373763,
-0.195024590958948));
#52531=CARTESIAN_POINT('Ctrl Pts',(-0.747455179358203,1.21560254385013E-5,
-0.193723222248809));
#52532=CARTESIAN_POINT('Ctrl Pts',(-0.747492032740272,-1.77696257387602E-5,
-0.320882040909085));
#52533=CARTESIAN_POINT('Ctrl Pts',(-0.747521461794713,-0.0308968347335454,
-0.3200031237551));
#52534=CARTESIAN_POINT('Ctrl Pts',(-0.738208053524619,-0.183950674319056,
-0.315646219066955));
#52535=CARTESIAN_POINT('Ctrl Pts',(-0.635857117988054,-0.448519615362855,
-0.307811326844651));
#52536=CARTESIAN_POINT('Ctrl Pts',(-0.349675784487414,-0.695133774103566,
-0.29737736424217));
#52537=CARTESIAN_POINT('Ctrl Pts',(0.0189274157531999,-0.777898369643473,
-0.28694340163969));
#52538=CARTESIAN_POINT('Ctrl Pts',(0.383069251609923,-0.677305003145055,
-0.276509439037209));
#52539=CARTESIAN_POINT('Ctrl Pts',(0.656918053157327,-0.417064487823471,
-0.266075476434728));
#52540=CARTESIAN_POINT('Ctrl Pts',(0.775925115315039,-0.0585179376441868,
-0.255641513832248));
#52541=CARTESIAN_POINT('Ctrl Pts',(0.712039292365906,0.313821812003498,
-0.245207551229767));
#52542=CARTESIAN_POINT('Ctrl Pts',(0.480319196218488,0.612190866640268,
-0.234773588627287));
#52543=CARTESIAN_POINT('Ctrl Pts',(0.135383189993233,0.766260668703223,
-0.224339626024806));
#52544=CARTESIAN_POINT('Ctrl Pts',(-0.24146359128836,0.739715845333337,
-0.213905663422326));
#52545=CARTESIAN_POINT('Ctrl Pts',(-0.561395755032477,0.538812615893194,
-0.203471700819845));
#52546=CARTESIAN_POINT('Ctrl Pts',(-0.721466439761006,0.259032440630972,
-0.194569089806659));
#52547=CARTESIAN_POINT('Ctrl Pts',(-0.747423337703997,0.0683976642946505,
-0.189144466327634));
#52548=CARTESIAN_POINT('Ctrl Pts',(-0.747444078220075,-6.40459137771915E-6,
-0.187197830382769));
#52549=CARTESIAN_POINT('Origin',(0.,0.,-1.33003901172249));
#52550=CARTESIAN_POINT('',(-0.747492771866375,-1.77854026473198E-5,-0.461091643301441));
#52551=CARTESIAN_POINT('',(-0.747552914013562,-7.59237280051339E-6,-0.4545662514354));
#52552=CARTESIAN_POINT('',(-0.7475,-1.95907305151415E-14,-1.33003901172249));
#52553=CARTESIAN_POINT('Ctrl Pts',(-0.747492771866375,-1.7785402647276E-5,
-0.461091643301441));
#52554=CARTESIAN_POINT('Ctrl Pts',(-0.747522042549812,-0.030644957535598,
-0.460219893348041));
#52555=CARTESIAN_POINT('Ctrl Pts',(-0.738300189612616,-0.183446679313347,
-0.455870155860481));
#52556=CARTESIAN_POINT('Ctrl Pts',(-0.636310057828864,-0.447876802013019,
-0.448042430838761));
#52557=CARTESIAN_POINT('Ctrl Pts',(-0.350378094607062,-0.694780044542988,
-0.43760846823628));
#52558=CARTESIAN_POINT('Ctrl Pts',(0.018141279213836,-0.777917099351843,
-0.4271745056338));
#52559=CARTESIAN_POINT('Ctrl Pts',(0.382384582988471,-0.677691781098527,
-0.416740543031318));
#52560=CARTESIAN_POINT('Ctrl Pts',(0.656496245978099,-0.417728139454391,
-0.406306580428839));
#52561=CARTESIAN_POINT('Ctrl Pts',(0.775865572452268,-0.0593020485231031,
-0.395872617826358));
#52562=CARTESIAN_POINT('Ctrl Pts',(0.712356090039248,0.313102092711016,
-0.385438655223878));
#52563=CARTESIAN_POINT('Ctrl Pts',(0.480937580760017,0.611705127399059,
-0.375004692621396));
#52564=CARTESIAN_POINT('Ctrl Pts',(0.136157562681009,0.766123513283346,
-0.364570730018916));
#52565=CARTESIAN_POINT('Ctrl Pts',(-0.240716072858239,0.739959385191355,
-0.354136767416435));
#52566=CARTESIAN_POINT('Ctrl Pts',(-0.560850667196372,0.539379874112091,
-0.343702804813955));
#52567=CARTESIAN_POINT('Ctrl Pts',(-0.721333836132676,0.259535992032645,
-0.334793026600185));
#52568=CARTESIAN_POINT('Ctrl Pts',(-0.747422664848419,0.0686493471490352,
-0.329361235920575));
#52569=CARTESIAN_POINT('Ctrl Pts',(-0.747444051384665,-6.42748184076503E-6,
-0.327407432775125));
#52570=CARTESIAN_POINT('Ctrl Pts',(-0.747552914013563,-7.59237280050992E-6,
-0.4545662514354));
#52571=CARTESIAN_POINT('Ctrl Pts',(-0.747557174200554,-0.0079627541396081,
-0.454339768716727));
#52572=CARTESIAN_POINT('Ctrl Pts',(-0.745521898301695,-0.13807937304922,
-0.450635298463893));
#52573=CARTESIAN_POINT('Ctrl Pts',(-0.674371225051021,-0.388210728933227,
-0.443452840676899));
#52574=CARTESIAN_POINT('Ctrl Pts',(-0.412054943730932,-0.660071846531001,
-0.433018878074418));
#52575=CARTESIAN_POINT('Ctrl Pts',(-0.052613438684712,-0.776347824950466,
-0.422584915471938));
#52576=CARTESIAN_POINT('Ctrl Pts',(0.319229548446942,-0.709631323036312,
-0.412150952869457));
#52577=CARTESIAN_POINT('Ctrl Pts',(0.615827130120364,-0.475648047450975,
-0.401716990266977));
#52578=CARTESIAN_POINT('Ctrl Pts',(0.767268468189366,-0.129550055793595,
-0.391283027664495));
#52579=CARTESIAN_POINT('Ctrl Pts',(0.73785741566876,0.247084101843196,-0.380849065062015));
#52580=CARTESIAN_POINT('Ctrl Pts',(0.53452643409528,0.565478213973466,-0.370415102459534));
#52581=CARTESIAN_POINT('Ctrl Pts',(0.205202547258297,0.750583795355784,
-0.359981139857054));
#52582=CARTESIAN_POINT('Ctrl Pts',(-0.172489509004575,0.758769720339227,
-0.349547177254573));
#52583=CARTESIAN_POINT('Ctrl Pts',(-0.509524166428119,0.588106489551374,
-0.339113214652092));
#52584=CARTESIAN_POINT('Ctrl Pts',(-0.708185410677575,0.304874056256311,
-0.329558169203597));
#52585=CARTESIAN_POINT('Ctrl Pts',(-0.747405007264241,0.0912955733046984,
-0.323481111289261));
#52586=CARTESIAN_POINT('Ctrl Pts',(-0.747492032740272,-1.77696257387602E-5,
-0.320882040909085));
#52587=CARTESIAN_POINT('Origin',(0.,0.,-1.33003901172249));
#52588=CARTESIAN_POINT('',(-0.747553321122147,-7.36938303809654E-6,-0.594775853827757));
#52589=CARTESIAN_POINT('',(-0.747538056636855,1.30170342584265E-5,-0.588250461961717));
#52590=CARTESIAN_POINT('',(-0.7475,-1.95907305151415E-14,-1.33003901172249));
#52591=CARTESIAN_POINT('Ctrl Pts',(-0.747553321122147,-7.36938303808141E-6,
-0.594775853827757));
#52592=CARTESIAN_POINT('Ctrl Pts',(-0.74755734320473,-0.0077107724177583,
-0.594556538309668));
#52593=CARTESIAN_POINT('Ctrl Pts',(-0.745590310689939,-0.137575565048743,
-0.590859235257418));
#52594=CARTESIAN_POINT('Ctrl Pts',(-0.674763198638609,-0.387529025027267,
-0.583683944671009));
#52595=CARTESIAN_POINT('Ctrl Pts',(-0.412721788492083,-0.659655095318369,
-0.573249982068528));
#52596=CARTESIAN_POINT('Ctrl Pts',(-0.0533979730410179,-0.776294258609907,
-0.562816019466048));
#52597=CARTESIAN_POINT('Ctrl Pts',(0.318512246619034,-0.709953567657271,
-0.552382056863567));
#52598=CARTESIAN_POINT('Ctrl Pts',(0.615346135603011,-0.476270146948171,
-0.541948094261087));
#52599=CARTESIAN_POINT('Ctrl Pts',(0.767137155915032,-0.130325375465359,
-0.531514131658606));
#52600=CARTESIAN_POINT('Ctrl Pts',(0.738106737168653,0.246338312127523,
-0.521080169056125));
#52601=CARTESIAN_POINT('Ctrl Pts',(0.535097621960437,0.564937743869073,
-0.510646206453644));
#52602=CARTESIAN_POINT('Ctrl Pts',(0.205960967115317,0.750376038730258,
-0.500212243851164));
#52603=CARTESIAN_POINT('Ctrl Pts',(-0.171722623797879,0.758943647414989,
-0.489778281248683));
#52604=CARTESIAN_POINT('Ctrl Pts',(-0.508929578017626,0.588621104017168,
-0.479344318646203));
#52605=CARTESIAN_POINT('Ctrl Pts',(-0.708026179252435,0.305377277568611,
-0.469782105997121));
#52606=CARTESIAN_POINT('Ctrl Pts',(-0.747405262420699,0.0915471027788979,
-0.463697880882201));
#52607=CARTESIAN_POINT('Ctrl Pts',(-0.747492771866375,-1.7785402647276E-5,
-0.461091643301441));
#52608=CARTESIAN_POINT('Ctrl Pts',(-0.747538056636855,1.30170342584213E-5,
-0.588250461961717));
#52609=CARTESIAN_POINT('Ctrl Pts',(-0.747449782311828,-0.107195335869156,
-0.585198426144193));
#52610=CARTESIAN_POINT('Ctrl Pts',(-0.697538394050389,-0.336653954873882,
-0.578668402792509));
#52611=CARTESIAN_POINT('Ctrl Pts',(-0.470949408769063,-0.619427779176754,
-0.568660391906666));
#52612=CARTESIAN_POINT('Ctrl Pts',(-0.123709349589915,-0.768231811408391,
-0.558226429304186));
#52613=CARTESIAN_POINT('Ctrl Pts',(0.25269016620706,-0.735956383991622,
-0.547792466701704));
#52614=CARTESIAN_POINT('Ctrl Pts',(0.569528234436074,-0.530209118571064,
-0.537358504099225));
#52615=CARTESIAN_POINT('Ctrl Pts',(0.752123144005562,-0.199486579716445,
-0.526924541496743));
#52616=CARTESIAN_POINT('Ctrl Pts',(0.757435558261681,0.178256821234392,
-0.516490578894263));
#52617=CARTESIAN_POINT('Ctrl Pts',(0.58421329122536,0.513983413731815,-0.506056616291782));
#52618=CARTESIAN_POINT('Ctrl Pts',(0.273286459598611,0.728559283954183,
-0.495622653689302));
#52619=CARTESIAN_POINT('Ctrl Pts',(-0.102056559562228,0.771406882187409,
-0.485188691086821));
#52620=CARTESIAN_POINT('Ctrl Pts',(-0.453343888260037,0.632426626742619,
-0.47475472848434));
#52621=CARTESIAN_POINT('Ctrl Pts',(-0.692468131949326,0.350629951601094,
-0.464547248600534));
#52622=CARTESIAN_POINT('Ctrl Pts',(-0.74749175253247,0.114200886509029,
-0.457817756250887));
#52623=CARTESIAN_POINT('Ctrl Pts',(-0.747552914013563,-7.59237280050992E-6,
-0.4545662514354));
#52624=CARTESIAN_POINT('Origin',(0.,0.,-1.33003901172249));
#52625=CARTESIAN_POINT('',(-0.747537418840408,1.3179381549518E-5,-0.728460064354072));
#52626=CARTESIAN_POINT('',(-0.747472643624562,1.62103417219173E-5,-0.721934672488032));
#52627=CARTESIAN_POINT('',(-0.7475,-1.95907305151415E-14,-1.33003901172249));
#52628=CARTESIAN_POINT('Ctrl Pts',(-0.747537418840409,1.31793815494937E-5,
-0.728460064354072));
#52629=CARTESIAN_POINT('Ctrl Pts',(-0.747448558105652,-0.106943676944281,
-0.725415195737134));
#52630=CARTESIAN_POINT('Ctrl Pts',(-0.697716187447847,-0.336151536347626,
-0.718892339586036));
#52631=CARTESIAN_POINT('Ctrl Pts',(-0.471575149406303,-0.618951531170264,
-0.708891495900775));
#52632=CARTESIAN_POINT('Ctrl Pts',(-0.124485645778937,-0.768106401138926,
-0.698457533298296));
#52633=CARTESIAN_POINT('Ctrl Pts',(0.251946294775518,-0.736211371838604,
-0.688023570695814));
#52634=CARTESIAN_POINT('Ctrl Pts',(0.568992125251127,-0.530784401501963,
-0.677589608093334));
#52635=CARTESIAN_POINT('Ctrl Pts',(0.751921163041749,-0.200246558136551,
-0.667155645490854));
#52636=CARTESIAN_POINT('Ctrl Pts',(0.757615314330881,0.177491281382813,
-0.656721682888373));
#52637=CARTESIAN_POINT('Ctrl Pts',(0.584732414132277,0.513392757388173,
-0.646287720285892));
#52638=CARTESIAN_POINT('Ctrl Pts',(0.274022587194117,0.728282734371093,
-0.635853757683412));
#52639=CARTESIAN_POINT('Ctrl Pts',(-0.101276939472307,0.771509624701283,
-0.625419795080931));
#52640=CARTESIAN_POINT('Ctrl Pts',(-0.452704539459636,0.632884443977122,
-0.61498583247845));
#52641=CARTESIAN_POINT('Ctrl Pts',(-0.69228154043425,0.351131872468849,
-0.604771185394059));
#52642=CARTESIAN_POINT('Ctrl Pts',(-0.747493559514422,0.114452674833002,
-0.598034525843828));
#52643=CARTESIAN_POINT('Ctrl Pts',(-0.747553321122147,-7.36938303808141E-6,
-0.594775853827757));
#52644=CARTESIAN_POINT('Ctrl Pts',(-0.747472643624562,1.62103417219207E-5,
-0.721934672488032));
#52645=CARTESIAN_POINT('Ctrl Pts',(-0.747402612221546,-0.0842954619945286,
-0.71953507110582));
#52646=CARTESIAN_POINT('Ctrl Pts',(-0.712499566770546,-0.290865199736192,
-0.713657482189446));
#52647=CARTESIAN_POINT('Ctrl Pts',(-0.525861117638762,-0.573545293931952,
-0.704301905738914));
#52648=CARTESIAN_POINT('Ctrl Pts',(-0.19375906706945,-0.753618964174968,
-0.693867943136433));
#52649=CARTESIAN_POINT('Ctrl Pts',(0.184013817024176,-0.756057560229359,
-0.683433980533953));
#52650=CARTESIAN_POINT('Ctrl Pts',(0.518412914638575,-0.580286282081279,
-0.673000017931471));
#52651=CARTESIAN_POINT('Ctrl Pts',(0.73061721497504,-0.267736072313561,
-0.662566055328992));
#52652=CARTESIAN_POINT('Ctrl Pts',(0.770608169635336,0.107922046529214,
-0.65213209272651));
#52653=CARTESIAN_POINT('Ctrl Pts',(0.628959534674377,0.458141924492801,
-0.641698130124031));
#52654=CARTESIAN_POINT('Ctrl Pts',(0.339059224908709,0.700373444128261,
-0.631264167521549));
#52655=CARTESIAN_POINT('Ctrl Pts',(-0.0307605314660725,0.777520359180196,
-0.620830204919069));
#52656=CARTESIAN_POINT('Ctrl Pts',(-0.393329741412475,0.671398416557689,
-0.610396242316588));
#52657=CARTESIAN_POINT('Ctrl Pts',(-0.663187433844336,0.407021555727386,
-0.599962279714107));
#52658=CARTESIAN_POINT('Ctrl Pts',(-0.74351458894893,0.152101734785077,
-0.592580352929151));
#52659=CARTESIAN_POINT('Ctrl Pts',(-0.747550376479258,0.0149753519108104,
-0.588676413678354));
#52660=CARTESIAN_POINT('Ctrl Pts',(-0.747538056636855,1.30170342584213E-5,
-0.588250461961717));
#52661=CARTESIAN_POINT('Origin',(0.,0.,-1.33003901172249));
#52662=CARTESIAN_POINT('',(-0.747472002174667,1.61159471936687E-5,-0.862144274880388));
#52663=CARTESIAN_POINT('',(-0.747440403350747,2.49991181755504E-7,-0.855618883014348));
#52664=CARTESIAN_POINT('',(-0.7475,-1.95907305151415E-14,-1.33003901172249));
#52665=CARTESIAN_POINT('Ctrl Pts',(-0.747472002174667,1.61159471936886E-5,
-0.862144274880388));
#52666=CARTESIAN_POINT('Ctrl Pts',(-0.747402682287736,-0.0840439390973357,
-0.85975184069876));
#52667=CARTESIAN_POINT('Ctrl Pts',(-0.712650382827926,-0.290361716183336,
-0.853881418982972));
#52668=CARTESIAN_POINT('Ctrl Pts',(-0.526440462347929,-0.573013576696856,
-0.844533009733024));
#52669=CARTESIAN_POINT('Ctrl Pts',(-0.194520560057908,-0.753422770554805,
-0.834099047130543));
#52670=CARTESIAN_POINT('Ctrl Pts',(0.183249666810382,-0.756243134903882,
-0.823665084528063));
#52671=CARTESIAN_POINT('Ctrl Pts',(0.517826224589069,-0.580809883355641,
-0.813231121925582));
#52672=CARTESIAN_POINT('Ctrl Pts',(0.730346273449163,-0.268474282445114,
-0.802797159323102));
#52673=CARTESIAN_POINT('Ctrl Pts',(0.770716840097935,0.107143230607854,
-0.79236319672062));
#52674=CARTESIAN_POINT('Ctrl Pts',(0.62942220247575,0.457506077015547,-0.781929234118141));
#52675=CARTESIAN_POINT('Ctrl Pts',(0.339766834898864,0.700030440322706,
-0.77149527151566));
#52676=CARTESIAN_POINT('Ctrl Pts',(-0.0299747696136753,0.777551048267701,
-0.761061308913179));
#52677=CARTESIAN_POINT('Ctrl Pts',(-0.392651039152919,0.671795564831833,
-0.750627346310698));
#52678=CARTESIAN_POINT('Ctrl Pts',(-0.66277576768029,0.4076915516066,-0.740193383708219));
#52679=CARTESIAN_POINT('Ctrl Pts',(-0.743438739207482,0.152605612016255,
-0.732804289722676));
#52680=CARTESIAN_POINT('Ctrl Pts',(-0.747550058881758,0.0152273129384325,
-0.728893183271294));
#52681=CARTESIAN_POINT('Ctrl Pts',(-0.747537418840409,1.31793815494937E-5,
-0.728460064354072));
#52682=CARTESIAN_POINT('Ctrl Pts',(-0.747440403350747,2.49991181772852E-7,
-0.855618883014348));
#52683=CARTESIAN_POINT('Ctrl Pts',(-0.747439664227336,-0.0613952789202318,
-0.853871716067446));
#52684=CARTESIAN_POINT('Ctrl Pts',(-0.725057127938405,-0.245007983420982,
-0.848646561586384));
#52685=CARTESIAN_POINT('Ctrl Pts',(-0.576325689361536,-0.522812412838008,
-0.839943419571161));
#52686=CARTESIAN_POINT('Ctrl Pts',(-0.262170190030731,-0.732632862145289,
-0.829509456968681));
#52687=CARTESIAN_POINT('Ctrl Pts',(0.113781287599417,-0.769764858789943,
-0.8190754943662));
#52688=CARTESIAN_POINT('Ctrl Pts',(0.462913446150841,-0.625456042107333,
-0.808641531763721));
#52689=CARTESIAN_POINT('Ctrl Pts',(0.702932553865032,-0.333721356752229,
-0.798207569161239));
#52690=CARTESIAN_POINT('Ctrl Pts',(0.77726385077405,0.036674589509254,-0.787773606558759));
#52691=CARTESIAN_POINT('Ctrl Pts',(0.668386751451238,0.398425990267,-0.777339643956278));
#52692=CARTESIAN_POINT('Ctrl Pts',(0.401964611697131,0.666264639748313,
-0.766905681353797));
#52693=CARTESIAN_POINT('Ctrl Pts',(0.0407956343310049,0.777058450475451,
-0.756471718751316));
#52694=CARTESIAN_POINT('Ctrl Pts',(-0.329989257542916,0.704692279751986,
-0.746037756148837));
#52695=CARTESIAN_POINT('Ctrl Pts',(-0.622992579377318,0.466223514289631,
-0.735603793546355));
#52696=CARTESIAN_POINT('Ctrl Pts',(-0.735537269423189,0.197977738940191,
-0.727569432326088));
#52697=CARTESIAN_POINT('Ctrl Pts',(-0.747504115891487,0.0379060617849304,
-0.72301305863998));
#52698=CARTESIAN_POINT('Ctrl Pts',(-0.747472643624562,1.62103417219207E-5,
-0.721934672488032));
#52699=CARTESIAN_POINT('Origin',(0.,0.,-1.33003901172249));
#52700=CARTESIAN_POINT('',(-0.747440394010334,2.88097105794361E-8,-0.995828485406704));
#52701=CARTESIAN_POINT('',(-0.747471187093045,-1.59917937688492E-5,-0.989303093540664));
#52702=CARTESIAN_POINT('',(-0.7475,-1.95907305151415E-14,-1.33003901172249));
#52703=CARTESIAN_POINT('Ctrl Pts',(-0.747440394010334,2.88097105755059E-8,
-0.995828485406704));
#52704=CARTESIAN_POINT('Ctrl Pts',(-0.747440305752118,-0.0611436444929975,
-0.994088485660387));
#52705=CARTESIAN_POINT('Ctrl Pts',(-0.725182114079541,-0.244504027566075,
-0.98887049837991));
#52706=CARTESIAN_POINT('Ctrl Pts',(-0.576853733233579,-0.522229725565813,
-0.980174523565272));
#52707=CARTESIAN_POINT('Ctrl Pts',(-0.262910442753169,-0.732367543071951,
-0.969740560962791));
#52708=CARTESIAN_POINT('Ctrl Pts',(0.113003322331731,-0.769879451565163,
-0.95930659836031));
#52709=CARTESIAN_POINT('Ctrl Pts',(0.462281136078411,-0.625923533367173,
-0.948872635757831));
#52710=CARTESIAN_POINT('Ctrl Pts',(0.70259494345804,-0.334431555819595,
-0.938438673155348));
#52711=CARTESIAN_POINT('Ctrl Pts',(0.777300516433144,0.0358890839459567,
-0.928004710552869));
#52712=CARTESIAN_POINT('Ctrl Pts',(0.668789051521525,0.397750328889645,
-0.917570747950388));
#52713=CARTESIAN_POINT('Ctrl Pts',(0.402637719871012,0.665858082479752,
-0.907136785347908));
#52714=CARTESIAN_POINT('Ctrl Pts',(0.0415808928872875,0.777016826591824,
-0.896702822745427));
#52715=CARTESIAN_POINT('Ctrl Pts',(-0.32927694153081,0.705025400441648,
-0.886268860142946));
#52716=CARTESIAN_POINT('Ctrl Pts',(-0.622521105437113,0.466852859850313,
-0.875834897540466));
#52717=CARTESIAN_POINT('Ctrl Pts',(-0.735437461077155,0.198481764760452,
-0.867793369119613));
#52718=CARTESIAN_POINT('Ctrl Pts',(-0.747503455677645,0.038157886060821,
-0.86322982823292));
#52719=CARTESIAN_POINT('Ctrl Pts',(-0.747472002174667,1.61159471936886E-5,
-0.862144274880388));
#52720=CARTESIAN_POINT('Ctrl Pts',(-0.747471187093045,-1.59917937688908E-5,
-0.989303093540664));
#52721=CARTESIAN_POINT('Ctrl Pts',(-0.747502606642687,-0.0384803988601513,
-0.988208361029073));
#52722=CARTESIAN_POINT('Ctrl Pts',(-0.735309243690986,-0.199127278369172,
-0.983635640983321));
#52723=CARTESIAN_POINT('Ctrl Pts',(-0.621916351700691,-0.467658178639452,
-0.97558493340341));
#52724=CARTESIAN_POINT('Ctrl Pts',(-0.328364174807744,-0.705450981188053,
-0.965150970800929));
#52725=CARTESIAN_POINT('Ctrl Pts',(0.0425865250681738,-0.776962359283856,
-0.954717008198449));
#52726=CARTESIAN_POINT('Ctrl Pts',(0.403499180542324,-0.665336403825433,
-0.944283045595967));
#52727=CARTESIAN_POINT('Ctrl Pts',(0.669303286159026,-0.396884404409992,
-0.933849082993487));
#52728=CARTESIAN_POINT('Ctrl Pts',(0.777346315469045,-0.0348830195569247,
-0.923415120391007));
#52729=CARTESIAN_POINT('Ctrl Pts',(0.702161510858138,0.335340620697414,
-0.912981157788526));
#52730=CARTESIAN_POINT('Ctrl Pts',(0.461470637519424,0.626521324425116,
-0.902547195186045));
#52731=CARTESIAN_POINT('Ctrl Pts',(0.112006796904718,0.770025062366403,
-0.892113232583565));
#52732=CARTESIAN_POINT('Ctrl Pts',(-0.26385809865297,0.732026654580473,
-0.881679269981084));
#52733=CARTESIAN_POINT('Ctrl Pts',(-0.577529159980992,0.521482682939164,
-0.871245307378604));
#52734=CARTESIAN_POINT('Ctrl Pts',(-0.72534176137517,0.243858607071591,
-0.862558511723024));
#52735=CARTESIAN_POINT('Ctrl Pts',(-0.747441135558977,0.0608213670538153,
-0.857349703601606));
#52736=CARTESIAN_POINT('Ctrl Pts',(-0.747440403350747,2.49991181772852E-7,
-0.855618883014348));
#52737=CARTESIAN_POINT('Origin',(0.,0.,-1.33003901172249));
#52738=CARTESIAN_POINT('',(-0.7475,-1.95907305151415E-14,-1.12625));
#52739=CARTESIAN_POINT('',(-0.747536615034749,-1.54000427277645E-5,-1.12298730406698));
#52740=CARTESIAN_POINT('',(-0.7475,-1.95907305151415E-14,-1.33003901172249));
#52741=CARTESIAN_POINT('',(-0.738728321778978,-0.114178441930227,-1.12625));
#52742=CARTESIAN_POINT('Origin',(0.,0.,-1.12625));
#52743=CARTESIAN_POINT('Ctrl Pts',(-0.738728321778979,-0.114178441930225,
-1.12625));
#52744=CARTESIAN_POINT('Ctrl Pts',(-0.720064014057808,-0.234935499803312,
-1.12277201246584));
#52745=CARTESIAN_POINT('Ctrl Pts',(-0.622428467720147,-0.467011987146758,
-1.11581603739752));
#52746=CARTESIAN_POINT('Ctrl Pts',(-0.329058176975973,-0.705127368582215,
-1.10538207479504));
#52747=CARTESIAN_POINT('Ctrl Pts',(0.0417919283474016,-0.77700066177415,
-1.09494811219256));
#52748=CARTESIAN_POINT('Ctrl Pts',(0.402831360764571,-0.66574603450436,
-1.08451414959008));
#52749=CARTESIAN_POINT('Ctrl Pts',(0.66889944257465,-0.397559467050142,
-1.0740801869876));
#52750=CARTESIAN_POINT('Ctrl Pts',(0.77731189566657,-0.0356691406410475,
-1.06364622438512));
#52751=CARTESIAN_POINT('Ctrl Pts',(0.70249941623784,0.334631148448006,-1.05321226178264));
#52752=CARTESIAN_POINT('Ctrl Pts',(0.462103868983754,0.626054505003761,
-1.04277829918016));
#52753=CARTESIAN_POINT('Ctrl Pts',(0.112784749994043,0.769911552166373,
-1.03234433657767));
#52754=CARTESIAN_POINT('Ctrl Pts',(-0.263118110857165,0.732292892594137,
-1.02191037397519));
#52755=CARTESIAN_POINT('Ctrl Pts',(-0.577001907123833,0.522066075167691,
-1.01147641137271));
#52756=CARTESIAN_POINT('Ctrl Pts',(-0.725217128854169,0.244362557690023,
-1.00278244851655));
#52757=CARTESIAN_POINT('Ctrl Pts',(-0.747440482166499,0.061073001796564,
-0.997566473194547));
#52758=CARTESIAN_POINT('Ctrl Pts',(-0.747440394010334,2.88097105755059E-8,
-0.995828485406704));
#52759=CARTESIAN_POINT('Ctrl Pts',(-0.747536615034749,-1.54000427278131E-5,
-1.12298730406698));
#52760=CARTESIAN_POINT('Ctrl Pts',(-0.747549574643972,-0.0155531187576153,
-1.1225450059907));
#52761=CARTESIAN_POINT('Ctrl Pts',(-0.743340401009098,-0.153262521212314,
-1.11862472038026));
#52762=CARTESIAN_POINT('Ctrl Pts',(-0.662248238305512,-0.408538693637006,
-1.11122644723566));
#52763=CARTESIAN_POINT('Ctrl Pts',(-0.391780881856498,-0.672308433025162,
-1.10079248463318));
#52764=CARTESIAN_POINT('Ctrl Pts',(-0.0289685614302447,-0.77758653236944,
-1.0903585220307));
#52765=CARTESIAN_POINT('Ctrl Pts',(0.340672665444815,-0.699591456600573,
-1.07992455942822));
#52766=CARTESIAN_POINT('Ctrl Pts',(0.630013764781798,-0.45669036663525,
-1.06949059682573));
#52767=CARTESIAN_POINT('Ctrl Pts',(0.770854889346007,-0.106145976774946,
-1.05905663422326));
#52768=CARTESIAN_POINT('Ctrl Pts',(0.72999817257357,0.269419497799126,-1.04862267162077));
#52769=CARTESIAN_POINT('Ctrl Pts',(0.517074073818034,0.581479511865617,
-1.03818870901829));
#52770=CARTESIAN_POINT('Ctrl Pts',(0.182270729955259,0.756479721113076,
-1.02775474641581));
#52771=CARTESIAN_POINT('Ctrl Pts',(-0.195495525574089,0.753170354596227,
-1.01732078381333));
#52772=CARTESIAN_POINT('Ctrl Pts',(-0.527181654493514,0.572331754114927,
-1.00688682121085));
#52773=CARTESIAN_POINT('Ctrl Pts',(-0.712843111741135,0.28971688006118,
-0.997547591119962));
#52774=CARTESIAN_POINT('Ctrl Pts',(-0.747402786092163,0.0837218074955242,
-0.991686348563233));
#52775=CARTESIAN_POINT('Ctrl Pts',(-0.747471187093045,-1.59917937688908E-5,
-0.989303093540664));
#52776=CARTESIAN_POINT('Origin',(0.,0.,1.095));
#52777=CARTESIAN_POINT('',(-0.792490573374725,2.00326525206102E-5,0.848268682536521));
#52778=CARTESIAN_POINT('',(-0.792490189019743,1.3140117316485E-5,0.826731317463479));
#52779=CARTESIAN_POINT('',(-0.7925,-9.70532588324277E-17,1.095));
#52780=CARTESIAN_POINT('',(0.345478907940192,0.713232482552815,0.8));
#52781=CARTESIAN_POINT('Ctrl Pts',(-0.792490573374725,2.00326525206102E-5,
0.848268682536521));
#52782=CARTESIAN_POINT('Ctrl Pts',(-0.792523353183581,0.0333301751535281,
0.847265264173584));
#52783=CARTESIAN_POINT('Ctrl Pts',(-0.790462051371192,0.0666362775783571,
0.846261845810648));
#52784=CARTESIAN_POINT('Ctrl Pts',(-0.786274148538905,0.0996727818564752,
0.845258427447711));
#52785=CARTESIAN_POINT('Ctrl Pts',(-0.769804202821169,0.22959686413684,
0.841312240864219));
#52786=CARTESIAN_POINT('Ctrl Pts',(-0.720443250858591,0.355351215356187,
0.837366054280727));
#52787=CARTESIAN_POINT('Ctrl Pts',(-0.644137104498692,0.461788800755913,
0.833419867697236));
#52788=CARTESIAN_POINT('Ctrl Pts',(-0.567830958138792,0.568226386155639,
0.829473681113744));
#52789=CARTESIAN_POINT('Ctrl Pts',(-0.46457961738157,0.655347205735744,
0.825527494530252));
#52790=CARTESIAN_POINT('Ctrl Pts',(-0.346820261793125,0.712655533465586,
0.821581307946761));
#52791=CARTESIAN_POINT('Ctrl Pts',(-0.229060906204681,0.769963861195427,
0.817635121363269));
#52792=CARTESIAN_POINT('Ctrl Pts',(-0.0967935357850139,0.797459697075005,
0.813688934779777));
#52793=CARTESIAN_POINT('Ctrl Pts',(0.0340494680202196,0.791834055085671,
0.809742748196285));
#52794=CARTESIAN_POINT('Ctrl Pts',(0.141728988687317,0.787204335381606,
0.80649516546419));
#52795=CARTESIAN_POINT('Ctrl Pts',(0.248443821076452,0.760142257936812,
0.803247582732095));
#52796=CARTESIAN_POINT('Ctrl Pts',(0.345504974425202,0.713245911452251,
0.8));
#52797=CARTESIAN_POINT('',(-0.345478907940189,0.713232482552817,0.8));
#52798=CARTESIAN_POINT('Origin',(0.,0.,0.8));
#52799=CARTESIAN_POINT('Ctrl Pts',(-0.345478907940187,0.713232482552818,
0.8));
#52800=CARTESIAN_POINT('Ctrl Pts',(-0.463374437871894,0.656125690688751,
0.803946186583492));
#52801=CARTESIAN_POINT('Ctrl Pts',(-0.56678182300553,0.569256548592082,
0.807892373166983));
#52802=CARTESIAN_POINT('Ctrl Pts',(-0.64328331919897,0.462978698222646,
0.811838559750475));
#52803=CARTESIAN_POINT('Ctrl Pts',(-0.719784815392412,0.356700847853208,
0.815784746333967));
#52804=CARTESIAN_POINT('Ctrl Pts',(-0.769380422645657,0.231014289211002,
0.819730932917459));
#52805=CARTESIAN_POINT('Ctrl Pts',(-0.786090265814568,0.101114707806154,
0.823677119500951));
#52806=CARTESIAN_POINT('Ctrl Pts',(-0.790401192991213,0.0676022666627898,
0.82469518548846));
#52807=CARTESIAN_POINT('Ctrl Pts',(-0.792523327817215,0.0338094174993378,
0.82571325147597));
#52808=CARTESIAN_POINT('Ctrl Pts',(-0.792490189019743,1.3140117316485E-5,
0.826731317463479));
#52809=CARTESIAN_POINT('Origin',(0.,0.,1.095));
#52810=CARTESIAN_POINT('',(-0.792556380474703,-9.7200913266593E-6,0.99826868253652));
#52811=CARTESIAN_POINT('',(-0.792557287165952,-9.28448389212729E-6,0.97673131746348));
#52812=CARTESIAN_POINT('',(-0.7925,-9.70532588324277E-17,1.095));
#52813=CARTESIAN_POINT('Ctrl Pts',(-0.792556380474703,-9.7200913266593E-6,
0.99826868253652));
#52814=CARTESIAN_POINT('Ctrl Pts',(-0.792481403648174,0.121101794392974,
0.994619503175485));
#52815=CARTESIAN_POINT('Ctrl Pts',(-0.764293771819342,0.242247017684031,
0.99097032381445));
#52816=CARTESIAN_POINT('Ctrl Pts',(-0.710683845299557,0.350842060800447,
0.987321144453415));
#52817=CARTESIAN_POINT('Ctrl Pts',(-0.652710599305326,0.468275669779912,
0.983374957869923));
#52818=CARTESIAN_POINT('Ctrl Pts',(-0.565008404019093,0.571033039869338,
0.979428771286432));
#52819=CARTESIAN_POINT('Ctrl Pts',(-0.458141477682844,0.646736473330992,
0.97548258470294));
#52820=CARTESIAN_POINT('Ctrl Pts',(-0.351274551346596,0.722439906792646,
0.971536398119448));
#52821=CARTESIAN_POINT('Ctrl Pts',(-0.225242893960332,0.771089403626528,
0.967590211535957));
#52822=CARTESIAN_POINT('Ctrl Pts',(-0.0952277211006728,0.786824860355167,
0.963644024952465));
#52823=CARTESIAN_POINT('Ctrl Pts',(0.0347874517589859,0.802560317083806,
0.959697838368973));
#52824=CARTESIAN_POINT('Ctrl Pts',(0.168786140092041,0.785381733707203,
0.955751651785481));
#52825=CARTESIAN_POINT('Ctrl Pts',(0.290627455022684,0.737358367191763,
0.951805465201989));
#52826=CARTESIAN_POINT('Ctrl Pts',(0.412468769953327,0.689335000676323,
0.947859278618497));
#52827=CARTESIAN_POINT('Ctrl Pts',(0.522152711481559,0.610466851022046,
0.943913092035006));
#52828=CARTESIAN_POINT('Ctrl Pts',(0.606467237537711,0.510254024749504,
0.939966905451514));
#52829=CARTESIAN_POINT('Ctrl Pts',(0.690781763593864,0.410041198476962,
0.936020718868022));
#52830=CARTESIAN_POINT('Ctrl Pts',(0.749726874177938,0.288483695586154,
0.93207453228453));
#52831=CARTESIAN_POINT('Ctrl Pts',(0.776202302140517,0.16022379814418,0.928128345701038));
#52832=CARTESIAN_POINT('Ctrl Pts',(0.802677730103097,0.0319639007022064,
0.924182159117547));
#52833=CARTESIAN_POINT('Ctrl Pts',(0.796683475444182,-0.102998391290932,
0.920235972534055));
#52834=CARTESIAN_POINT('Ctrl Pts',(0.758941579632242,-0.228406124124693,
0.916289785950564));
#52835=CARTESIAN_POINT('Ctrl Pts',(0.7211996838203,-0.353813856958455,0.912343599367072));
#52836=CARTESIAN_POINT('Ctrl Pts',(0.651710146855333,-0.469667030632837,
0.908397412783579));
#52837=CARTESIAN_POINT('Ctrl Pts',(0.558843370603139,-0.562010471638567,
0.904451226200087));
#52838=CARTESIAN_POINT('Ctrl Pts',(0.465976594350946,-0.654353912644296,
0.900505039616596));
#52839=CARTESIAN_POINT('Ctrl Pts',(0.349732578811529,-0.723187620981374,
0.896558853033105));
#52840=CARTESIAN_POINT('Ctrl Pts',(0.224113563887374,-0.760220218573038,
0.892612666449613));
#52841=CARTESIAN_POINT('Ctrl Pts',(0.0984945489632185,-0.797252816164703,
0.888666479866121));
#52842=CARTESIAN_POINT('Ctrl Pts',(-0.0364994653456741,-0.802484303010954,
0.884720293282628));
#52843=CARTESIAN_POINT('Ctrl Pts',(-0.164607698271848,-0.775284466464064,
0.880774106699137));
#52844=CARTESIAN_POINT('Ctrl Pts',(-0.292715931198022,-0.748084629917174,
0.876827920115645));
#52845=CARTESIAN_POINT('Ctrl Pts',(-0.413938382741478,-0.688453469977143,
0.872881733532154));
#52846=CARTESIAN_POINT('Ctrl Pts',(-0.513673131666121,-0.60357399285205,
0.868935546948662));
#52847=CARTESIAN_POINT('Ctrl Pts',(-0.613407880590764,-0.518694515726958,
0.86498936036517));
#52848=CARTESIAN_POINT('Ctrl Pts',(-0.691654926896594,-0.408566721416806,
0.861043173781678));
#52849=CARTESIAN_POINT('Ctrl Pts',(-0.738988980313063,-0.286455917591038,
0.857096987198186));
#52850=CARTESIAN_POINT('Ctrl Pts',(-0.774287146073082,-0.195394893160973,
0.854154218977631));
#52851=CARTESIAN_POINT('Ctrl Pts',(-0.792394438618434,-0.0976700559435039,
0.851211450757076));
#52852=CARTESIAN_POINT('Ctrl Pts',(-0.792490573374725,2.00326525206102E-5,
0.848268682536521));
#52853=CARTESIAN_POINT('Ctrl Pts',(-0.792490189019743,1.3140117316485E-5,
0.826731317463479));
#52854=CARTESIAN_POINT('Ctrl Pts',(-0.792394876538436,-0.0971903585595296,
0.829659438059461));
#52855=CARTESIAN_POINT('Ctrl Pts',(-0.774470502847006,-0.194422216474874,
0.832587558655444));
#52856=CARTESIAN_POINT('Ctrl Pts',(-0.739514560452847,-0.285092406647597,
0.835515679251426));
#52857=CARTESIAN_POINT('Ctrl Pts',(-0.69240493283764,-0.407287335529011,
0.839461865834918));
#52858=CARTESIAN_POINT('Ctrl Pts',(-0.61436159852265,-0.517564589124346,
0.843408052418409));
#52859=CARTESIAN_POINT('Ctrl Pts',(-0.514783468555716,-0.602628892990279,
0.847354239001901));
#52860=CARTESIAN_POINT('Ctrl Pts',(-0.415205338588783,-0.687693196856211,
0.851300425585393));
#52861=CARTESIAN_POINT('Ctrl Pts',(-0.294092412969906,-0.74754455099274,
0.855246612168885));
#52862=CARTESIAN_POINT('Ctrl Pts',(-0.166034353688321,-0.774979445676994,
0.859192798752377));
#52863=CARTESIAN_POINT('Ctrl Pts',(-0.0379762944067349,-0.802414340361247,
0.863138985335869));
#52864=CARTESIAN_POINT('Ctrl Pts',(0.0970268985375597,-0.797432775593224,
0.867085171919361));
#52865=CARTESIAN_POINT('Ctrl Pts',(0.222713811041056,-0.760631818600032,
0.871031358502853));
#52866=CARTESIAN_POINT('Ctrl Pts',(0.348400723544551,-0.723830861606839,
0.874977545086344));
#52867=CARTESIAN_POINT('Ctrl Pts',(0.464771355607247,-0.655210512388478,
0.878923731669835));
#52868=CARTESIAN_POINT('Ctrl Pts',(0.55780797689814,-0.563037985744865,
0.882869918253327));
#52869=CARTESIAN_POINT('Ctrl Pts',(0.650844598189034,-0.470865459101252,
0.886816104836819));
#52870=CARTESIAN_POINT('Ctrl Pts',(0.720547208708123,-0.355140755032387,
0.890762291420312));
#52871=CARTESIAN_POINT('Ctrl Pts',(0.758519861389888,-0.229802795205853,
0.894708478003803));
#52872=CARTESIAN_POINT('Ctrl Pts',(0.796492514071653,-0.104464835379319,
0.898654664587295));
#52873=CARTESIAN_POINT('Ctrl Pts',(0.802735208916092,0.0304863802048845,
0.902600851170786));
#52874=CARTESIAN_POINT('Ctrl Pts',(0.77649591743639,0.158794839290955,0.906547037754278));
#52875=CARTESIAN_POINT('Ctrl Pts',(0.750256625956688,0.287103298377025,
0.910493224337769));
#52876=CARTESIAN_POINT('Ctrl Pts',(0.691535348152843,0.408769000964962,
0.914439410921262));
#52877=CARTESIAN_POINT('Ctrl Pts',(0.607405420110863,0.509136830275265,
0.918385597504753));
#52878=CARTESIAN_POINT('Ctrl Pts',(0.523275492068883,0.609504659585568,
0.922331784088245));
#52879=CARTESIAN_POINT('Ctrl Pts',(0.413736913788769,0.688574615618236,
0.926277970671737));
#52880=CARTESIAN_POINT('Ctrl Pts',(0.29198420193571,0.736822182783594,0.930224157255229));
#52881=CARTESIAN_POINT('Ctrl Pts',(0.170231490082652,0.785069749948953,
0.93417034383872));
#52882=CARTESIAN_POINT('Ctrl Pts',(0.0362646446566508,0.802494928247001,
0.938116530422213));
#52883=CARTESIAN_POINT('Ctrl Pts',(-0.093779273240774,0.786998807714651,
0.942062717005704));
#52884=CARTESIAN_POINT('Ctrl Pts',(-0.2238231911382,0.771502687182301,0.946008903589196));
#52885=CARTESIAN_POINT('Ctrl Pts',(-0.34994418150705,0.723085267819551,
0.949955090172688));
#52886=CARTESIAN_POINT('Ctrl Pts',(-0.456950272099103,0.647578672431404,
0.953901276756179));
#52887=CARTESIAN_POINT('Ctrl Pts',(-0.563956362691155,0.572072077043258,
0.957847463339671));
#52888=CARTESIAN_POINT('Ctrl Pts',(-0.65184755350641,0.469476305629716,
0.961793649923163));
#52889=CARTESIAN_POINT('Ctrl Pts',(-0.710036858724068,0.352149603432412,
0.965739836506655));
#52890=CARTESIAN_POINT('Ctrl Pts',(-0.764062572465559,0.243217922543028,
0.969403663492263));
#52891=CARTESIAN_POINT('Ctrl Pts',(-0.792484823565687,0.121587962456681,
0.973067490477871));
#52892=CARTESIAN_POINT('Ctrl Pts',(-0.792557287165952,-9.28448389212729E-6,
0.97673131746348));
#52893=CARTESIAN_POINT('Origin',(0.,0.,1.095));
#52894=CARTESIAN_POINT('',(-0.792443402549405,-1.07763833267771E-5,1.14826868253652));
#52895=CARTESIAN_POINT('',(-0.792444147951047,-1.11489312963033E-5,1.12673131746348));
#52896=CARTESIAN_POINT('',(-0.7925,-9.70532588324277E-17,1.095));
#52897=CARTESIAN_POINT('Ctrl Pts',(-0.792443402549405,-1.07763833267771E-5,
1.14826868253652));
#52898=CARTESIAN_POINT('Ctrl Pts',(-0.792405491575818,0.0779733200496504,
1.14591992876088));
#52899=CARTESIAN_POINT('Ctrl Pts',(-0.780968401909595,0.1559682971011,1.14357117498524));
#52900=CARTESIAN_POINT('Ctrl Pts',(-0.758294050000535,0.230546770333913,
1.14122242120959));
#52901=CARTESIAN_POINT('Ctrl Pts',(-0.720198433414051,0.355847503659272,
1.1372762346261));
#52902=CARTESIAN_POINT('Ctrl Pts',(-0.650382262731333,0.47150412689294,
1.13333004804261));
#52903=CARTESIAN_POINT('Ctrl Pts',(-0.557255284838512,0.563585155142655,
1.12938386145912));
#52904=CARTESIAN_POINT('Ctrl Pts',(-0.464128306945689,0.65566618339237,
1.12543767487563));
#52905=CARTESIAN_POINT('Ctrl Pts',(-0.347690521842762,0.724171616658134,
1.12149148829214));
#52906=CARTESIAN_POINT('Ctrl Pts',(-0.221967509722995,0.760849593681277,
1.11754530170864));
#52907=CARTESIAN_POINT('Ctrl Pts',(-0.0962444976032272,0.797527570704419,
1.11359911512515));
#52908=CARTESIAN_POINT('Ctrl Pts',(0.0387637415333804,0.802378091484939,
1.10965292854166));
#52909=CARTESIAN_POINT('Ctrl Pts',(0.16679471280093,0.774816883759842,1.10570674195817));
#52910=CARTESIAN_POINT('Ctrl Pts',(0.294825684068478,0.747255676034745,
1.10176055537468));
#52911=CARTESIAN_POINT('Ctrl Pts',(0.415879387466968,0.687282739804032,
1.09781436879119));
#52912=CARTESIAN_POINT('Ctrl Pts',(0.515374229717151,0.602122149502075,
1.09386818220769));
#52913=CARTESIAN_POINT('Ctrl Pts',(0.614869071967334,0.516961559200118,
1.0899219956242));
#52914=CARTESIAN_POINT('Ctrl Pts',(0.69280505306921,0.406613314826917,1.08597580904071));
#52915=CARTESIAN_POINT('Ctrl Pts',(0.739794349715095,0.284369477453707,
1.08202962245722));
#52916=CARTESIAN_POINT('Ctrl Pts',(0.78678364636098,0.162125640080496,1.07808343587373));
#52917=CARTESIAN_POINT('Ctrl Pts',(0.802826258550874,0.0279862097072739,
1.07413724929023));
#52918=CARTESIAN_POINT('Ctrl Pts',(0.785989764231391,-0.101890971637066,
1.07019106270674));
#52919=CARTESIAN_POINT('Ctrl Pts',(0.769153269911908,-0.231768152981406,
1.06624487612325));
#52920=CARTESIAN_POINT('Ctrl Pts',(0.719437669083049,-0.357383085296865,
1.06229868953976));
#52921=CARTESIAN_POINT('Ctrl Pts',(0.642831482959536,-0.463604749860529,
1.05835250295627));
#52922=CARTESIAN_POINT('Ctrl Pts',(0.566225296836024,-0.569826414424192,
1.05440631637278));
#52923=CARTESIAN_POINT('Ctrl Pts',(0.462728525417858,-0.656654811236061,
1.05046012978928));
#52924=CARTESIAN_POINT('Ctrl Pts',(0.344807931671896,-0.71363097594976,
1.04651394320579));
#52925=CARTESIAN_POINT('Ctrl Pts',(0.226887337925933,-0.770607140663459,
1.0425677566223));
#52926=CARTESIAN_POINT('Ctrl Pts',(0.0945429218521742,-0.79773107327899,
1.03862157003881));
#52927=CARTESIAN_POINT('Ctrl Pts',(-0.0362836939983929,-0.79173554494208,
1.03467538345532));
#52928=CARTESIAN_POINT('Ctrl Pts',(-0.167110309848962,-0.78574001660517,
1.03072919687183));
#52929=CARTESIAN_POINT('Ctrl Pts',(-0.296419125476338,-0.746625027315819,
1.02678301028833));
#52930=CARTESIAN_POINT('Ctrl Pts',(-0.4086341733228,-0.679102195530961,
1.02283682370484));
#52931=CARTESIAN_POINT('Ctrl Pts',(-0.52084922116926,-0.611579363746103,
1.01889063712135));
#52932=CARTESIAN_POINT('Ctrl Pts',(-0.615970501234805,-0.515648689465738,
1.01494445053786));
#52933=CARTESIAN_POINT('Ctrl Pts',(-0.682540125167227,-0.40286555711433,
1.01099826395437));
#52934=CARTESIAN_POINT('Ctrl Pts',(-0.74910974909965,-0.290082424762922,
1.00705207737087));
#52935=CARTESIAN_POINT('Ctrl Pts',(-0.787127716898949,-0.160446834340471,
1.00310589078738));
#52936=CARTESIAN_POINT('Ctrl Pts',(-0.792014552447484,-0.0295741151944942,
0.999159704203891));
#52937=CARTESIAN_POINT('Ctrl Pts',(-0.79238235701581,-0.0197240632553592,
0.998862696981434));
#52938=CARTESIAN_POINT('Ctrl Pts',(-0.792562482849181,-0.00986700332289492,
0.998565689758977));
#52939=CARTESIAN_POINT('Ctrl Pts',(-0.792556380474703,-9.7200913266593E-6,
0.99826868253652));
#52940=CARTESIAN_POINT('Ctrl Pts',(-0.792557287165952,-9.28448389212729E-6,
0.97673131746348));
#52941=CARTESIAN_POINT('Ctrl Pts',(-0.792562871707229,-0.00938040104719254,
0.977013677061363));
#52942=CARTESIAN_POINT('Ctrl Pts',(-0.792400078381659,-0.0187513233173363,
0.977296036659247));
#52943=CARTESIAN_POINT('Ctrl Pts',(-0.792067650133023,-0.0281162240255477,
0.97757839625713));
#52944=CARTESIAN_POINT('Ctrl Pts',(-0.787421716704263,-0.158997716305135,
0.981524582840622));
#52945=CARTESIAN_POINT('Ctrl Pts',(-0.749642430226683,-0.288703067883244,
0.985470769424114));
#52946=CARTESIAN_POINT('Ctrl Pts',(-0.683280515807775,-0.401608542979231,
0.989416956007606));
#52947=CARTESIAN_POINT('Ctrl Pts',(-0.616918601388867,-0.514514018075219,
0.993363142591098));
#52948=CARTESIAN_POINT('Ctrl Pts',(-0.521974059028629,-0.610619616689085,
0.997309329174589));
#52949=CARTESIAN_POINT('Ctrl Pts',(-0.409883488297753,-0.678348885460243,
1.00125551575808));
#52950=CARTESIAN_POINT('Ctrl Pts',(-0.297792917566875,-0.746078154231402,
1.00520170234157));
#52951=CARTESIAN_POINT('Ctrl Pts',(-0.16855631846536,-0.785431093159854,
1.00914788892507));
#52952=CARTESIAN_POINT('Ctrl Pts',(-0.0377409595363729,-0.791667420581768,
1.01309407550856));
#52953=CARTESIAN_POINT('Ctrl Pts',(0.0930743993926127,-0.797903748003683,
1.01704026209205));
#52954=CARTESIAN_POINT('Ctrl Pts',(0.225468518149069,-0.771023463919061,
1.02098644867554));
#52955=CARTESIAN_POINT('Ctrl Pts',(0.343493787150374,-0.714264448786606,
1.02493263525903));
#52956=CARTESIAN_POINT('Ctrl Pts',(0.461519056151679,-0.657505433654151,
1.02887882184252));
#52957=CARTESIAN_POINT('Ctrl Pts',(0.565175475397833,-0.570867687473863,
1.03282500842602));
#52958=CARTESIAN_POINT('Ctrl Pts',(0.641977051484891,-0.464787209444585,
1.03677119500951));
#52959=CARTESIAN_POINT('Ctrl Pts',(0.71877862757195,-0.358706731415306,
1.040717381593));
#52960=CARTESIAN_POINT('Ctrl Pts',(0.768725360499914,-0.233183521537036,
1.04466356817649));
#52961=CARTESIAN_POINT('Ctrl Pts',(0.785800887887494,-0.103337550163271,
1.04860975475998));
#52962=CARTESIAN_POINT('Ctrl Pts',(0.802876415275075,0.0265084212104935,
1.05255594134347));
#52963=CARTESIAN_POINT('Ctrl Pts',(0.787080737122274,0.160677154079753,
1.05650212792697));
#52964=CARTESIAN_POINT('Ctrl Pts',(0.740316530909984,0.283007276821933,
1.06044831451046));
#52965=CARTESIAN_POINT('Ctrl Pts',(0.693552324697694,0.405337399564113,
1.06439450109395));
#52966=CARTESIAN_POINT('Ctrl Pts',(0.615819590425917,0.515828912179213,
1.06834068767744));
#52967=CARTESIAN_POINT('Ctrl Pts',(0.516481669184491,0.601172496109797,
1.07228687426093));
#52968=CARTESIAN_POINT('Ctrl Pts',(0.417143747943065,0.686516080040382,
1.07623306084442));
#52969=CARTESIAN_POINT('Ctrl Pts',(0.296200639731992,0.74671173528645,1.08017924742792));
#52970=CARTESIAN_POINT('Ctrl Pts',(0.168220616025976,0.774508559681008,
1.08412543401141));
#52971=CARTESIAN_POINT('Ctrl Pts',(0.0402405923199609,0.802305384075567,
1.0880716205949));
#52972=CARTESIAN_POINT('Ctrl Pts',(-0.0947763468809948,0.797703377618616,
1.09201780717839));
#52973=CARTESIAN_POINT('Ctrl Pts',(-0.220566658720863,0.761256877630617,
1.09596399376188));
#52974=CARTESIAN_POINT('Ctrl Pts',(-0.34635697056073,0.724810377642619,
1.09991018034538));
#52975=CARTESIAN_POINT('Ctrl Pts',(-0.462920655039508,0.656519384123574,
1.10385636692887));
#52976=CARTESIAN_POINT('Ctrl Pts',(-0.556216966681838,0.564609927873067,
1.10780255351236));
#52977=CARTESIAN_POINT('Ctrl Pts',(-0.649513278324167,0.47270047162256,
1.11174874009585));
#52978=CARTESIAN_POINT('Ctrl Pts',(-0.719542217130047,0.35717255264059,
1.11569492667934));
#52979=CARTESIAN_POINT('Ctrl Pts',(-0.757868407107316,0.231942152673131,
1.11964111326283));
#52980=CARTESIAN_POINT('Ctrl Pts',(-0.780822256131107,0.156940705992757,
1.12200451466305));
#52981=CARTESIAN_POINT('Ctrl Pts',(-0.792404633700123,0.0784590725890344,
1.12436791606326));
#52982=CARTESIAN_POINT('Ctrl Pts',(-0.792444147951047,-1.11489312963033E-5,
1.12673131746348));
#52983=CARTESIAN_POINT('Origin',(0.,0.,1.095));
#52984=CARTESIAN_POINT('',(-0.792486097671081,1.97476927368961E-5,1.29826868253652));
#52985=CARTESIAN_POINT('',(-0.792484660449143,1.96714801883982E-5,1.27673131746348));
#52986=CARTESIAN_POINT('',(-0.7925,-9.70532588324277E-17,1.095));
#52987=CARTESIAN_POINT('Ctrl Pts',(-0.792486097671081,1.97476927368961E-5,
1.29826868253652));
#52988=CARTESIAN_POINT('Ctrl Pts',(-0.792519712746547,0.0348213055222317,
1.29722035434627));
#52989=CARTESIAN_POINT('Ctrl Pts',(-0.790269179267766,0.0696185478218366,
1.29617202615602));
#52990=CARTESIAN_POINT('Ctrl Pts',(-0.785699122793507,0.104108443553474,
1.29512369796577));
#52991=CARTESIAN_POINT('Ctrl Pts',(-0.76849621275801,0.233937599220784,
1.29117751138228));
#52992=CARTESIAN_POINT('Ctrl Pts',(-0.718426354171464,0.359411745751982,
1.28723132479879));
#52993=CARTESIAN_POINT('Ctrl Pts',(-0.641520740569973,0.465416822854705,
1.2832851382153));
#52994=CARTESIAN_POINT('Ctrl Pts',(-0.564615126968481,0.571421899957427,
1.27933895163181));
#52995=CARTESIAN_POINT('Ctrl Pts',(-0.460873758352043,0.657957907631675,
1.27539276504832));
#52996=CARTESIAN_POINT('Ctrl Pts',(-0.342792860783382,0.71460110143601,
1.27144657846482));
#52997=CARTESIAN_POINT('Ctrl Pts',(-0.224711963214721,0.771244295240344,
1.26750039188133));
#52998=CARTESIAN_POINT('Ctrl Pts',(-0.0922915366938353,0.797994675174765,
1.26355420529784));
#52999=CARTESIAN_POINT('Ctrl Pts',(0.0385176403463696,0.79163000888026,
1.25960801871435));
#53000=CARTESIAN_POINT('Ctrl Pts',(0.169326817386578,0.785265342585755,
1.25566183213086));
#53001=CARTESIAN_POINT('Ctrl Pts',(0.298524744946107,0.745785630062321,
1.25171564554737));
#53002=CARTESIAN_POINT('Ctrl Pts',(0.410548812552865,0.677946422727524,
1.24776945896387));
#53003=CARTESIAN_POINT('Ctrl Pts',(0.522572880159619,0.610107215392729,
1.24382327238038));
#53004=CARTESIAN_POINT('Ctrl Pts',(0.617423087813604,0.513908513246573,
1.23987708579689));
#53005=CARTESIAN_POINT('Ctrl Pts',(0.683674199345799,0.400937986135629,
1.2359308992134));
#53006=CARTESIAN_POINT('Ctrl Pts',(0.749925310877995,0.287967459024683,
1.2319847126299));
#53007=CARTESIAN_POINT('Ctrl Pts',(0.787577326288399,0.158225106948951,
1.22803852604641));
#53008=CARTESIAN_POINT('Ctrl Pts',(0.792094850463563,0.0273391193478977,
1.22409233946292));
#53009=CARTESIAN_POINT('Ctrl Pts',(0.796612374638728,-0.103546868253156,
1.22014615287943));
#53010=CARTESIAN_POINT('Ctrl Pts',(0.767995407578652,-0.235576491379531,
1.21619996629594));
#53011=CARTESIAN_POINT('Ctrl Pts',(0.709691022465244,-0.352846046045368,
1.21225377971245));
#53012=CARTESIAN_POINT('Ctrl Pts',(0.651386637351836,-0.470115600711205,
1.20830759312896));
#53013=CARTESIAN_POINT('Ctrl Pts',(0.563394834185097,-0.572625086916506,
1.20436140654546));
#53014=CARTESIAN_POINT('Ctrl Pts',(0.456314716087557,-0.648026665700992,
1.20041521996197));
#53015=CARTESIAN_POINT('Ctrl Pts',(0.349234597990017,-0.723428244485478,
1.19646903337848));
#53016=CARTESIAN_POINT('Ctrl Pts',(0.223066164961679,-0.771721915849148,
1.19252284679499));
#53017=CARTESIAN_POINT('Ctrl Pts',(0.0930071079731554,-0.787090437906651,
1.1885766602115));
#53018=CARTESIAN_POINT('Ctrl Pts',(-0.0370519490153704,-0.802458959964154,
1.184630473628));
#53019=CARTESIAN_POINT('Ctrl Pts',(-0.17100162996408,-0.784902332715489,
1.18068428704451));
#53020=CARTESIAN_POINT('Ctrl Pts',(-0.292706949220785,-0.736535349766373,
1.17673810046102));
#53021=CARTESIAN_POINT('Ctrl Pts',(-0.414412268477487,-0.688168366817258,
1.17279191387753));
#53022=CARTESIAN_POINT('Ctrl Pts',(-0.523873226042186,-0.608991028167693,
1.16884572729404));
#53023=CARTESIAN_POINT('Ctrl Pts',(-0.60790463948464,-0.508540685560815,
1.16489954071055));
#53024=CARTESIAN_POINT('Ctrl Pts',(-0.691936052927096,-0.408090342953935,
1.16095335412705));
#53025=CARTESIAN_POINT('Ctrl Pts',(-0.750537922247308,-0.28636699638974,
1.15700716754356));
#53026=CARTESIAN_POINT('Ctrl Pts',(-0.776651325662288,-0.158032901399117,
1.15306098096007));
#53027=CARTESIAN_POINT('Ctrl Pts',(-0.787222140411448,-0.106082723837479,
1.15146354815222));
#53028=CARTESIAN_POINT('Ctrl Pts',(-0.792469186534774,-0.0530492665922584,
1.14986611534437));
#53029=CARTESIAN_POINT('Ctrl Pts',(-0.792443402549405,-1.07763833267771E-5,
1.14826868253652));
#53030=CARTESIAN_POINT('Ctrl Pts',(-0.792444147951047,-1.11489312963033E-5,
1.12673131746348));
#53031=CARTESIAN_POINT('Ctrl Pts',(-0.79247061090012,-0.0525631631340214,
1.12831410264676));
#53032=CARTESIAN_POINT('Ctrl Pts',(-0.787320021835728,-0.105110059030113,
1.12989688783003));
#53033=CARTESIAN_POINT('Ctrl Pts',(-0.776940900150374,-0.15660307261215,
1.13147967301331));
#53034=CARTESIAN_POINT('Ctrl Pts',(-0.751063762067508,-0.284985016977022,
1.1354258595968));
#53035=CARTESIAN_POINT('Ctrl Pts',(-0.692686044753119,-0.406816024753814,
1.13937204618029));
#53036=CARTESIAN_POINT('Ctrl Pts',(-0.608839669631833,-0.507420872018991,
1.14331823276378));
#53037=CARTESIAN_POINT('Ctrl Pts',(-0.524993294510546,-0.608025719284169,
1.14726441934728));
#53038=CARTESIAN_POINT('Ctrl Pts',(-0.415678261582362,-0.68740440603773,
1.15121060593077));
#53039=CARTESIAN_POINT('Ctrl Pts',(-0.294062175841689,-0.735995327034944,
1.15515679251426));
#53040=CARTESIAN_POINT('Ctrl Pts',(-0.172446090101016,-0.784586248032158,
1.15910297909775));
#53041=CARTESIAN_POINT('Ctrl Pts',(-0.0385289515478548,-0.802389403273024,
1.16304916568124));
#53042=CARTESIAN_POINT('Ctrl Pts',(0.0915581740785099,-0.787260303481235,
1.16699535226474));
#53043=CARTESIAN_POINT('Ctrl Pts',(0.221645299704875,-0.772131203689446,
1.17094153884823));
#53044=CARTESIAN_POINT('Ctrl Pts',(0.347902412404443,-0.724069848865002,
1.17488772543172));
#53045=CARTESIAN_POINT('Ctrl Pts',(0.455121139245943,-0.648865497071205,
1.17883391201521));
#53046=CARTESIAN_POINT('Ctrl Pts',(0.562339866087442,-0.573661145277409,
1.1827800985987));
#53047=CARTESIAN_POINT('Ctrl Pts',(0.650520207070873,-0.471313796514261,
1.1867262851822));
#53048=CARTESIAN_POINT('Ctrl Pts',(0.709040348642845,-0.354151759383475,
1.19067247176569));
#53049=CARTESIAN_POINT('Ctrl Pts',(0.767560490214817,-0.236989722252689,
1.19461865834918));
#53050=CARTESIAN_POINT('Ctrl Pts',(0.796420432375329,-0.105012996754264,
1.19856484493267));
#53051=CARTESIAN_POINT('Ctrl Pts',(0.792143834237383,0.0258810849400756,
1.20251103151616));
#53052=CARTESIAN_POINT('Ctrl Pts',(0.787867236099438,0.156775166634416,
1.20645721809965));
#53053=CARTESIAN_POINT('Ctrl Pts',(0.750454097663033,0.286586604524672,
1.21040340468315));
#53054=CARTESIAN_POINT('Ctrl Pts',(0.684411039978694,0.39967888739995,1.21434959126664));
#53055=CARTESIAN_POINT('Ctrl Pts',(0.618367982294357,0.512771170275227,
1.21829577785013));
#53056=CARTESIAN_POINT('Ctrl Pts',(0.523695005362085,0.609144298135527,
1.22224196443362));
#53057=CARTESIAN_POINT('Ctrl Pts',(0.411795996922659,0.677189590584832,
1.22618815101711));
#53058=CARTESIAN_POINT('Ctrl Pts',(0.299896988483233,0.745234883034137,
1.2301343376006));
#53059=CARTESIAN_POINT('Ctrl Pts',(0.170771948536651,0.784952340072448,
1.2340805241841));
#53060=CARTESIAN_POINT('Ctrl Pts',(0.0399747078357781,0.791557772630288,
1.23802671076759));
#53061=CARTESIAN_POINT('Ctrl Pts',(-0.0908225328650967,0.798163205188129,
1.24197289735108));
#53062=CARTESIAN_POINT('Ctrl Pts',(-0.223291974320261,0.771656613265497,
1.24591908393457));
#53063=CARTESIAN_POINT('Ctrl Pts',(-0.341476933974791,0.715230863596611,
1.24986527051806));
#53064=CARTESIAN_POINT('Ctrl Pts',(-0.459661893629321,0.658805113927726,
1.25381145710156));
#53065=CARTESIAN_POINT('Ctrl Pts',(-0.563562371483215,0.572460206512586,
1.25775764368505));
#53066=CARTESIAN_POINT('Ctrl Pts',(-0.640662975879288,0.466596866701304,
1.26170383026854));
#53067=CARTESIAN_POINT('Ctrl Pts',(-0.717763580275359,0.360733526890024,
1.26565001685203));
#53068=CARTESIAN_POINT('Ctrl Pts',(-0.76806431121361,0.235351754682601,
1.26959620343552));
#53069=CARTESIAN_POINT('Ctrl Pts',(-0.785506165296385,0.105554483369243,
1.27354239001901));
#53070=CARTESIAN_POINT('Ctrl Pts',(-0.790204440115218,0.0705912708305541,
1.27460536583384));
#53071=CARTESIAN_POINT('Ctrl Pts',(-0.792518506333689,0.0353076739102088,
1.27566834164866));
#53072=CARTESIAN_POINT('Ctrl Pts',(-0.792484660449143,1.96714801883982E-5,
1.27673131746348));
#53073=CARTESIAN_POINT('Origin',(0.,0.,1.095));
#53074=CARTESIAN_POINT('',(-0.79255903846122,-8.36642852242164E-6,1.44826868253652));
#53075=CARTESIAN_POINT('',(-0.792559834217432,-7.91270320494323E-6,1.42673131746348));
#53076=CARTESIAN_POINT('',(-0.7925,-9.70532588324277E-17,1.095));
#53077=CARTESIAN_POINT('Ctrl Pts',(-0.79255903846122,-8.36642852242164E-6,
1.44826868253652));
#53078=CARTESIAN_POINT('Ctrl Pts',(-0.792492123018653,0.122592452217723,
1.44457459334817));
#53079=CARTESIAN_POINT('Ctrl Pts',(-0.763581778346857,0.245223739974001,
1.44088050415983));
#53080=CARTESIAN_POINT('Ctrl Pts',(-0.708692548810537,0.354847221826574,
1.43718641497148));
#53081=CARTESIAN_POINT('Ctrl Pts',(-0.650057488818566,0.471951788410097,
1.43324022838799));
#53082=CARTESIAN_POINT('Ctrl Pts',(-0.561776778393065,0.574212574410295,
1.42929404180449));
#53083=CARTESIAN_POINT('Ctrl Pts',(-0.454484321146134,0.649311698192748,
1.425347855221));
#53084=CARTESIAN_POINT('Ctrl Pts',(-0.347191863899205,0.7244108219752,1.42140166863751));
#53085=CARTESIAN_POINT('Ctrl Pts',(-0.220887659830848,0.772348283539907,
1.41745548205402));
#53086=CARTESIAN_POINT('Ctrl Pts',(-0.0907857542901829,0.787349748457175,
1.41350929547053));
#53087=CARTESIAN_POINT('Ctrl Pts',(0.0393161512504821,0.802351213374442,
1.40956310888704));
#53088=CARTESIAN_POINT('Ctrl Pts',(0.173215758263455,0.784416681644269,
1.40561692230354));
#53089=CARTESIAN_POINT('Ctrl Pts',(0.294784112781199,0.735706467573458,
1.40167073572005));
#53090=CARTESIAN_POINT('Ctrl Pts',(0.416352467298942,0.686996253502646,
1.39772454913656));
#53091=CARTESIAN_POINT('Ctrl Pts',(0.525589569321458,0.607510357091197,
1.39377836255307));
#53092=CARTESIAN_POINT('Ctrl Pts',(0.609337201066242,0.506823297584445,
1.38983217596958));
#53093=CARTESIAN_POINT('Ctrl Pts',(0.693084832811026,0.406136238077694,
1.38588598938608));
#53094=CARTESIAN_POINT('Ctrl Pts',(0.751342994278079,0.28424801547564,1.38193980280259));
#53095=CARTESIAN_POINT('Ctrl Pts',(0.777094165211017,0.155840745546875,
1.3779936162191));
#53096=CARTESIAN_POINT('Ctrl Pts',(0.802845336143955,0.02743347561811,1.37404742963561));
#53097=CARTESIAN_POINT('Ctrl Pts',(0.796089516542778,-0.107492841637366,
1.37010124305212));
#53098=CARTESIAN_POINT('Ctrl Pts',(0.757640482532682,-0.232685579280836,
1.36615505646863));
#53099=CARTESIAN_POINT('Ctrl Pts',(0.719191448522586,-0.357878316924306,
1.36220886988514));
#53100=CARTESIAN_POINT('Ctrl Pts',(0.649049200103572,-0.473337474955769,
1.35826268330164));
#53101=CARTESIAN_POINT('Ctrl Pts',(0.555662762042532,-0.565155354267195,
1.35431649671815));
#53102=CARTESIAN_POINT('Ctrl Pts',(0.46227632398149,-0.656973233578622,
1.35037031013466));
#53103=CARTESIAN_POINT('Ctrl Pts',(0.345645696278421,-0.725149834170012,
1.34642412355117));
#53104=CARTESIAN_POINT('Ctrl Pts',(0.219819688092605,-0.761472904511042,
1.34247793696768));
#53105=CARTESIAN_POINT('Ctrl Pts',(0.0939936799067887,-0.797795974852073,
1.33853175038418));
#53106=CARTESIAN_POINT('Ctrl Pts',(-0.0410277087617754,-0.802265514942745,
1.33458556380069));
#53107=CARTESIAN_POINT('Ctrl Pts',(-0.168980399092773,-0.77434314376771,
1.3306393772172));
#53108=CARTESIAN_POINT('Ctrl Pts',(-0.296933089423769,-0.746420772592674,
1.32669319063371));
#53109=CARTESIAN_POINT('Ctrl Pts',(-0.417817081417198,-0.686106490151933,
1.32274700405022));
#53110=CARTESIAN_POINT('Ctrl Pts',(-0.517071224478458,-0.600665487933144,
1.31880081746672));
#53111=CARTESIAN_POINT('Ctrl Pts',(-0.616325367539718,-0.515224485714355,
1.31485463088323));
#53112=CARTESIAN_POINT('Ctrl Pts',(-0.693949661668808,-0.404656763717519,
1.31090844429974));
#53113=CARTESIAN_POINT('Ctrl Pts',(-0.74059382799113,-0.282280820317389,
1.30696225771625));
#53114=CARTESIAN_POINT('Ctrl Pts',(-0.774846691106731,-0.192414782001653,
1.30406439932301));
#53115=CARTESIAN_POINT('Ctrl Pts',(-0.79239317664741,-0.0961810293084249,
1.30116654092976));
#53116=CARTESIAN_POINT('Ctrl Pts',(-0.792486097671081,1.97476927368961E-5,
1.29826868253652));
#53117=CARTESIAN_POINT('Ctrl Pts',(-0.792484660449143,1.96714801883982E-5,
1.27673131746348));
#53118=CARTESIAN_POINT('Ctrl Pts',(-0.792392857025736,-0.0956953459194891,
1.27961452823215));
#53119=CARTESIAN_POINT('Ctrl Pts',(-0.775027255054072,-0.191442775046391,
1.28249773900082));
#53120=CARTESIAN_POINT('Ctrl Pts',(-0.741112163299563,-0.280917151643365,
1.28538094976949));
#53121=CARTESIAN_POINT('Ctrl Pts',(-0.69469332999267,-0.40337874492332,
1.28932713635298));
#53122=CARTESIAN_POINT('Ctrl Pts',(-0.617272686151585,-0.514089161063939,
1.29327332293647));
#53123=CARTESIAN_POINT('Ctrl Pts',(-0.518175979838655,-0.599712713385525,
1.29721950951997));
#53124=CARTESIAN_POINT('Ctrl Pts',(-0.419079273525725,-0.685336265707111,
1.30116569610346));
#53125=CARTESIAN_POINT('Ctrl Pts',(-0.298306504740949,-0.745872954209667,
1.30511188268695));
#53126=CARTESIAN_POINT('Ctrl Pts',(-0.170405426623534,-0.774030797355784,
1.30905806927044));
#53127=CARTESIAN_POINT('Ctrl Pts',(-0.042504348506119,-0.802188640501901,
1.31300425585393));
#53128=CARTESIAN_POINT('Ctrl Pts',(0.0925250389439315,-0.79796763829158,
1.31695044243742));
#53129=CARTESIAN_POINT('Ctrl Pts',(0.218417693408498,-0.761876233967231,
1.32089662902092));
#53130=CARTESIAN_POINT('Ctrl Pts',(0.344310347873065,-0.725784829642882,
1.32484281560441));
#53131=CARTESIAN_POINT('Ctrl Pts',(0.461066269352145,-0.657823023204503,
1.3287890021879));
#53132=CARTESIAN_POINT('Ctrl Pts',(0.5546215563528,-0.566177193029512,1.33273518877139));
#53133=CARTESIAN_POINT('Ctrl Pts',(0.648176843353457,-0.474531362854518,
1.33668137535488));
#53134=CARTESIAN_POINT('Ctrl Pts',(0.718531495875688,-0.359201508942911,
1.34062756193837));
#53135=CARTESIAN_POINT('Ctrl Pts',(0.757210903894515,-0.234079755000792,
1.34457374852187));
#53136=CARTESIAN_POINT('Ctrl Pts',(0.795890311913341,-0.108958001058676,
1.34851993510536));
#53137=CARTESIAN_POINT('Ctrl Pts',(0.802894475428763,0.0259556529139527,
1.35246612168885));
#53138=CARTESIAN_POINT('Ctrl Pts',(0.777379703906943,0.15441010534137,1.35641230827234));
#53139=CARTESIAN_POINT('Ctrl Pts',(0.751864932385123,0.282864557768787,
1.36035849485583));
#53140=CARTESIAN_POINT('Ctrl Pts',(0.693831225826063,0.404859808650995,
1.36430468143932));
#53141=CARTESIAN_POINT('Ctrl Pts',(0.610269067641456,0.505700850066526,
1.36825086802282));
#53142=CARTESIAN_POINT('Ctrl Pts',(0.526706909456849,0.606541891482058,
1.37219705460631));
#53143=CARTESIAN_POINT('Ctrl Pts',(0.417616299646695,0.686228723430912,
1.3761432411898));
#53144=CARTESIAN_POINT('Ctrl Pts',(0.296137810190029,0.735162622862339,
1.38008942777329));
#53145=CARTESIAN_POINT('Ctrl Pts',(0.174659320733361,0.784096522293767,
1.38403561435679));
#53146=CARTESIAN_POINT('Ctrl Pts',(0.0407929516301808,0.802277489207765,
1.38798180094028));
#53147=CARTESIAN_POINT('Ctrl Pts',(-0.0893363468434648,0.78751552480611,
1.39192798752377));
#53148=CARTESIAN_POINT('Ctrl Pts',(-0.219465645317109,0.772753560404456,
1.39587417410726));
#53149=CARTESIAN_POINT('Ctrl Pts',(-0.345857873161221,0.725048664687147,
1.39982036069075));
#53150=CARTESIAN_POINT('Ctrl Pts',(-0.453288382072276,0.650147158231332,
1.40376654727424));
#53151=CARTESIAN_POINT('Ctrl Pts',(-0.56071889098333,0.575245651775519,
1.40771273385774));
#53152=CARTESIAN_POINT('Ctrl Pts',(-0.64918768096133,0.473147534581201,
1.41165892044123));
#53153=CARTESIAN_POINT('Ctrl Pts',(-0.708038193163794,0.356151093918478,
1.41560510702472));
#53154=CARTESIAN_POINT('Ctrl Pts',(-0.763347554859349,0.24619455808673,
1.41931384383764));
#53155=CARTESIAN_POINT('Ctrl Pts',(-0.792495780424916,0.123078679523467,
1.42302258065056));
#53156=CARTESIAN_POINT('Ctrl Pts',(-0.792559834217432,-7.91270320494323E-6,
1.42673131746348));
#53157=CARTESIAN_POINT('Origin',(0.,0.,1.095));
#53158=CARTESIAN_POINT('',(-0.792445760035067,-1.19013985881156E-5,1.59826868253652));
#53159=CARTESIAN_POINT('',(-0.792446584180059,-1.22568943931671E-5,1.57673131746348));
#53160=CARTESIAN_POINT('',(-0.7925,-9.70532588324277E-17,1.095));
#53161=CARTESIAN_POINT('Ctrl Pts',(-0.792445760035067,-1.19013985881156E-5,
1.59826868253652));
#53162=CARTESIAN_POINT('Ctrl Pts',(-0.792402924653838,0.079462628716892,
1.59587501893357));
#53163=CARTESIAN_POINT('Ctrl Pts',(-0.780517347576401,0.158949689219715,
1.59348135533061));
#53164=CARTESIAN_POINT('Ctrl Pts',(-0.756980882452868,0.234822535499662,
1.59108769172766));
#53165=CARTESIAN_POINT('Ctrl Pts',(-0.718178737164498,0.359906280630659,
1.58714150514417));
#53166=CARTESIAN_POINT('Ctrl Pts',(-0.647710969507546,0.475167054131685,
1.58319531856068));
#53167=CARTESIAN_POINT('Ctrl Pts',(-0.554065814855426,0.566721053417116,
1.57924913197718));
#53168=CARTESIAN_POINT('Ctrl Pts',(-0.460420660203306,0.658275052702546,
1.57530294539369));
#53169=CARTESIAN_POINT('Ctrl Pts',(-0.343598118556019,0.726122277772382,
1.5713567588102));
#53170=CARTESIAN_POINT('Ctrl Pts',(-0.217670116177076,0.762090152213681,
1.56741057222671));
#53171=CARTESIAN_POINT('Ctrl Pts',(-0.091742113798131,0.79805802665498,
1.56346438564321));
#53172=CARTESIAN_POINT('Ctrl Pts',(0.04329134931247,0.80214655046774,1.55951819905972));
#53173=CARTESIAN_POINT('Ctrl Pts',(0.171164739900571,0.773863238170921,
1.55557201247623));
#53174=CARTESIAN_POINT('Ctrl Pts',(0.299038130488669,0.745579925874101,
1.55162582589274));
#53175=CARTESIAN_POINT('Ctrl Pts',(0.419751448554267,0.684924777467703,
1.54767963930925));
#53176=CARTESIAN_POINT('Ctrl Pts',(0.51876410212864,0.5992040436448,1.54373345272576));
#53177=CARTESIAN_POINT('Ctrl Pts',(0.617776755703014,0.513483309821894,
1.53978726614226));
#53178=CARTESIAN_POINT('Ctrl Pts',(0.695088744786162,0.402696990582482,
1.53584107955877));
#53179=CARTESIAN_POINT('Ctrl Pts',(0.741387409386929,0.280189915557558,
1.53189489297528));
#53180=CARTESIAN_POINT('Ctrl Pts',(0.787686073987695,0.157682840532634,
1.52794870639179));
#53181=CARTESIAN_POINT('Ctrl Pts',(0.802971414106082,0.0234550097221994,
1.5240025198083));
#53182=CARTESIAN_POINT('Ctrl Pts',(0.78540222533046,-0.106325086520418,
1.52005633322481));
#53183=CARTESIAN_POINT('Ctrl Pts',(0.767833036554838,-0.236105182763034,
1.51611014664131));
#53184=CARTESIAN_POINT('Ctrl Pts',(0.717409318885208,-0.361437544437834,
1.51216396005782));
#53185=CARTESIAN_POINT('Ctrl Pts',(0.640204890156501,-0.467225190028658,
1.50821777347433));
#53186=CARTESIAN_POINT('Ctrl Pts',(0.563000461427793,-0.573012835619484,
1.50427158689084));
#53187=CARTESIAN_POINT('Ctrl Pts',(0.459015321640008,-0.659255765126335,
1.50032540030735));
#53188=CARTESIAN_POINT('Ctrl Pts',(0.340775060452138,-0.715565537006538,
1.49637921372386));
#53189=CARTESIAN_POINT('Ctrl Pts',(0.222534799264268,-0.77187530888674,
1.49243302714036));
#53190=CARTESIAN_POINT('Ctrl Pts',(0.0900394166763145,-0.798251923140294,
1.48848684055687));
#53191=CARTESIAN_POINT('Ctrl Pts',(-0.040751280002766,-0.791518169567666,
1.48454065397338));
#53192=CARTESIAN_POINT('Ctrl Pts',(-0.171541976681846,-0.784784415995039,
1.48059446738989));
#53193=CARTESIAN_POINT('Ctrl Pts',(-0.300627987452053,-0.74494029459623,
1.4766482808064));
#53194=CARTESIAN_POINT('Ctrl Pts',(-0.412460182842351,-0.676785251868913,
1.4727020942229));
#53195=CARTESIAN_POINT('Ctrl Pts',(-0.524292378232649,-0.608630209141596,
1.46875590763941));
#53196=CARTESIAN_POINT('Ctrl Pts',(-0.618870758243037,-0.512164245085771,
1.46480972105592));
#53197=CARTESIAN_POINT('Ctrl Pts',(-0.684802829859224,-0.399007222734641,
1.46086353447243));
#53198=CARTESIAN_POINT('Ctrl Pts',(-0.750734901475411,-0.285850200383513,
1.45691734788894));
#53199=CARTESIAN_POINT('Ctrl Pts',(-0.788020664697396,-0.15600211973708,
1.45297116130545));
#53200=CARTESIAN_POINT('Ctrl Pts',(-0.792168841529171,-0.0251039058304422,
1.44902497472195));
#53201=CARTESIAN_POINT('Ctrl Pts',(-0.792433842828974,-0.0167416304902463,
1.44877287732681));
#53202=CARTESIAN_POINT('Ctrl Pts',(-0.792563605001957,-0.00837506940927601,
1.44852077993166));
#53203=CARTESIAN_POINT('Ctrl Pts',(-0.79255903846122,-8.36642852242164E-6,
1.44826868253652));
#53204=CARTESIAN_POINT('Ctrl Pts',(-0.792559834217432,-7.91270320494323E-6,
1.42673131746348));
#53205=CARTESIAN_POINT('Ctrl Pts',(-0.792563935225162,-0.00788846194650599,
1.42696876723405));
#53206=CARTESIAN_POINT('Ctrl Pts',(-0.792448816490436,-0.0157688911413652,
1.42720621700462));
#53207=CARTESIAN_POINT('Ctrl Pts',(-0.792213710879083,-0.023645739006679,
1.42744366677519));
#53208=CARTESIAN_POINT('Ctrl Pts',(-0.788306481964977,-0.154551367137981,
1.43138985335869));
#53209=CARTESIAN_POINT('Ctrl Pts',(-0.751259789709837,-0.28446785926946,
1.43533603994218));
#53210=CARTESIAN_POINT('Ctrl Pts',(-0.685536114679231,-0.397746049821345,
1.43928222652567));
#53211=CARTESIAN_POINT('Ctrl Pts',(-0.619812439648625,-0.511024240373231,
1.44322841310916));
#53212=CARTESIAN_POINT('Ctrl Pts',(-0.525411781842551,-0.607664129345523,
1.44717459969265));
#53213=CARTESIAN_POINT('Ctrl Pts',(-0.413705226645241,-0.676024903479442,
1.45112078627615));
#53214=CARTESIAN_POINT('Ctrl Pts',(-0.301998671447931,-0.74438567761336,
1.45506697285964));
#53215=CARTESIAN_POINT('Ctrl Pts',(-0.172986218859384,-0.784467336908906,
1.45901315944313));
#53216=CARTESIAN_POINT('Ctrl Pts',(-0.0422081378576713,-0.791441822104801,
1.46295934602662));
#53217=CARTESIAN_POINT('Ctrl Pts',(0.0885699431440433,-0.798416307300696,
1.46690553261011));
#53218=CARTESIAN_POINT('Ctrl Pts',(0.221113652558924,-0.772283618396939,
1.4708517191936));
#53219=CARTESIAN_POINT('Ctrl Pts',(0.339457361842355,-0.716191583425139,
1.4747979057771));
#53220=CARTESIAN_POINT('Ctrl Pts',(0.457801071125785,-0.660099548453339,
1.47874409236059));
#53221=CARTESIAN_POINT('Ctrl Pts',(0.561944780277766,-0.574048167413494,
1.48269027894408));
#53222=CARTESIAN_POINT('Ctrl Pts',(0.639343799075583,-0.468402808767816,
1.48663646552757));
#53223=CARTESIAN_POINT('Ctrl Pts',(0.7167428178734,-0.362757450122139,1.49058265211106));
#53224=CARTESIAN_POINT('Ctrl Pts',(0.767397146317053,-0.237518113870631,
1.49452883869456));
#53225=CARTESIAN_POINT('Ctrl Pts',(0.78520518821855,-0.107770576098722,
1.49847502527805));
#53226=CARTESIAN_POINT('Ctrl Pts',(0.803013230120048,0.021976961673187,
1.50242121186154));
#53227=CARTESIAN_POINT('Ctrl Pts',(0.787974985479389,0.156232700965494,
1.50636739844503));
#53228=CARTESIAN_POINT('Ctrl Pts',(0.7419018946807,0.278824789692679,1.51031358502852));
#53229=CARTESIAN_POINT('Ctrl Pts',(0.69582880388201,0.401416878419864,1.51425977161201));
#53230=CARTESIAN_POINT('Ctrl Pts',(0.618720866925289,0.512345316581927,
1.5182059581955));
#53231=CARTESIAN_POINT('Ctrl Pts',(0.519866164585757,0.598248155531527,
1.522152144779));
#53232=CARTESIAN_POINT('Ctrl Pts',(0.421011462246225,0.684150994481125,
1.52609833136249));
#53233=CARTESIAN_POINT('Ctrl Pts',(0.30040999452388,0.745028234218261,1.53004451794598));
#53234=CARTESIAN_POINT('Ctrl Pts',(0.172588880390198,0.773546871911222,
1.53399070452947));
#53235=CARTESIAN_POINT('Ctrl Pts',(0.0447677662565173,0.802065509604184,
1.53793689111296));
#53236=CARTESIAN_POINT('Ctrl Pts',(-0.0902729942885018,0.798225545252973,
1.54188307769645));
#53237=CARTESIAN_POINT('Ctrl Pts',(-0.216266988974055,0.762489523966117,
1.54582926427995));
#53238=CARTESIAN_POINT('Ctrl Pts',(-0.342260983659614,0.72675350267926,
1.54977545086344));
#53239=CARTESIAN_POINT('Ctrl Pts',(-0.459208212485706,0.659121424456755,
1.55372163744693));
#53240=CARTESIAN_POINT('Ctrl Pts',(-0.553021729923176,0.567739950074642,
1.55766782403042));
#53241=CARTESIAN_POINT('Ctrl Pts',(-0.646835247360645,0.47635847569253,
1.56161401061392));
#53242=CARTESIAN_POINT('Ctrl Pts',(-0.717515053409493,0.361227605150811,
1.56556019719741));
#53243=CARTESIAN_POINT('Ctrl Pts',(-0.756547371490182,0.236215493499633,
1.5695063837809));
#53244=CARTESIAN_POINT('Ctrl Pts',(-0.78036833582658,0.159922073080573,
1.57191469500842));
#53245=CARTESIAN_POINT('Ctrl Pts',(-0.792402138697298,0.0799483673713918,
1.57432300623595));
#53246=CARTESIAN_POINT('Ctrl Pts',(-0.792446584180059,-1.22568943931671E-5,
1.57673131746348));
#53247=CARTESIAN_POINT('Origin',(0.,0.,1.095));
#53248=CARTESIAN_POINT('',(-0.792481714638565,1.94816894887317E-5,1.74826868253652));
#53249=CARTESIAN_POINT('',(-0.792480310976121,1.93743401778285E-5,1.72673131746348));
#53250=CARTESIAN_POINT('',(-0.7925,-9.70532588324277E-17,1.095));
#53251=CARTESIAN_POINT('Ctrl Pts',(-0.792481714638565,1.94816894887317E-5,
1.74826868253652));
#53252=CARTESIAN_POINT('Ctrl Pts',(-0.792515970057648,0.0363124968327356,
1.74717544451896));
#53253=CARTESIAN_POINT('Ctrl Pts',(-0.790067815952362,0.0726009269833459,
1.7460822065014));
#53254=CARTESIAN_POINT('Ctrl Pts',(-0.785099074206255,0.108540882887942,
1.74498896848384));
#53255=CARTESIAN_POINT('Ctrl Pts',(-0.767163746582846,0.23827088634904,
1.74104278190035));
#53256=CARTESIAN_POINT('Ctrl Pts',(-0.716386571322305,0.36346046522512,
1.73709659531685));
#53257=CARTESIAN_POINT('Ctrl Pts',(-0.638883942196417,0.469029836983938,
1.73315040873336));
#53258=CARTESIAN_POINT('Ctrl Pts',(-0.561381313070528,0.574599208742756,
1.72920422214987));
#53259=CARTESIAN_POINT('Ctrl Pts',(-0.457153230079291,0.660548373384312,
1.72525803556638));
#53260=CARTESIAN_POINT('Ctrl Pts',(-0.338754546744625,0.716524274981285,
1.72131184898289));
#53261=CARTESIAN_POINT('Ctrl Pts',(-0.220355863409961,0.772500176578257,
1.7173656623994));
#53262=CARTESIAN_POINT('Ctrl Pts',(-0.0877865797318678,0.798502815130648,
1.7134194758159));
#53263=CARTESIAN_POINT('Ctrl Pts',(0.0429845951824947,0.791400027896518,
1.70947328923241));
#53264=CARTESIAN_POINT('Ctrl Pts',(0.173755770096857,0.784297240662389,
1.70552710264892));
#53265=CARTESIAN_POINT('Ctrl Pts',(0.302728836247484,0.744089027641742,
1.70158091606543));
#53266=CARTESIAN_POINT('Ctrl Pts',(0.414368268972285,0.6756186921974,1.69763472948194));
#53267=CARTESIAN_POINT('Ctrl Pts',(0.526007701697086,0.607148356753058,
1.69368854289845));
#53268=CARTESIAN_POINT('Ctrl Pts',(0.620313500996059,0.510415898885018,
1.68974235631495));
#53269=CARTESIAN_POINT('Ctrl Pts',(0.685926007720852,0.3970732822915,1.68579616973146));
#53270=CARTESIAN_POINT('Ctrl Pts',(0.751538514445645,0.283730665697983,
1.68184998314797));
#53271=CARTESIAN_POINT('Ctrl Pts',(0.788457728596263,0.153777890378985,
1.67790379656448));
#53272=CARTESIAN_POINT('Ctrl Pts',(0.792236525055337,0.0228684924264428,
1.67395760998099));
#53273=CARTESIAN_POINT('Ctrl Pts',(0.796015321514411,-0.108040905526099,
1.67001142339749));
#53274=CARTESIAN_POINT('Ctrl Pts',(0.766653700281941,-0.239906926112185,
1.666065236814));
#53275=CARTESIAN_POINT('Ctrl Pts',(0.707688432285305,-0.356845572183794,
1.66211905023051));
#53276=CARTESIAN_POINT('Ctrl Pts',(0.648723164288668,-0.473784218255407,
1.65817286364702));
#53277=CARTESIAN_POINT('Ctrl Pts',(0.560154249527864,-0.575795489812542,
1.65422667706353));
#53278=CARTESIAN_POINT('Ctrl Pts',(0.452650307433518,-0.650591560626139,
1.65028049048003));
#53279=CARTESIAN_POINT('Ctrl Pts',(0.345146365339177,-0.725387631439732,
1.64633430389654));
#53280=CARTESIAN_POINT('Ctrl Pts',(0.218707395911295,-0.772968501509789,
1.64238811731305));
#53281=CARTESIAN_POINT('Ctrl Pts',(0.088563677737676,-0.787602789839644,
1.63844193072956));
#53282=CARTESIAN_POINT('Ctrl Pts',(-0.0415800404359447,-0.802237078169498,
1.63449574414607));
#53283=CARTESIAN_POINT('Ctrl Pts',(-0.175428507355303,-0.78392478475915,
1.63054955756258));
#53284=CARTESIAN_POINT('Ctrl Pts',(-0.296858929162171,-0.734871727415269,
1.62660337097908));
#53285=CARTESIAN_POINT('Ctrl Pts',(-0.418289350969042,-0.685818670071388,
1.62265718439559));
#53286=CARTESIAN_POINT('Ctrl Pts',(-0.527301727663422,-0.606024848793974,
1.6187109978121));
#53287=CARTESIAN_POINT('Ctrl Pts',(-0.610764910881114,-0.505101874094718,
1.61476481122861));
#53288=CARTESIAN_POINT('Ctrl Pts',(-0.694228094098805,-0.404178899395464,
1.61081862464512));
#53289=CARTESIAN_POINT('Ctrl Pts',(-0.752142083839809,-0.28212677127437,
1.60687243806163));
#53290=CARTESIAN_POINT('Ctrl Pts',(-0.777530817250417,-0.153647348833338,
1.60292625147813));
#53291=CARTESIAN_POINT('Ctrl Pts',(-0.787519344460865,-0.103100510348724,
1.6013737284976));
#53292=CARTESIAN_POINT('Ctrl Pts',(-0.792473542933907,-0.0515588415030537,
1.59982120551706));
#53293=CARTESIAN_POINT('Ctrl Pts',(-0.792445760035067,-1.19013985881156E-5,
1.59826868253652));
#53294=CARTESIAN_POINT('Ctrl Pts',(-0.792446584180059,-1.22568943931671E-5,
1.57673131746348));
#53295=CARTESIAN_POINT('Ctrl Pts',(-0.792474965733008,-0.0510727145712751,
1.57826919281944));
#53296=CARTESIAN_POINT('Ctrl Pts',(-0.787614426950324,-0.102127838006081,
1.57980706817541));
#53297=CARTESIAN_POINT('Ctrl Pts',(-0.777812317880636,-0.152215908600686,
1.58134494353137));
#53298=CARTESIAN_POINT('Ctrl Pts',(-0.752660116077868,-0.280741846289199,
1.58529113011487));
#53299=CARTESIAN_POINT('Ctrl Pts',(-0.6949708823598,-0.402900368905588,
1.58923731669836));
#53300=CARTESIAN_POINT('Ctrl Pts',(-0.611693606464474,-0.503976801537991,
1.59318350328185));
#53301=CARTESIAN_POINT('Ctrl Pts',(-0.52841633056915,-0.605053234170393,
1.59712968986534));
#53302=CARTESIAN_POINT('Ctrl Pts',(-0.41955101249657,-0.685047576818808,
1.60107587644883));
#53303=CARTESIAN_POINT('Ctrl Pts',(-0.298211086580291,-0.734324065054783,
1.60502206303232));
#53304=CARTESIAN_POINT('Ctrl Pts',(-0.176871160664012,-0.783600553290759,
1.60896824961582));
#53305=CARTESIAN_POINT('Ctrl Pts',(-0.0430566269040337,-0.802159187114293,
1.61291443619931));
#53306=CARTESIAN_POINT('Ctrl Pts',(0.0871138082795939,-0.787764475642946,
1.6168606227828));
#53307=CARTESIAN_POINT('Ctrl Pts',(0.217284243463222,-0.773369764171598,
1.62080680936629));
#53308=CARTESIAN_POINT('Ctrl Pts',(0.343810580070499,-0.726021707405367,
1.62475299594978));
#53309=CARTESIAN_POINT('Ctrl Pts',(0.451452015649914,-0.651423642680866,
1.62869918253328));
#53310=CARTESIAN_POINT('Ctrl Pts',(0.559093451229331,-0.576825577956364,
1.63264536911677));
#53311=CARTESIAN_POINT('Ctrl Pts',(0.647849985780886,-0.474977505273591,
1.63659155570026));
#53312=CARTESIAN_POINT('Ctrl Pts',(0.70703040002444,-0.358147592647585,
1.64053774228375));
#53313=CARTESIAN_POINT('Ctrl Pts',(0.766210814267993,-0.241317680021578,
1.64448392886724));
#53314=CARTESIAN_POINT('Ctrl Pts',(0.795815108203546,-0.10950592745234,
1.64843011545073));
#53315=CARTESIAN_POINT('Ctrl Pts',(0.792277279624073,0.021410204797208,
1.65237630203423));
#53316=CARTESIAN_POINT('Ctrl Pts',(0.7887394510446,0.152326337046754,1.65632248861772));
#53317=CARTESIAN_POINT('Ctrl Pts',(0.752059499950102,0.282346848976609,
1.66026867520121));
#53318=CARTESIAN_POINT('Ctrl Pts',(0.686655730889281,0.395810045242522,
1.6642148617847));
#53319=CARTESIAN_POINT('Ctrl Pts',(0.621251961828459,0.509273241508435,
1.66816104836819));
#53320=CARTESIAN_POINT('Ctrl Pts',(0.527124374801314,0.606179122110405,
1.67210723495168));
#53321=CARTESIAN_POINT('Ctrl Pts',(0.415611162294765,0.674854833615329,
1.67605342153518));
#53322=CARTESIAN_POINT('Ctrl Pts',(0.304097949788216,0.743530545120253,
1.67999960811867));
#53323=CARTESIAN_POINT('Ctrl Pts',(0.175199111802263,0.783976087528131,
1.68394579470216));
#53324=CARTESIAN_POINT('Ctrl Pts',(0.0444412318028534,0.791319569828665,
1.68789198128565));
#53325=CARTESIAN_POINT('Ctrl Pts',(-0.0863166481965564,0.7986630521292,
1.69183816786914));
#53326=CARTESIAN_POINT('Ctrl Pts',(-0.218933570209423,0.772904474322392,
1.69578435445264));
#53327=CARTESIAN_POINT('Ctrl Pts',(-0.337435086825647,0.717146600673075,
1.69973054103613));
#53328=CARTESIAN_POINT('Ctrl Pts',(-0.455936603441873,0.661388727023757,
1.70367672761962));
#53329=CARTESIAN_POINT('Ctrl Pts',(-0.560322714661454,0.575631557531931,
1.70762291420311));
#53330=CARTESIAN_POINT('Ctrl Pts',(-0.638019531581584,0.470205021239029,
1.7115691007866));
#53331=CARTESIAN_POINT('Ctrl Pts',(-0.715716348501714,0.364778484946126,
1.71551528737009));
#53332=CARTESIAN_POINT('Ctrl Pts',(-0.766723871122392,0.239682581852148,
1.71946147395359));
#53333=CARTESIAN_POINT('Ctrl Pts',(-0.784897959048439,0.109985810719267,
1.72340766053708));
#53334=CARTESIAN_POINT('Ctrl Pts',(-0.790000305490033,0.0735736473485991,
1.72451554617921));
#53335=CARTESIAN_POINT('Ctrl Pts',(-0.792514731297942,0.0367988450569207,
1.72562343182135));
#53336=CARTESIAN_POINT('Ctrl Pts',(-0.792480310976121,1.93743401778285E-5,
1.72673131746348));
#53337=CARTESIAN_POINT('Origin',(0.,0.,1.095));
#53338=CARTESIAN_POINT('',(-0.792561345414955,-6.95798684707816E-6,1.89826868253652));
#53339=CARTESIAN_POINT('',(-0.792562019808975,-6.48812038781812E-6,1.87673131746348));
#53340=CARTESIAN_POINT('',(-0.7925,-9.70532588324277E-17,1.095));
#53341=CARTESIAN_POINT('Ctrl Pts',(-0.792561345414955,-6.95798684707816E-6,
1.89826868253652));
#53342=CARTESIAN_POINT('Ctrl Pts',(-0.792503577448366,0.124083294659953,
1.89452968352086));
#53343=CARTESIAN_POINT('Ctrl Pts',(-0.762860507627894,0.248200183905096,
1.8907906845052));
#53344=CARTESIAN_POINT('Ctrl Pts',(-0.706678680884356,0.358841081198739,
1.88705168548954));
#53345=CARTESIAN_POINT('Ctrl Pts',(-0.647383674385861,0.475612875643471,
1.88310549890605));
#53346=CARTESIAN_POINT('Ctrl Pts',(-0.558527260508677,0.577373820519587,
1.87915931232256));
#53347=CARTESIAN_POINT('Ctrl Pts',(-0.450812689552982,0.651866242813804,
1.87521312573907));
#53348=CARTESIAN_POINT('Ctrl Pts',(-0.343098118597287,0.726358665108021,
1.87126693915557));
#53349=CARTESIAN_POINT('Ctrl Pts',(-0.21652539056308,0.773582564820339,
1.86732075257208));
#53350=CARTESIAN_POINT('Ctrl Pts',(-0.0863408960085328,0.78784956003754,
1.86337456598859));
#53351=CARTESIAN_POINT('Ctrl Pts',(0.0438435985460143,0.80211655525474,
1.8594283794051));
#53352=CARTESIAN_POINT('Ctrl Pts',(0.177639859620902,0.783426645976824,
1.85548219282161));
#53353=CARTESIAN_POINT('Ctrl Pts',(0.298931381843208,0.734031135939183,
1.85153600623812));
#53354=CARTESIAN_POINT('Ctrl Pts',(0.420222904065518,0.684635625901541,
1.84758981965462));
#53355=CARTESIAN_POINT('Ctrl Pts',(0.529009687435246,0.604534515104173,
1.84364363307113));
#53356=CARTESIAN_POINT('Ctrl Pts',(0.612187757561329,0.503376428797804,
1.83969744648764));
#53357=CARTESIAN_POINT('Ctrl Pts',(0.695365827687409,0.402218342491439,
1.83575125990415));
#53358=CARTESIAN_POINT('Ctrl Pts',(0.752935184569847,0.280003280676073,
1.83180507332066));
#53359=CARTESIAN_POINT('Ctrl Pts',(0.777961278303689,0.151452728723369,
1.82785888673717));
#53360=CARTESIAN_POINT('Ctrl Pts',(0.802987372037531,0.0229021767706633,
1.82391270015367));
#53361=CARTESIAN_POINT('Ctrl Pts',(0.795470202622776,-0.111983865319381,
1.81996651357018));
#53362=CARTESIAN_POINT('Ctrl Pts',(0.75631525501308,-0.236957621975268,
1.81602032698669));
#53363=CARTESIAN_POINT('Ctrl Pts',(0.717160307403383,-0.361931378631156,
1.8120741404032));
#53364=CARTESIAN_POINT('Ctrl Pts',(0.646367581598744,-0.476992849852886,
1.80812795381971));
#53365=CARTESIAN_POINT('Ctrl Pts',(0.552464455992677,-0.568282240125679,
1.80418176723621));
#53366=CARTESIAN_POINT('Ctrl Pts',(0.458561330386612,-0.659571630398471,
1.80023558065272));
#53367=CARTESIAN_POINT('Ctrl Pts',(0.341547804979119,-0.727088939722326,
1.79628939406923));
#53368=CARTESIAN_POINT('Ctrl Pts',(0.215518811092083,-0.762701331874485,
1.79234320748574));
#53369=CARTESIAN_POINT('Ctrl Pts',(0.0894898172050466,-0.798313724026643,
1.78839702090225));
#53370=CARTESIAN_POINT('Ctrl Pts',(-0.0455546451615332,-0.802021199007106,
1.78445083431876));
#53371=CARTESIAN_POINT('Ctrl Pts',(-0.173347717831807,-0.773377170790614,
1.78050464773526));
#53372=CARTESIAN_POINT('Ctrl Pts',(-0.301140790502082,-0.744733142574123,
1.77655846115177));
#53373=CARTESIAN_POINT('Ctrl Pts',(-0.42168247347605,-0.683737611160677,
1.77261227456828));
#53374=CARTESIAN_POINT('Ctrl Pts',(-0.5204528491884,-0.597737828273649,
1.76866608798479));
#53375=CARTESIAN_POINT('Ctrl Pts',(-0.61922322490075,-0.51173804538662,
1.7647199014013));
#53376=CARTESIAN_POINT('Ctrl Pts',(-0.696222293351481,-0.400734011026008,
1.7607737148178));
#53377=CARTESIAN_POINT('Ctrl Pts',(-0.742175087583709,-0.278096779822644,
1.75682752823431));
#53378=CARTESIAN_POINT('Ctrl Pts',(-0.775397277065014,-0.189434547186454,
1.75397457966838));
#53379=CARTESIAN_POINT('Ctrl Pts',(-0.792392320611665,-0.0946919204416087,
1.75112163110245));
#53380=CARTESIAN_POINT('Ctrl Pts',(-0.792481714638565,1.94816894887317E-5,
1.74826868253652));
#53381=CARTESIAN_POINT('Ctrl Pts',(-0.792480310976121,1.93743401778285E-5,
1.72673131746348));
#53382=CARTESIAN_POINT('Ctrl Pts',(-0.792392129282894,-0.0942062410012334,
1.72956961840484));
#53383=CARTESIAN_POINT('Ctrl Pts',(-0.775574922487285,-0.188462496952598,
1.73240791934619));
#53384=CARTESIAN_POINT('Ctrl Pts',(-0.742685718766298,-0.276730207636548,
1.73524622028755));
#53385=CARTESIAN_POINT('Ctrl Pts',(-0.696958737326693,-0.399451815687699,
1.73919240687104));
#53386=CARTESIAN_POINT('Ctrl Pts',(-0.620164121216066,-0.510597392618217,
1.74313859345454));
#53387=CARTESIAN_POINT('Ctrl Pts',(-0.5215522099674,-0.596778834205856,
1.74708478003803));
#53388=CARTESIAN_POINT('Ctrl Pts',(-0.422940298718735,-0.682960275793493,
1.75103096662152));
#53389=CARTESIAN_POINT('Ctrl Pts',(-0.302511092332032,-0.744177582038251,
1.75497715320501));
#53390=CARTESIAN_POINT('Ctrl Pts',(-0.174770959940769,-0.773056787202183,
1.7589233397885));
#53391=CARTESIAN_POINT('Ctrl Pts',(-0.0470308275495023,-0.801935992366116,
1.762869526372));
#53392=CARTESIAN_POINT('Ctrl Pts',(0.088020230846324,-0.79847709644922,
1.76681571295549));
#53393=CARTESIAN_POINT('Ctrl Pts',(0.21411456254238,-0.763096742743189,
1.77076189953898));
#53394=CARTESIAN_POINT('Ctrl Pts',(0.340208894238434,-0.727716389037158,
1.77470808612247));
#53395=CARTESIAN_POINT('Ctrl Pts',(0.457346499234716,-0.660414577541993,
1.77865427270596));
#53396=CARTESIAN_POINT('Ctrl Pts',(0.551417500131295,-0.569298186565646,
1.78260045928945));
#53397=CARTESIAN_POINT('Ctrl Pts',(0.645488501027873,-0.478181795589299,
1.78654664587295));
#53398=CARTESIAN_POINT('Ctrl Pts',(0.716492897824747,-0.363250825131771,
1.79049283245644));
#53399=CARTESIAN_POINT('Ctrl Pts',(0.755877815177639,-0.238349351163912,
1.79443901903993));
#53400=CARTESIAN_POINT('Ctrl Pts',(0.795262732530532,-0.113447877196051,
1.79838520562342));
#53401=CARTESIAN_POINT('Ctrl Pts',(0.803028170439441,0.021424100282145,
1.80233139220691));
#53402=CARTESIAN_POINT('Ctrl Pts',(0.778238738626799,0.150020499861006,
1.80627757879041));
#53403=CARTESIAN_POINT('Ctrl Pts',(0.753449306814156,0.278616899439865,
1.8102237653739));
#53404=CARTESIAN_POINT('Ctrl Pts',(0.696105005279964,0.400937721119394,
1.81416995195739));
#53405=CARTESIAN_POINT('Ctrl Pts',(0.613113274758198,0.502248740160955,
1.81811613854088));
#53406=CARTESIAN_POINT('Ctrl Pts',(0.53012154423643,0.603559759202518,1.82206232512437));
#53407=CARTESIAN_POINT('Ctrl Pts',(0.421482384727094,0.683860975606109,
1.82600851170787));
#53408=CARTESIAN_POINT('Ctrl Pts',(0.300281988504285,0.733479660289139,
1.82995469829136));
#53409=CARTESIAN_POINT('Ctrl Pts',(0.179081592281479,0.783098344972167,
1.83390088487485));
#53410=CARTESIAN_POINT('Ctrl Pts',(0.0453199593452004,0.802034497934631,
1.83784707145834));
#53411=CARTESIAN_POINT('Ctrl Pts',(-0.0848905760835689,0.788007154009545,
1.84179325804183));
#53412=CARTESIAN_POINT('Ctrl Pts',(-0.21510111151234,0.773979810084459,
1.84573944462532));
#53413=CARTESIAN_POINT('Ctrl Pts',(-0.341760549433607,0.726988969271823,
1.84968563120882));
#53414=CARTESIAN_POINT('Ctrl Pts',(-0.449612054600708,0.652694940255893,
1.85363181779231));
#53415=CARTESIAN_POINT('Ctrl Pts',(-0.557463559767808,0.578400911239963,
1.8575780043758));
#53416=CARTESIAN_POINT('Ctrl Pts',(-0.646507132180743,0.476803694020739,
1.86152419095929));
#53417=CARTESIAN_POINT('Ctrl Pts',(-0.706016977249189,0.360141239674046,
1.86547037754278));
#53418=CARTESIAN_POINT('Ctrl Pts',(-0.762623254037114,0.249170909068881,
1.86922402418301));
#53419=CARTESIAN_POINT('Ctrl Pts',(-0.79250747892361,0.124569584863353,
1.87297767082325));
#53420=CARTESIAN_POINT('Ctrl Pts',(-0.792562019808975,-6.48812038781812E-6,
1.87673131746348));
#53421=CARTESIAN_POINT('Origin',(0.,0.,1.095));
#53422=CARTESIAN_POINT('',(-0.792448351156449,-1.30718296499355E-5,2.04826868253652));
#53423=CARTESIAN_POINT('',(-0.792449256123249,-1.33074723724148E-5,2.02673131746348));
#53424=CARTESIAN_POINT('',(-0.7925,-9.70532588324277E-17,1.095));
#53425=CARTESIAN_POINT('Ctrl Pts',(-0.792448351156449,-1.30718296499355E-5,
2.04826868253652));
#53426=CARTESIAN_POINT('Ctrl Pts',(-0.792400580040907,0.0809518333973197,
2.04583010910626));
#53427=CARTESIAN_POINT('Ctrl Pts',(-0.780057502508409,0.161931022031344,
2.04339153567599));
#53428=CARTESIAN_POINT('Ctrl Pts',(-0.755643607895046,0.239090868906411,
2.04095296224572));
#53429=CARTESIAN_POINT('Ctrl Pts',(-0.716136172040015,0.363953687775635,
2.03700677566223));
#53430=CARTESIAN_POINT('Ctrl Pts',(-0.645019047037377,0.478814846861572,
2.03306058907874));
#53431=CARTESIAN_POINT('Ctrl Pts',(-0.550858697000239,0.569838878089452,
2.02911440249525));
#53432=CARTESIAN_POINT('Ctrl Pts',(-0.456698346963102,0.660862909317332,
2.02516821591175));
#53433=CARTESIAN_POINT('Ctrl Pts',(-0.339494771891465,0.728049812687156,
2.02122202932826));
#53434=CARTESIAN_POINT('Ctrl Pts',(-0.213365790576425,0.7633064507015,2.01727584274477));
#53435=CARTESIAN_POINT('Ctrl Pts',(-0.087236809261385,0.798563088715845,
2.01332965616128));
#53436=CARTESIAN_POINT('Ctrl Pts',(0.0478175782970594,0.801889461374709,
2.00938346957779));
#53437=CARTESIAN_POINT('Ctrl Pts',(0.175529315812979,0.772884939389923,
2.0054372829943));
#53438=CARTESIAN_POINT('Ctrl Pts',(0.303241053328903,0.743880417405136,
2.0014910964108));
#53439=CARTESIAN_POINT('Ctrl Pts',(0.423610140802298,0.682545000776699,
1.99754490982731));
#53440=CARTESIAN_POINT('Ctrl Pts',(0.522137452055428,0.596266856583147,
1.99359872324382));
#53441=CARTESIAN_POINT('Ctrl Pts',(0.620664763308554,0.509988712389599,
1.98965253666033));
#53442=CARTESIAN_POINT('Ctrl Pts',(0.697350298341415,0.398767840630934,
1.98570635007684));
#53443=CARTESIAN_POINT('Ctrl Pts',(0.742956856388529,0.276001428216633,
1.98176016349334));
#53444=CARTESIAN_POINT('Ctrl Pts',(0.788563414435643,0.153235015802332,
1.97781397690985));
#53445=CARTESIAN_POINT('Ctrl Pts',(0.803090995497015,0.0189230627323887,
1.97386779032636));
#53446=CARTESIAN_POINT('Ctrl Pts',(0.784789671794817,-0.110755814222861,
1.96992160374287));
#53447=CARTESIAN_POINT('Ctrl Pts',(0.76648834809262,-0.240434691178112,
1.96597541715938));
#53448=CARTESIAN_POINT('Ctrl Pts',(0.715358119626854,-0.365480492018664,
1.96202923057589));
#53449=CARTESIAN_POINT('Ctrl Pts',(0.63755790722776,-0.470830749750958,
1.95808304399239));
#53450=CARTESIAN_POINT('Ctrl Pts',(0.559757694828668,-0.576181007483251,
1.9541368574089));
#53451=CARTESIAN_POINT('Ctrl Pts',(0.455287498496249,-0.66183572210728,
1.95019067082541));
#53452=CARTESIAN_POINT('Ctrl Pts',(0.336731335738727,-0.717477307524271,
1.94624448424192));
#53453=CARTESIAN_POINT('Ctrl Pts',(0.218175172981203,-0.773118892941263,
1.94229829765843));
#53454=CARTESIAN_POINT('Ctrl Pts',(0.0855330437985741,-0.798747349151216,
1.93835211107493));
#53455=CARTESIAN_POINT('Ctrl Pts',(-0.0452175680979145,-0.791275584909749,
1.93440592449144));
#53456=CARTESIAN_POINT('Ctrl Pts',(-0.175968179994401,-0.783803820668283,
1.93045973790795));
#53457=CARTESIAN_POINT('Ctrl Pts',(-0.304827274604749,-0.743231835975397,
1.92651355132446));
#53458=CARTESIAN_POINT('Ctrl Pts',(-0.416273055752392,-0.674446752949849,
1.92256736474097));
#53459=CARTESIAN_POINT('Ctrl Pts',(-0.527718836900035,-0.605661669924301,
1.91862117815748));
#53460=CARTESIAN_POINT('Ctrl Pts',(-0.621751304584975,-0.508663488566089,
1.91467499157398));
#53461=CARTESIAN_POINT('Ctrl Pts',(-0.687043723986203,-0.39513618023112,
1.91072880499049));
#53462=CARTESIAN_POINT('Ctrl Pts',(-0.752336143387432,-0.281608871896149,
1.906782618407));
#53463=CARTESIAN_POINT('Ctrl Pts',(-0.78888851450495,-0.151552436584419,
1.90283643182351));
#53464=CARTESIAN_POINT('Ctrl Pts',(-0.792297900503804,-0.0206328969218787,
1.89889024524002));
#53465=CARTESIAN_POINT('Ctrl Pts',(-0.792476904303538,-0.013759197356366,
1.89868305767219));
#53466=CARTESIAN_POINT('Ctrl Pts',(-0.792564546486805,-0.00688311856615801,
1.89847587010435));
#53467=CARTESIAN_POINT('Ctrl Pts',(-0.792561345414955,-6.95798684707816E-6,
1.89826868253652));
#53468=CARTESIAN_POINT('Ctrl Pts',(-0.792562019808975,-6.48812038781812E-6,
1.87673131746348));
#53469=CARTESIAN_POINT('Ctrl Pts',(-0.792564817434852,-0.0063965062341521,
1.87692385740674));
#53470=CARTESIAN_POINT('Ctrl Pts',(-0.792489130621737,-0.0127864579098014,
1.87711639735));
#53471=CARTESIAN_POINT('Ctrl Pts',(-0.79233453996622,-0.0191745001120404,
1.87730893729326));
#53472=CARTESIAN_POINT('Ctrl Pts',(-0.789166139890846,-0.150100094077262,
1.88125512387675));
#53473=CARTESIAN_POINT('Ctrl Pts',(-0.752853222016141,-0.280223590533543,
1.88520131046024));
#53474=CARTESIAN_POINT('Ctrl Pts',(-0.687769879693997,-0.393870889078232,
1.88914749704373));
#53475=CARTESIAN_POINT('Ctrl Pts',(-0.622686537371856,-0.507518187622918,
1.89309368362722));
#53476=CARTESIAN_POINT('Ctrl Pts',(-0.528832770602275,-0.604689288256013,
1.89703987021072));
#53477=CARTESIAN_POINT('Ctrl Pts',(-0.417513788695573,-0.673679390309865,
1.90098605679421));
#53478=CARTESIAN_POINT('Ctrl Pts',(-0.306194806788868,-0.742669492363719,
1.9049322433777));
#53479=CARTESIAN_POINT('Ctrl Pts',(-0.177410609745039,-0.783478595838328,
1.90887842996119));
#53480=CARTESIAN_POINT('Ctrl Pts',(-0.0466739718904146,-0.791191016773624,
1.91282461654468));
#53481=CARTESIAN_POINT('Ctrl Pts',(0.0840626659642058,-0.798903437708921,
1.91677080312818));
#53482=CARTESIAN_POINT('Ctrl Pts',(0.216751744629622,-0.773519176104906,
1.92071698971167));
#53483=CARTESIAN_POINT('Ctrl Pts',(0.335410125026388,-0.718095907739533,
1.92466317629516));
#53484=CARTESIAN_POINT('Ctrl Pts',(0.454068505423155,-0.66267263937416,
1.92860936287865));
#53485=CARTESIAN_POINT('Ctrl Pts',(0.558696187551273,-0.577210364247426,
1.93255554946214));
#53486=CARTESIAN_POINT('Ctrl Pts',(0.636690183942362,-0.472003489758499,
1.93650173604564));
#53487=CARTESIAN_POINT('Ctrl Pts',(0.714684180333452,-0.36679661526957,
1.94044792262913));
#53488=CARTESIAN_POINT('Ctrl Pts',(0.766044490987512,-0.241845141418452,
1.94439410921262));
#53489=CARTESIAN_POINT('Ctrl Pts',(0.78458448023081,-0.112200169605353,
1.94834029579611));
#53490=CARTESIAN_POINT('Ctrl Pts',(0.803124469474107,0.0174448022077428,
1.9522864823796));
#53491=CARTESIAN_POINT('Ctrl Pts',(0.788844137306641,0.151783271982819,
1.95623266896309));
#53492=CARTESIAN_POINT('Ctrl Pts',(0.743463629318252,0.274633422178461,
1.96017885554659));
#53493=CARTESIAN_POINT('Ctrl Pts',(0.698083121329863,0.397483572374106,
1.96412504213008));
#53494=CARTESIAN_POINT('Ctrl Pts',(0.621602437520548,0.508845402990322,
1.96807122871357));
#53495=CARTESIAN_POINT('Ctrl Pts',(0.523234102552766,0.595304761057008,
1.97201741529706));
#53496=CARTESIAN_POINT('Ctrl Pts',(0.424865767584983,0.681764119123695,
1.97596360188055));
#53497=CARTESIAN_POINT('Ctrl Pts',(0.304609781458736,0.74332100464085,1.97990978846404));
#53498=CARTESIAN_POINT('Ctrl Pts',(0.176951647912409,0.772560547231348,
1.98385597504754));
#53499=CARTESIAN_POINT('Ctrl Pts',(0.0492935143660849,0.801800089821845,
1.98780216163103));
#53500=CARTESIAN_POINT('Ctrl Pts',(-0.0857667666003156,0.798722289485685,
1.99174834821452));
#53501=CARTESIAN_POINT('Ctrl Pts',(-0.211960431274993,0.763697885264852,
1.99569453479801));
#53502=CARTESIAN_POINT('Ctrl Pts',(-0.338154095949671,0.728673481044019,
1.9996407213815));
#53503=CARTESIAN_POINT('Ctrl Pts',(-0.455481144332627,0.661702472938513,
2.00358690796499));
#53504=CARTESIAN_POINT('Ctrl Pts',(-0.549808879704876,0.570851890488339,
2.00753309454849));
#53505=CARTESIAN_POINT('Ctrl Pts',(-0.644136615077125,0.480001308038165,
2.01147928113198));
#53506=CARTESIAN_POINT('Ctrl Pts',(-0.715465037438667,0.365271151243323,
2.01542546771547));
#53507=CARTESIAN_POINT('Ctrl Pts',(-0.75520224037866,0.240481310225466,
2.01937165429896));
#53508=CARTESIAN_POINT('Ctrl Pts',(-0.779905619413149,0.162903360238067,
2.0218248753538));
#53509=CARTESIAN_POINT('Ctrl Pts',(-0.792399873864259,0.0814376230681167,
2.02427809640864));
#53510=CARTESIAN_POINT('Ctrl Pts',(-0.792449256123249,-1.33074723724148E-5,
2.02673131746348));
#53511=CARTESIAN_POINT('Origin',(0.,0.,0.522718733092613));
#53512=CARTESIAN_POINT('',(-0.706803933141875,-1.1659082385242E-5,2.09771873309261));
#53513=CARTESIAN_POINT('',(-0.706829164831431,1.42933870884709E-5,2.12728126690739));
#53514=CARTESIAN_POINT('',(-0.70685,-2.56204009907072E-14,0.522718733092613));
#53515=CARTESIAN_POINT('',(0.347825520797267,-0.615372974259066,2.1475));
#53516=CARTESIAN_POINT('Ctrl Pts',(-0.706803933141875,-1.16590823852313E-5,
2.09771873309261));
#53517=CARTESIAN_POINT('Ctrl Pts',(-0.706830275063582,-0.0446572816595,
2.09922634624584));
#53518=CARTESIAN_POINT('Ctrl Pts',(-0.691762579617961,-0.206145477660671,
2.10468014598255));
#53519=CARTESIAN_POINT('Ctrl Pts',(-0.570183826489577,-0.466147172833569,
2.11408013230277));
#53520=CARTESIAN_POINT('Ctrl Pts',(-0.279700959344392,-0.681302019989293,
2.12591869205323));
#53521=CARTESIAN_POINT('Ctrl Pts',(0.0570467425526827,-0.729307650008237,
2.13705864795232));
#53522=CARTESIAN_POINT('Ctrl Pts',(0.264076432689668,-0.662598430928655,
2.1442524172679));
#53523=CARTESIAN_POINT('Ctrl Pts',(0.347825520797267,-0.615372974259065,
2.1475));
#53524=CARTESIAN_POINT('',(-0.468142317532551,-0.529603335559031,2.1475));
#53525=CARTESIAN_POINT('Origin',(0.,0.,2.1475));
#53526=CARTESIAN_POINT('Ctrl Pts',(-0.706829164831431,1.42933870884675E-5,
2.12728126690739));
#53527=CARTESIAN_POINT('Ctrl Pts',(-0.706754789907476,-0.0827061914899486,
2.13007465802143));
#53528=CARTESIAN_POINT('Ctrl Pts',(-0.671726507282576,-0.282346804235477,
2.13681423571897));
#53529=CARTESIAN_POINT('Ctrl Pts',(-0.555684412749315,-0.452220591560317,
2.14355381341651));
#53530=CARTESIAN_POINT('Ctrl Pts',(-0.468142317532544,-0.529603335559038,
2.1475));
#53531=CARTESIAN_POINT('Origin',(0.,0.,0.522718733092613));
#53532=CARTESIAN_POINT('',(-0.706904715465692,-6.20599748763955E-6,1.94771873309261));
#53533=CARTESIAN_POINT('',(-0.706804740303746,-1.18692578732482E-5,1.97728126690739));
#53534=CARTESIAN_POINT('',(-0.70685,-2.56204009907072E-14,0.522718733092613));
#53535=CARTESIAN_POINT('Ctrl Pts',(-0.706904715465692,-6.20599748754613E-6,
1.94771873309261));
#53536=CARTESIAN_POINT('Ctrl Pts',(-0.70690757057943,-0.00613922064163216,
1.94792592066044));
#53537=CARTESIAN_POINT('Ctrl Pts',(-0.705340536134816,-0.129082898063355,
1.95207929481177));
#53538=CARTESIAN_POINT('Ctrl Pts',(-0.638424933033424,-0.367174286939925,
1.96017885554658));
#53539=CARTESIAN_POINT('Ctrl Pts',(-0.386815407040617,-0.626719389121822,
1.97201741529706));
#53540=CARTESIAN_POINT('Ctrl Pts',(-0.0420177375441198,-0.735280805071978,
1.98385597504754));
#53541=CARTESIAN_POINT('Ctrl Pts',(0.312902473229659,-0.666704877228424,
1.99569453479801));
#53542=CARTESIAN_POINT('Ctrl Pts',(0.592440990368726,-0.437512315593109,
2.00753309454849));
#53543=CARTESIAN_POINT('Ctrl Pts',(0.729253868568196,-0.102918154113688,
2.01937165429896));
#53544=CARTESIAN_POINT('Ctrl Pts',(0.690381361287827,0.256470126116556,
2.03121021404944));
#53545=CARTESIAN_POINT('Ctrl Pts',(0.485188287074669,0.554071917419808,
2.04304877379991));
#53546=CARTESIAN_POINT('Ctrl Pts',(0.163107948346954,0.718191561244962,
2.05488733355038));
#53547=CARTESIAN_POINT('Ctrl Pts',(-0.198266917945865,0.709290943526656,
2.06672589330087));
#53548=CARTESIAN_POINT('Ctrl Pts',(-0.511877064467201,0.529514050225861,
2.07856445305133));
#53549=CARTESIAN_POINT('Ctrl Pts',(-0.677936930706799,0.261311015960508,
2.08889539964859));
#53550=CARTESIAN_POINT('Ctrl Pts',(-0.706761324923553,0.0722029065449757,
2.09528015966235));
#53551=CARTESIAN_POINT('Ctrl Pts',(-0.706803933141875,-1.16590823852313E-5,
2.09771873309261));
#53552=CARTESIAN_POINT('Ctrl Pts',(-0.706804740303746,-1.18692578732899E-5,
1.97728126690739));
#53553=CARTESIAN_POINT('Ctrl Pts',(-0.706831545071039,-0.0442235615473762,
1.97877423243604));
#53554=CARTESIAN_POINT('Ctrl Pts',(-0.691952157749641,-0.205277190188198,
1.98421338454819));
#53555=CARTESIAN_POINT('Ctrl Pts',(-0.571040857364167,-0.465097524278119,
1.99359872324382));
#53556=CARTESIAN_POINT('Ctrl Pts',(-0.280954601492375,-0.680784722238707,
2.0054372829943));
#53557=CARTESIAN_POINT('Ctrl Pts',(0.0768167392428667,-0.732463381911148,
2.01727584274477));
#53558=CARTESIAN_POINT('Ctrl Pts',(0.416082091960603,-0.607683269644344,
2.02911440249525));
#53559=CARTESIAN_POINT('Ctrl Pts',(0.655108589511754,-0.336505836512168,
2.04095296224572));
#53560=CARTESIAN_POINT('Ctrl Pts',(0.736312206455239,0.0157403015675272,
2.0527915219962));
#53561=CARTESIAN_POINT('Ctrl Pts',(0.640129844349537,0.364193045069704,
2.06463008174667));
#53562=CARTESIAN_POINT('Ctrl Pts',(0.389733384979782,0.624910355165805,
2.07646864149715));
#53563=CARTESIAN_POINT('Ctrl Pts',(0.0454451798068112,0.735074392267673,
2.08830720124762));
#53564=CARTESIAN_POINT('Ctrl Pts',(-0.309790030899746,0.668161503213349,
2.1001457609981));
#53565=CARTESIAN_POINT('Ctrl Pts',(-0.590395841023348,0.440259893769033,
2.11198432074857));
#53566=CARTESIAN_POINT('Ctrl Pts',(-0.696114850406353,0.185128362892587,
2.12102948938501));
#53567=CARTESIAN_POINT('Ctrl Pts',(-0.706859858376257,0.0341519405347402,
2.12612847143794));
#53568=CARTESIAN_POINT('Ctrl Pts',(-0.706829164831431,1.42933870884675E-5,
2.12728126690739));
#53569=CARTESIAN_POINT('Origin',(0.,0.,0.522718733092613));
#53570=CARTESIAN_POINT('',(-0.70683369084198,1.7376192061708E-5,1.79771873309261));
#53571=CARTESIAN_POINT('',(-0.7069053169741,-5.78691218949823E-6,1.82728126690739));
#53572=CARTESIAN_POINT('',(-0.70685,-2.56204009907072E-14,0.522718733092613));
#53573=CARTESIAN_POINT('Ctrl Pts',(-0.70683369084198,1.73761920617202E-5,
1.79771873309261));
#53574=CARTESIAN_POINT('Ctrl Pts',(-0.706753958137987,-0.0844580239295342,
1.80057168165854));
#53575=CARTESIAN_POINT('Ctrl Pts',(-0.670628779363002,-0.285845817928073,
1.80737081680797));
#53576=CARTESIAN_POINT('Ctrl Pts',(-0.483622895882263,-0.55543878746919,
1.81811613854088));
#53577=CARTESIAN_POINT('Ctrl Pts',(-0.161080730796523,-0.718648975656924,
1.82995469829136));
#53578=CARTESIAN_POINT('Ctrl Pts',(0.200267577937169,-0.708728614685542,
1.84179325804183));
#53579=CARTESIAN_POINT('Ctrl Pts',(0.513369194723111,-0.528067630096644,
1.85363181779231));
#53580=CARTESIAN_POINT('Ctrl Pts',(0.702794449871408,-0.22018926694303,
1.86547037754278));
#53581=CARTESIAN_POINT('Ctrl Pts',(0.722908687855579,0.140735145112547,
1.87730893729326));
#53582=CARTESIAN_POINT('Ctrl Pts',(0.568866164528063,0.467754891904443,
1.88914749704373));
#53583=CARTESIAN_POINT('Ctrl Pts',(0.277777440900717,0.68208727108596,1.90098605679421));
#53584=CARTESIAN_POINT('Ctrl Pts',(-0.0802309646795408,0.732097223286951,
1.91282461654468));
#53585=CARTESIAN_POINT('Ctrl Pts',(-0.418910836519209,0.605736793589845,
1.92466317629516));
#53586=CARTESIAN_POINT('Ctrl Pts',(-0.652509368967175,0.338212972333276,
1.9362945484778));
#53587=CARTESIAN_POINT('Ctrl Pts',(-0.706853190813096,0.110672904517833,
1.94397973407695));
#53588=CARTESIAN_POINT('Ctrl Pts',(-0.706904715465692,-6.20599748754613E-6,
1.94771873309261));
#53589=CARTESIAN_POINT('Ctrl Pts',(-0.7069053169741,-5.78691218945833E-6,
1.82728126690739));
#53590=CARTESIAN_POINT('Ctrl Pts',(-0.706907812244574,-0.00570519928280016,
1.82747380685065));
#53591=CARTESIAN_POINT('Ctrl Pts',(-0.705456723071662,-0.128215175728052,
1.8316125333774));
#53592=CARTESIAN_POINT('Ctrl Pts',(-0.639099702185964,-0.365998534307576,
1.83969744648764));
#53593=CARTESIAN_POINT('Ctrl Pts',(-0.387968339254434,-0.626006329194029,
1.85153600623812));
#53594=CARTESIAN_POINT('Ctrl Pts',(-0.043371078634514,-0.735202221147443,
1.86337456598859));
#53595=CARTESIAN_POINT('Ctrl Pts',(0.311674758291609,-0.667279702605622,
1.87521312573907));
#53596=CARTESIAN_POINT('Ctrl Pts',(0.591634671650319,-0.438602065356417,
1.88705168548954));
#53597=CARTESIAN_POINT('Ctrl Pts',(0.729063197527252,-0.104260301476294,
1.89889024524002));
#53598=CARTESIAN_POINT('Ctrl Pts',(0.690852272129496,0.255198931434154,
1.91072880499049));
#53599=CARTESIAN_POINT('Ctrl Pts',(0.486207333262819,0.553177896624332,
1.92256736474097));
#53600=CARTESIAN_POINT('Ctrl Pts',(0.16442962805144,0.71789014089361,1.93440592449145));
#53601=CARTESIAN_POINT('Ctrl Pts',(-0.196961007662504,0.709654646252797,
1.94624448424192));
#53602=CARTESIAN_POINT('Ctrl Pts',(-0.51090154072052,0.530455439643165,
1.9580830439924));
#53603=CARTESIAN_POINT('Ctrl Pts',(-0.677690936174323,0.262178463108642,
1.96842863821422));
#53604=CARTESIAN_POINT('Ctrl Pts',(-0.706760695067449,0.0726361941522846,
1.97482804585255));
#53605=CARTESIAN_POINT('Ctrl Pts',(-0.706804740303746,-1.18692578732899E-5,
1.97728126690739));
#53606=CARTESIAN_POINT('Origin',(0.,0.,0.522718733092613));
#53607=CARTESIAN_POINT('',(-0.706801622057775,-1.06151464860647E-5,1.64771873309261));
#53608=CARTESIAN_POINT('',(-0.706832438881351,1.728044458367E-5,1.67728126690739));
#53609=CARTESIAN_POINT('',(-0.70685,-2.56204009907072E-14,0.522718733092613));
#53610=CARTESIAN_POINT('Ctrl Pts',(-0.706801622057775,-1.06151464860232E-5,
1.64771873309261));
#53611=CARTESIAN_POINT('Ctrl Pts',(-0.706826402300104,-0.0459865831122182,
1.64927125607315));
#53612=CARTESIAN_POINT('Ctrl Pts',(-0.691176049341311,-0.208807130958488,
1.65476996563718));
#53613=CARTESIAN_POINT('Ctrl Pts',(-0.567544005886828,-0.469358235709884,
1.6642148617847));
#53614=CARTESIAN_POINT('Ctrl Pts',(-0.275851645761568,-0.682868377930474,
1.67605342153517));
#53615=CARTESIAN_POINT('Ctrl Pts',(0.0822964508010132,-0.731867915837495,
1.68789198128565));
#53616=CARTESIAN_POINT('Ctrl Pts',(0.420618414990665,-0.604552314541516,
1.69973054103613));
#53617=CARTESIAN_POINT('Ctrl Pts',(0.657608714291634,-0.331593321607157,
1.7115691007866));
#53618=CARTESIAN_POINT('Ctrl Pts',(0.736173743824141,0.0212501988393111,
1.72340766053708));
#53619=CARTESIAN_POINT('Ctrl Pts',(0.637386312193742,0.36897430950518,1.73524622028755));
#53620=CARTESIAN_POINT('Ctrl Pts',(0.38504541288342,0.627808395980971,1.74708478003803));
#53621=CARTESIAN_POINT('Ctrl Pts',(0.0399427814314016,0.735396441559441,
1.7589233397885));
#53622=CARTESIAN_POINT('Ctrl Pts',(-0.314782511317597,0.665819286755307,
1.77076189953898));
#53623=CARTESIAN_POINT('Ctrl Pts',(-0.5936731881467,0.435838843751334,1.78260045928945));
#53624=CARTESIAN_POINT('Ctrl Pts',(-0.696798799331513,0.181585790695073,
1.791586070474));
#53625=CARTESIAN_POINT('Ctrl Pts',(-0.706864244082333,0.0323879979636773,
1.79662549507505));
#53626=CARTESIAN_POINT('Ctrl Pts',(-0.70683369084198,1.73761920617202E-5,
1.79771873309261));
#53627=CARTESIAN_POINT('Ctrl Pts',(-0.706832438881352,1.72804445836769E-5,
1.67728126690739));
#53628=CARTESIAN_POINT('Ctrl Pts',(-0.706753787487206,-0.0840248346394162,
1.68011956784875));
#53629=CARTESIAN_POINT('Ctrl Pts',(-0.670899552291929,-0.284978893811032,
1.6869040553736));
#53630=CARTESIAN_POINT('Ctrl Pts',(-0.484644460168804,-0.554547656814542,
1.69763472948194));
#53631=CARTESIAN_POINT('Ctrl Pts',(-0.162403256883848,-0.718351264079303,
1.70947328923241));
#53632=CARTESIAN_POINT('Ctrl Pts',(0.198962701325951,-0.709096044222425,
1.72131184898289));
#53633=CARTESIAN_POINT('Ctrl Pts',(0.512396326909379,-0.529011682877222,
1.73315040873336));
#53634=CARTESIAN_POINT('Ctrl Pts',(0.702387965556207,-0.221482510128057,
1.74498896848384));
#53635=CARTESIAN_POINT('Ctrl Pts',(0.723166513641681,0.139404268220684,
1.75682752823431));
#53636=CARTESIAN_POINT('Ctrl Pts',(0.569726187309398,0.46670700438791,1.76866608798479));
#53637=CARTESIAN_POINT('Ctrl Pts',(0.279032471602733,0.681574820721842,
1.78050464773527));
#53638=CARTESIAN_POINT('Ctrl Pts',(-0.0788832769436621,0.732243665093515,
1.79234320748574));
#53639=CARTESIAN_POINT('Ctrl Pts',(-0.417795164746744,0.606506848077444,
1.80418176723622));
#53640=CARTESIAN_POINT('Ctrl Pts',(-0.652180521522544,0.339077101493092,
1.81582778704343));
#53641=CARTESIAN_POINT('Ctrl Pts',(-0.706856670633635,0.111106638562335,
1.82352762026716));
#53642=CARTESIAN_POINT('Ctrl Pts',(-0.7069053169741,-5.78691218945833E-6,
1.82728126690739));
#53643=CARTESIAN_POINT('Origin',(0.,0.,0.522718733092613));
#53644=CARTESIAN_POINT('',(-0.706902657837619,-7.46222082938423E-6,1.49771873309261));
#53645=CARTESIAN_POINT('',(-0.706802357132712,-1.09322218498076E-5,1.52728126690739));
#53646=CARTESIAN_POINT('',(-0.70685,-2.56204009907072E-14,0.522718733092613));
#53647=CARTESIAN_POINT('Ctrl Pts',(-0.706902657837619,-7.46222082939445E-6,
1.49771873309261));
#53648=CARTESIAN_POINT('Ctrl Pts',(-0.706906730846225,-0.00746992783842311,
1.49797083048776));
#53649=CARTESIAN_POINT('Ctrl Pts',(-0.704979296674476,-0.13174339950389,
1.50216911446639));
#53650=CARTESIAN_POINT('Ctrl Pts',(-0.636342616245341,-0.370771394253652,
1.51031358502852));
#53651=CARTESIAN_POINT('Ctrl Pts',(-0.383272352862338,-0.628892403816528,
1.522152144779));
#53652=CARTESIAN_POINT('Ctrl Pts',(-0.0378675072613757,-0.735506222910841,
1.53399070452947));
#53653=CARTESIAN_POINT('Ctrl Pts',(0.316660042955515,-0.664928394071252,
1.54582926427995));
#53654=CARTESIAN_POINT('Ctrl Pts',(0.594900658951714,-0.434161903010362,
1.55766782403042));
#53655=CARTESIAN_POINT('Ctrl Pts',(0.729823074730051,-0.0988009698248782,
1.5695063837809));
#53656=CARTESIAN_POINT('Ctrl Pts',(0.688922976322423,0.260362218345552,
1.58134494353137));
#53657=CARTESIAN_POINT('Ctrl Pts',(0.482053653356788,0.556801245806918,
1.59318350328185));
#53658=CARTESIAN_POINT('Ctrl Pts',(0.159052231749204,0.719100646378767,
1.60502206303232));
#53659=CARTESIAN_POINT('Ctrl Pts',(-0.202266645473739,0.708160685279523,
1.6168606227828));
#53660=CARTESIAN_POINT('Ctrl Pts',(-0.514857233095386,0.526616921087925,
1.62869918253327));
#53661=CARTESIAN_POINT('Ctrl Pts',(-0.678685547138705,0.25865074554612,
1.63898521930321));
#53662=CARTESIAN_POINT('Ctrl Pts',(-0.706763416140776,0.070874648717395,
1.64532506948966));
#53663=CARTESIAN_POINT('Ctrl Pts',(-0.706801622057775,-1.06151464860232E-5,
1.64771873309261));
#53664=CARTESIAN_POINT('Ctrl Pts',(-0.706802357132712,-1.09322218498076E-5,
1.52728126690739));
#53665=CARTESIAN_POINT('Ctrl Pts',(-0.70682767132918,-0.0455529946936496,
1.52881914226335));
#53666=CARTESIAN_POINT('Ctrl Pts',(-0.691368236317636,-0.2079389765849,
1.53430320420281));
#53667=CARTESIAN_POINT('Ctrl Pts',(-0.568406982135528,-0.468312779144872,
1.54373345272576));
#53668=CARTESIAN_POINT('Ctrl Pts',(-0.277108117480876,-0.682359471009978,
1.55557201247623));
#53669=CARTESIAN_POINT('Ctrl Pts',(0.0809491816544183,-0.732018159911551,
1.56741057222671));
#53670=CARTESIAN_POINT('Ctrl Pts',(0.419504920572478,-0.605325514137882,
1.57924913197718));
#53671=CARTESIAN_POINT('Ctrl Pts',(0.656997247819542,-0.33280320432406,
1.59108769172766));
#53672=CARTESIAN_POINT('Ctrl Pts',(0.736211614387408,0.0198951072351811,
1.60292625147813));
#53673=CARTESIAN_POINT('Ctrl Pts',(0.638064396351524,0.367800465686733,
1.61476481122861));
#53674=CARTESIAN_POINT('Ctrl Pts',(0.386200352603368,0.62709859200914,1.62660337097908));
#53675=CARTESIAN_POINT('Ctrl Pts',(0.0412963388606396,0.735321677123366,
1.63844193072956));
#53676=CARTESIAN_POINT('Ctrl Pts',(-0.313556423252151,0.666397573441058,
1.65028049048004));
#53677=CARTESIAN_POINT('Ctrl Pts',(-0.59286994772746,0.436930865850026,
1.66211905023051));
#53678=CARTESIAN_POINT('Ctrl Pts',(-0.696632251283717,0.18245391022506,
1.67111930903963));
#53679=CARTESIAN_POINT('Ctrl Pts',(-0.706863139202462,0.0328217837583204,
1.67617338126525));
#53680=CARTESIAN_POINT('Ctrl Pts',(-0.706832438881352,1.72804445836769E-5,
1.67728126690739));
#53681=CARTESIAN_POINT('Origin',(0.,0.,0.522718733092613));
#53682=CARTESIAN_POINT('',(-0.706837600175146,1.76134468301129E-5,1.34771873309261));
#53683=CARTESIAN_POINT('',(-0.706903367591914,-7.0575322025368E-6,1.37728126690739));
#53684=CARTESIAN_POINT('',(-0.70685,-2.56204009907072E-14,0.522718733092613));
#53685=CARTESIAN_POINT('Ctrl Pts',(-0.706837600175146,1.76134468300899E-5,
1.34771873309261));
#53686=CARTESIAN_POINT('Ctrl Pts',(-0.706754721657063,-0.0857861962986243,
1.35061659148585));
#53687=CARTESIAN_POINT('Ctrl Pts',(-0.669792860630747,-0.288503634206156,
1.35746063646259));
#53688=CARTESIAN_POINT('Ctrl Pts',(-0.480480572542965,-0.558159270688526,
1.36825086802282));
#53689=CARTESIAN_POINT('Ctrl Pts',(-0.157022466269567,-0.719546591356936,
1.38008942777329));
#53690=CARTESIAN_POINT('Ctrl Pts',(0.204264102488947,-0.707587117237976,
1.39192798752377));
#53691=CARTESIAN_POINT('Ctrl Pts',(0.516341171985148,-0.525162018961544,
1.40376654727424));
#53692=CARTESIAN_POINT('Ctrl Pts',(0.704025897392014,-0.216219536231424,
1.41560510702472));
#53693=CARTESIAN_POINT('Ctrl Pts',(0.722102936199932,0.144812643019176,
1.42744366677519));
#53694=CARTESIAN_POINT('Ctrl Pts',(0.566217328251717,0.470957842311017,
1.43928222652567));
#53695=CARTESIAN_POINT('Ctrl Pts',(0.273923654190083,0.683644047529059,
1.45112078627614));
#53696=CARTESIAN_POINT('Ctrl Pts',(-0.0843612816475947,0.73163278098069,
1.46295934602662));
#53697=CARTESIAN_POINT('Ctrl Pts',(-0.422322644344321,0.603363021837419,
1.4747979057771));
#53698=CARTESIAN_POINT('Ctrl Pts',(-0.653511582405244,0.335563154723619,
1.48638436813243));
#53699=CARTESIAN_POINT('Ctrl Pts',(-0.706842974329004,0.109343185930717,
1.49402464390426));
#53700=CARTESIAN_POINT('Ctrl Pts',(-0.706902657837619,-7.46222082939445E-6,
1.49771873309261));
#53701=CARTESIAN_POINT('Ctrl Pts',(-0.706903367591914,-7.05753220258103E-6,
1.37728126690739));
#53702=CARTESIAN_POINT('Ctrl Pts',(-0.706907025380322,-0.00703591082257907,
1.37751871667796));
#53703=CARTESIAN_POINT('Ctrl Pts',(-0.705097952042887,-0.130875652267875,
1.38170235303202));
#53704=CARTESIAN_POINT('Ctrl Pts',(-0.637024010013693,-0.3695994685019,
1.38983217596958));
#53705=CARTESIAN_POINT('Ctrl Pts',(-0.384429290883511,-0.62818586163779,
1.40167073572005));
#53706=CARTESIAN_POINT('Ctrl Pts',(-0.0392212702694481,-0.735435278191946,
1.41350929547053));
#53707=CARTESIAN_POINT('Ctrl Pts',(0.315435591559856,-0.665510138185811,
1.425347855221));
#53708=CARTESIAN_POINT('Ctrl Pts',(0.594100503158886,-0.435256187316358,
1.43718641497148));
#53709=CARTESIAN_POINT('Ctrl Pts',(0.729639980990038,-0.100144169034792,
1.44902497472195));
#53710=CARTESIAN_POINT('Ctrl Pts',(0.689401053958178,0.259093695894295,
1.46086353447243));
#53711=CARTESIAN_POINT('Ctrl Pts',(0.483077728136633,0.555913001313301,
1.47270209422291));
#53712=CARTESIAN_POINT('Ctrl Pts',(0.160375592643109,0.718806667842741,
1.48454065397338));
#53713=CARTESIAN_POINT('Ctrl Pts',(-0.200962810856885,0.708531795407456,
1.49637921372385));
#53714=CARTESIAN_POINT('Ctrl Pts',(-0.51388703304889,0.527563715313158,
1.50821777347433));
#53715=CARTESIAN_POINT('Ctrl Pts',(-0.678442306952803,0.259518385311895,
1.51851845786884));
#53716=CARTESIAN_POINT('Ctrl Pts',(-0.706762715127049,0.0713078908220291,
1.52487295567986));
#53717=CARTESIAN_POINT('Ctrl Pts',(-0.706802357132712,-1.09322218498076E-5,
1.52728126690739));
#53718=CARTESIAN_POINT('Origin',(0.,0.,0.522718733092613));
#53719=CARTESIAN_POINT('',(-0.70679951935905,-9.6117180550407E-6,1.19771873309261));
#53720=CARTESIAN_POINT('',(-0.70683631828199,1.75454709868683E-5,1.22728126690739));
#53721=CARTESIAN_POINT('',(-0.70685,-2.56204009907072E-14,0.522718733092613));
#53722=CARTESIAN_POINT('Ctrl Pts',(-0.70679951935905,-9.61171805506644E-6,
1.19771873309261));
#53723=CARTESIAN_POINT('Ctrl Pts',(-0.706822516721899,-0.0473159294520395,
1.19931616590046));
#53724=CARTESIAN_POINT('Ctrl Pts',(-0.690581482598579,-0.211468896388643,
1.2048597852918));
#53725=CARTESIAN_POINT('Ctrl Pts',(-0.564886142186152,-0.472553698972733,
1.21434959126664));
#53726=CARTESIAN_POINT('Ctrl Pts',(-0.271993481537794,-0.684414273702493,
1.22618815101711));
#53727=CARTESIAN_POINT('Ctrl Pts',(0.0864254407786529,-0.731391820594802,
1.23802671076759));
#53728=CARTESIAN_POINT('Ctrl Pts',(0.42402351100988,-0.602168924935201,
1.24986527051806));
#53729=CARTESIAN_POINT('Ctrl Pts',(0.65946959076411,-0.327876822761505,
1.26170383026854));
#53730=CARTESIAN_POINT('Ctrl Pts',(0.7360420948641,0.02540446092383,1.27354239001901));
#53731=CARTESIAN_POINT('Ctrl Pts',(0.635293853503172,0.372565526784018,
1.28538094976949));
#53732=CARTESIAN_POINT('Ctrl Pts',(0.381496241085932,0.62997140417964,1.29721950951997));
#53733=CARTESIAN_POINT('Ctrl Pts',(0.0357919315763396,0.735610147891393,
1.30905806927044));
#53734=CARTESIAN_POINT('Ctrl Pts',(-0.318535053229798,0.664032206982953,
1.32089662902092));
#53735=CARTESIAN_POINT('Ctrl Pts',(-0.596123392939055,0.432481505312761,
1.33273518877139));
#53736=CARTESIAN_POINT('Ctrl Pts',(-0.697304244243687,0.178924149227873,
1.34167589012862));
#53737=CARTESIAN_POINT('Ctrl Pts',(-0.706867582277473,0.0310579682124794,
1.34667040490236));
#53738=CARTESIAN_POINT('Ctrl Pts',(-0.706837600175146,1.76134468300899E-5,
1.34771873309261));
#53739=CARTESIAN_POINT('Ctrl Pts',(-0.70683631828199,1.75454709868614E-5,
1.22728126690739));
#53740=CARTESIAN_POINT('Ctrl Pts',(-0.706754436578726,-0.0853530034866889,
1.23016447767606));
#53741=CARTESIAN_POINT('Ctrl Pts',(-0.670066454565782,-0.287636803571761,
1.23699387502822));
#53742=CARTESIAN_POINT('Ctrl Pts',(-0.481507149662053,-0.557273919428443,
1.24776945896388));
#53743=CARTESIAN_POINT('Ctrl Pts',(-0.158346651432958,-0.719256348203324,
1.25960801871435));
#53744=CARTESIAN_POINT('Ctrl Pts',(0.202961320248067,-0.707961905001939,
1.27144657846483));
#53745=CARTESIAN_POINT('Ctrl Pts',(0.515373647430983,-0.526111547092912,
1.2832851382153));
#53746=CARTESIAN_POINT('Ctrl Pts',(0.703626717974851,-0.217515052818769,
1.29512369796578));
#53747=CARTESIAN_POINT('Ctrl Pts',(0.722368268691099,0.143483242363127,
1.30696225771625));
#53748=CARTESIAN_POINT('Ctrl Pts',(0.567083251096378,0.469914825023403,
1.31880081746673));
#53749=CARTESIAN_POINT('Ctrl Pts',(0.275181556922342,0.683138688101186,
1.3306393772172));
#53750=CARTESIAN_POINT('Ctrl Pts',(-0.0830144418180345,0.731786826132074,
1.34247793696768));
#53751=CARTESIAN_POINT('Ctrl Pts',(-0.421211336145891,0.604139360373918,
1.35431649671815));
#53752=CARTESIAN_POINT('Ctrl Pts',(-0.653185707793217,0.336427474765252,
1.36591760669806));
#53753=CARTESIAN_POINT('Ctrl Pts',(-0.70684623645849,0.109776863875274,
1.37357253009447));
#53754=CARTESIAN_POINT('Ctrl Pts',(-0.706903367591914,-7.05753220258103E-6,
1.37728126690739));
#53755=CARTESIAN_POINT('Origin',(0.,0.,0.522718733092613));
#53756=CARTESIAN_POINT('',(-0.706900287114882,-8.66958556023345E-6,1.04771873309261));
#53757=CARTESIAN_POINT('',(-0.706800184200881,-9.94400265103002E-6,1.07728126690739));
#53758=CARTESIAN_POINT('',(-0.70685,-2.56204009907072E-14,0.522718733092613));
#53759=CARTESIAN_POINT('Ctrl Pts',(-0.706900287114882,-8.66958556019516E-6,
1.04771873309261));
#53760=CARTESIAN_POINT('Ctrl Pts',(-0.706905729970906,-0.0088006199353823,
1.04801574031507));
#53761=CARTESIAN_POINT('Ctrl Pts',(-0.70461048072898,-0.134403976845368,
1.05225893412102));
#53762=CARTESIAN_POINT('Ctrl Pts',(-0.634240032318171,-0.374356692787108,
1.06044831451046));
#53763=CARTESIAN_POINT('Ctrl Pts',(-0.379717091696098,-0.631045388490867,
1.07228687426093));
#53764=CARTESIAN_POINT('Ctrl Pts',(-0.0337160709028718,-0.73570821566756,
1.08412543401141));
#53765=CARTESIAN_POINT('Ctrl Pts',(0.320407527210959,-0.663130732629247,
1.09596399376188));
#53766=CARTESIAN_POINT('Ctrl Pts',(0.597341380372839,-0.430797664036932,
1.10780255351236));
#53767=CARTESIAN_POINT('Ctrl Pts',(0.730369036319385,-0.094680635997126,
1.11964111326283));
#53768=CARTESIAN_POINT('Ctrl Pts',(0.687442649847106,0.264246012681654,
1.13147967301331));
#53769=CARTESIAN_POINT('Ctrl Pts',(0.478903665966244,0.559512851300696,
1.14331823276378));
#53770=CARTESIAN_POINT('Ctrl Pts',(0.154991450519341,0.719986807040808,
1.15515679251426));
#53771=CARTESIAN_POINT('Ctrl Pts',(-0.206259933078302,0.707007915127706,
1.16699535226474));
#53772=CARTESIAN_POINT('Ctrl Pts',(-0.51782099957674,0.523702935302196,
1.17883391201521));
#53773=CARTESIAN_POINT('Ctrl Pts',(-0.679425760049597,0.255990445315929,
1.18907503895784));
#53774=CARTESIAN_POINT('Ctrl Pts',(-0.706765705640842,0.0695462981414409,
1.19536997931697));
#53775=CARTESIAN_POINT('Ctrl Pts',(-0.70679951935905,-9.61171805506644E-6,
1.19771873309261));
#53776=CARTESIAN_POINT('Ctrl Pts',(-0.706800184200881,-9.94400265104389E-6,
1.07728126690739));
#53777=CARTESIAN_POINT('Ctrl Pts',(-0.706823787147948,-0.0468823619700862,
1.07886405209067));
#53778=CARTESIAN_POINT('Ctrl Pts',(-0.690776290670716,-0.21060074762263,
1.08439302385743));
#53779=CARTESIAN_POINT('Ctrl Pts',(-0.565755004731942,-0.471513129267208,
1.09386818220769));
#53780=CARTESIAN_POINT('Ctrl Pts',(-0.273252805267132,-0.683912465791199,
1.10570674195817));
#53781=CARTESIAN_POINT('Ctrl Pts',(0.0850790409901614,-0.7315496655969,
1.11754530170865));
#53782=CARTESIAN_POINT('Ctrl Pts',(0.422914397879838,-0.602948396230368,
1.12938386145912));
#53783=CARTESIAN_POINT('Ctrl Pts',(0.658864962009067,-0.329090137025705,
1.14122242120959));
#53784=CARTESIAN_POINT('Ctrl Pts',(0.736087612291053,0.0240496046218443,
1.15306098096007));
#53785=CARTESIAN_POINT('Ctrl Pts',(0.635978551456582,0.371395528430276,
1.16489954071055));
#53786=CARTESIAN_POINT('Ctrl Pts',(0.382655168196356,0.629268129419748,
1.17673810046102));
#53787=CARTESIAN_POINT('Ctrl Pts',(0.0371458893840861,0.735543023454563,
1.1885766602115));
#53788=CARTESIAN_POINT('Ctrl Pts',(-0.317312248253455,0.664617403894264,
1.20041521996197));
#53789=CARTESIAN_POINT('Ctrl Pts',(-0.595326328143767,0.433578043112969,
1.21225377971245));
#53790=CARTESIAN_POINT('Ctrl Pts',(-0.697140254592215,0.179792257193208,
1.22120912869425));
#53791=CARTESIAN_POINT('Ctrl Pts',(-0.706866506248542,0.0314917719916984,
1.22621829109257));
#53792=CARTESIAN_POINT('Ctrl Pts',(-0.70683631828199,1.75454709868614E-5,
1.22728126690739));
#53793=CARTESIAN_POINT('Origin',(0.,0.,0.522718733092613));
#53794=CARTESIAN_POINT('',(-0.706841592163942,1.78676093792155E-5,0.897718733092612));
#53795=CARTESIAN_POINT('',(-0.70690109581483,-8.28105672090462E-6,0.927281266907388));
#53796=CARTESIAN_POINT('',(-0.70685,-2.56204009907072E-14,0.522718733092613));
#53797=CARTESIAN_POINT('Ctrl Pts',(-0.706841592163942,1.7867609379222E-5,
0.897718733092612));
#53798=CARTESIAN_POINT('Ctrl Pts',(-0.706755847239672,-0.0871142953232393,
0.900661501313167));
#53799=CARTESIAN_POINT('Ctrl Pts',(-0.668948275249204,-0.291161300644555,
0.907550456117214));
#53800=CARTESIAN_POINT('Ctrl Pts',(-0.47732294727357,-0.560861892554869,
0.918385597504754));
#53801=CARTESIAN_POINT('Ctrl Pts',(-0.152959200118396,-0.720421332568536,
0.930224157255227));
#53802=CARTESIAN_POINT('Ctrl Pts',(0.20825412107116,-0.70642306199211,0.942062717005705));
#53803=CARTESIAN_POINT('Ctrl Pts',(0.519296704228398,-0.522239692636662,
0.953901276756179));
#53804=CARTESIAN_POINT('Ctrl Pts',(0.705234922034154,-0.212242913538608,
0.965739836506655));
#53805=CARTESIAN_POINT('Ctrl Pts',(0.721274186030318,0.148885525939063,
0.97757839625713));
#53806=CARTESIAN_POINT('Ctrl Pts',(0.563550458271255,0.474145794399759,
0.989416956007605));
#53807=CARTESIAN_POINT('Ctrl Pts',(0.270061143182683,0.68517904960402,1.00125551575808));
#53808=CARTESIAN_POINT('Ctrl Pts',(-0.0884889117632597,0.731145036959546,
1.01309407550856));
#53809=CARTESIAN_POINT('Ctrl Pts',(-0.425721001442049,0.600970033160064,
1.02493263525903));
#53810=CARTESIAN_POINT('Ctrl Pts',(-0.654504697899648,0.332912764005127,
1.03647418778705));
#53811=CARTESIAN_POINT('Ctrl Pts',(-0.706833413462098,0.108013632008419,
1.04406955373158));
#53812=CARTESIAN_POINT('Ctrl Pts',(-0.706900287114882,-8.66958556019516E-6,
1.04771873309261));
#53813=CARTESIAN_POINT('Ctrl Pts',(-0.70690109581483,-8.28105672094105E-6,
0.927281266907388));
#53814=CARTESIAN_POINT('Ctrl Pts',(-0.706906076802844,-0.00836660754601505,
0.927563626505272));
#53815=CARTESIAN_POINT('Ctrl Pts',(-0.704731608357342,-0.133536203475843,
0.931792172686647));
#53816=CARTESIAN_POINT('Ctrl Pts',(-0.63492802922278,-0.373188632550485,
0.939966905451515));
#53817=CARTESIAN_POINT('Ctrl Pts',(-0.380877998557793,-0.630345386040242,
0.951805465201989));
#53818=CARTESIAN_POINT('Ctrl Pts',(-0.0350702127852755,-0.735644912405828,
0.963644024952465));
#53819=CARTESIAN_POINT('Ctrl Pts',(0.319186378418513,-0.663719377496494,
0.97548258470294));
#53820=CARTESIAN_POINT('Ctrl Pts',(0.596547412907388,-0.43189644669194,
0.987321144453416));
#53821=CARTESIAN_POINT('Ctrl Pts',(0.730193525854251,-0.0960248470611938,
0.99915970420389));
#53822=CARTESIAN_POINT('Ctrl Pts',(0.68792787877927,0.262980208441528,1.01099826395437));
#53823=CARTESIAN_POINT('Ctrl Pts',(0.47993273725243,0.558630400335474,1.02283682370484));
#53824=CARTESIAN_POINT('Ctrl Pts',(0.156316449407645,0.71970030157465,1.03467538345532));
#53825=CARTESIAN_POINT('Ctrl Pts',(-0.204958213586156,0.707386377546527,
1.04651394320579));
#53826=CARTESIAN_POINT('Ctrl Pts',(-0.516856158218931,0.524655189777677,
1.05835250295627));
#53827=CARTESIAN_POINT('Ctrl Pts',(-0.679185260542492,0.256858137567063,
1.06860827752347));
#53828=CARTESIAN_POINT('Ctrl Pts',(-0.706764940480673,0.0699795526303456,
1.07491786550717));
#53829=CARTESIAN_POINT('Ctrl Pts',(-0.706800184200881,-9.94400265104389E-6,
1.07728126690739));
#53830=CARTESIAN_POINT('Origin',(1.87600653078293E-16,4.24518889064203E-17,
2.1475));
#53831=CARTESIAN_POINT('',(0.418139433688265,0.673212941048267,2.1475));
#53832=CARTESIAN_POINT('Ctrl Pts',(0.347825520797284,-0.615372974259056,
2.1475));
#53833=CARTESIAN_POINT('Ctrl Pts',(0.366504384047157,-0.606234343800672,
2.1475));
#53834=CARTESIAN_POINT('Ctrl Pts',(0.384749844785911,-0.596282384617426,
2.1475));
#53835=CARTESIAN_POINT('Ctrl Pts',(0.402505152806889,-0.585540595271413,
2.1475));
#53836=CARTESIAN_POINT('Ctrl Pts',(0.428009251227577,-0.570110862800913,
2.1475));
#53837=CARTESIAN_POINT('Ctrl Pts',(0.452502861659596,-0.553052634814332,
2.1475));
#53838=CARTESIAN_POINT('Ctrl Pts',(0.475875172607634,-0.534507449294233,
2.1475));
#53839=CARTESIAN_POINT('Ctrl Pts',(0.483690013455006,-0.528306621586319,
2.1475));
#53840=CARTESIAN_POINT('Ctrl Pts',(0.49137937742968,-0.52193932807035,2.1475));
#53841=CARTESIAN_POINT('Ctrl Pts',(0.498938722077998,-0.515410220415254,
2.1475));
#53842=CARTESIAN_POINT('Ctrl Pts',(0.506291908151787,-0.509059174694062,
2.1475));
#53843=CARTESIAN_POINT('Ctrl Pts',(0.513516097025268,-0.502560044328262,
2.1475));
#53844=CARTESIAN_POINT('Ctrl Pts',(0.520602202220868,-0.495922947505538,
2.1475));
#53845=CARTESIAN_POINT('Ctrl Pts',(0.546097282072312,-0.472043353736282,
2.1475));
#53846=CARTESIAN_POINT('Ctrl Pts',(0.569829953644379,-0.446361692321662,
2.1475));
#53847=CARTESIAN_POINT('Ctrl Pts',(0.591620827976965,-0.419094425996583,
2.1475));
#53848=CARTESIAN_POINT('Ctrl Pts',(0.602803004994532,-0.4051019907148,2.1475));
#53849=CARTESIAN_POINT('Ctrl Pts',(0.613473370194027,-0.390691282161003,
2.1475));
#53850=CARTESIAN_POINT('Ctrl Pts',(0.623603958795138,-0.375887559258075,
2.1475));
#53851=CARTESIAN_POINT('Ctrl Pts',(0.628606813990278,-0.368576939416676,
2.1475));
#53852=CARTESIAN_POINT('Ctrl Pts',(0.633473720251848,-0.361176490586554,
2.1475));
#53853=CARTESIAN_POINT('Ctrl Pts',(0.638197570377914,-0.353696641187965,
2.1475));
#53854=CARTESIAN_POINT('Ctrl Pts',(0.642548760340772,-0.34680687018375,
2.1475));
#53855=CARTESIAN_POINT('Ctrl Pts',(0.646779785634514,-0.339847969614829,
2.1475));
#53856=CARTESIAN_POINT('Ctrl Pts',(0.650888589541644,-0.332822744658013,
2.1475));
#53857=CARTESIAN_POINT('Ctrl Pts',(0.668513875925227,-0.30268706416031,
2.1475));
#53858=CARTESIAN_POINT('Ctrl Pts',(0.683893435765135,-0.271333802424689,
2.1475));
#53859=CARTESIAN_POINT('Ctrl Pts',(0.696998727473395,-0.239040247593054,
2.1475));
#53860=CARTESIAN_POINT('Ctrl Pts',(0.706401272193133,-0.215870859209857,
2.1475));
#53861=CARTESIAN_POINT('Ctrl Pts',(0.714632351997429,-0.192216505193648,
2.1475));
#53862=CARTESIAN_POINT('Ctrl Pts',(0.721667468561761,-0.168170826670213,
2.1475));
#53863=CARTESIAN_POINT('Ctrl Pts',(0.724957297731772,-0.156926354187669,
2.1475));
#53864=CARTESIAN_POINT('Ctrl Pts',(0.727985421385293,-0.1455962292866,2.1475));
#53865=CARTESIAN_POINT('Ctrl Pts',(0.730748372576983,-0.13418971384335,
2.1475));
#53866=CARTESIAN_POINT('Ctrl Pts',(0.732573304081957,-0.126655701133689,
2.1475));
#53867=CARTESIAN_POINT('Ctrl Pts',(0.734282538299918,-0.119088358725395,
2.1475));
#53868=CARTESIAN_POINT('Ctrl Pts',(0.735874921113159,-0.111490329588116,
2.1475));
#53869=CARTESIAN_POINT('Ctrl Pts',(0.737355097989788,-0.104427689283639,
2.1475));
#53870=CARTESIAN_POINT('Ctrl Pts',(0.738732308322656,-0.0973480380322194,
2.1475));
#53871=CARTESIAN_POINT('Ctrl Pts',(0.74000621129757,-0.090254603420933,
2.1475));
#53872=CARTESIAN_POINT('Ctrl Pts',(0.746406749010265,-0.0546146868526241,
2.1475));
#53873=CARTESIAN_POINT('Ctrl Pts',(0.750204865999736,-0.0186215654781291,
2.1475));
#53874=CARTESIAN_POINT('Ctrl Pts',(0.751350950426485,0.0174402270492316,
2.1475));
#53875=CARTESIAN_POINT('Ctrl Pts',(0.75235059886048,0.0488943796278962,
2.1475));
#53876=CARTESIAN_POINT('Ctrl Pts',(0.751332104048278,0.0804017898196976,
2.1475));
#53877=CARTESIAN_POINT('Ctrl Pts',(0.748351764615436,0.111783286065349,
2.1475));
#53878=CARTESIAN_POINT('Ctrl Pts',(0.746587659322543,0.130358439960856,
2.1475));
#53879=CARTESIAN_POINT('Ctrl Pts',(0.744135577432054,0.148889565682442,
2.1475));
#53880=CARTESIAN_POINT('Ctrl Pts',(0.741001939024339,0.167339239948629,
2.1475));
#53881=CARTESIAN_POINT('Ctrl Pts',(0.739443648103443,0.176513865786667,
2.1475));
#53882=CARTESIAN_POINT('Ctrl Pts',(0.737715946431412,0.185671312975827,
2.1475));
#53883=CARTESIAN_POINT('Ctrl Pts',(0.735824903550453,0.194782575820964,
2.1475));
#53884=CARTESIAN_POINT('Ctrl Pts',(0.728435000820851,0.23038798003859,2.1475));
#53885=CARTESIAN_POINT('Ctrl Pts',(0.718543897721654,0.265363085334939,
2.1475));
#53886=CARTESIAN_POINT('Ctrl Pts',(0.706253565541109,0.29944106174563,2.1475));
#53887=CARTESIAN_POINT('Ctrl Pts',(0.695958937871222,0.327985455317563,
2.1475));
#53888=CARTESIAN_POINT('Ctrl Pts',(0.683979973451509,0.355900995416786,
2.1475));
#53889=CARTESIAN_POINT('Ctrl Pts',(0.670348680947668,0.383027498229693,
2.1475));
#53890=CARTESIAN_POINT('Ctrl Pts',(0.662930091155104,0.397790617487756,
2.1475));
#53891=CARTESIAN_POINT('Ctrl Pts',(0.655021659947315,0.412319921069258,
2.1475));
#53892=CARTESIAN_POINT('Ctrl Pts',(0.646640126270176,0.426597056225371,
2.1475));
#53893=CARTESIAN_POINT('Ctrl Pts',(0.641911494744018,0.434651824481754,
2.1475));
#53894=CARTESIAN_POINT('Ctrl Pts',(0.637032242582384,0.44262631047491,2.1475));
#53895=CARTESIAN_POINT('Ctrl Pts',(0.632005108758899,0.450517044624497,
2.1475));
#53896=CARTESIAN_POINT('Ctrl Pts',(0.628031056722689,0.456754831247137,
2.1475));
#53897=CARTESIAN_POINT('Ctrl Pts',(0.623965446459039,0.462938715871801,
2.1475));
#53898=CARTESIAN_POINT('Ctrl Pts',(0.619816661607203,0.469057313504708,
2.1475));
#53899=CARTESIAN_POINT('Ctrl Pts',(0.599259679759847,0.499374600364076,
2.1475));
#53900=CARTESIAN_POINT('Ctrl Pts',(0.576621974739516,0.52815831445839,2.1475));
#53901=CARTESIAN_POINT('Ctrl Pts',(0.552123780088927,0.555233296369141,
2.1475));
#53902=CARTESIAN_POINT('Ctrl Pts',(0.527504999689496,0.582441547568308,
2.1475));
#53903=CARTESIAN_POINT('Ctrl Pts',(0.501006647273973,0.607925183051395,
2.1475));
#53904=CARTESIAN_POINT('Ctrl Pts',(0.472807519465647,0.631480354457914,
2.1475));
#53905=CARTESIAN_POINT('Ctrl Pts',(0.455234045944165,0.646159751062663,
2.1475));
#53906=CARTESIAN_POINT('Ctrl Pts',(0.436999200557785,0.66008962575319,2.1475));
#53907=CARTESIAN_POINT('Ctrl Pts',(0.418139433688274,0.673212941048261,
2.1475));
#53908=CARTESIAN_POINT('',(-0.7925,-9.70532588324278E-17,2.1475));
#53909=CARTESIAN_POINT('Origin',(0.,0.,2.1475));
#53910=CARTESIAN_POINT('',(-0.269045505528518,0.74544573781992,2.1475));
#53911=CARTESIAN_POINT('Origin',(0.,0.,2.1475));
#53912=CARTESIAN_POINT('Ctrl Pts',(-0.26905776807643,0.745453775914814,
2.1475));
#53913=CARTESIAN_POINT('Ctrl Pts',(-0.290441959207503,0.736475484699571,
2.1475));
#53914=CARTESIAN_POINT('Ctrl Pts',(-0.311396350827975,0.726569175411544,
2.1475));
#53915=CARTESIAN_POINT('Ctrl Pts',(-0.331855269122231,0.715747333928717,
2.1475));
#53916=CARTESIAN_POINT('Ctrl Pts',(-0.360321255985201,0.700690115699845,
2.1475));
#53917=CARTESIAN_POINT('Ctrl Pts',(-0.387829046120874,0.683861250117464,
2.1475));
#53918=CARTESIAN_POINT('Ctrl Pts',(-0.414237112173797,0.665381488245243,
2.1475));
#53919=CARTESIAN_POINT('Ctrl Pts',(-0.423486150408677,0.658909222393396,
2.1475));
#53920=CARTESIAN_POINT('Ctrl Pts',(-0.432600109161616,0.652234251657612,
2.1475));
#53921=CARTESIAN_POINT('Ctrl Pts',(-0.441572263629033,0.645361178051106,
2.1475));
#53922=CARTESIAN_POINT('Ctrl Pts',(-0.448544286378795,0.64002029524315,
2.1475));
#53923=CARTESIAN_POINT('Ctrl Pts',(-0.455427404303372,0.634562177123534,
2.1475));
#53924=CARTESIAN_POINT('Ctrl Pts',(-0.462212578349833,0.628994443678651,
2.1475));
#53925=CARTESIAN_POINT('Ctrl Pts',(-0.491850576505366,0.604674290291282,
2.1475));
#53926=CARTESIAN_POINT('Ctrl Pts',(-0.51966025566805,0.578238020468965,
2.1475));
#53927=CARTESIAN_POINT('Ctrl Pts',(-0.545395837156543,0.549886756197395,
2.1475));
#53928=CARTESIAN_POINT('Ctrl Pts',(-0.556375006365601,0.537791699092607,
2.1475));
#53929=CARTESIAN_POINT('Ctrl Pts',(-0.56697609741352,0.525347612886411,
2.1475));
#53930=CARTESIAN_POINT('Ctrl Pts',(-0.577177055036603,0.512568207937034,
2.1475));
#53931=CARTESIAN_POINT('Ctrl Pts',(-0.583958944968145,0.504072092085993,
2.1475));
#53932=CARTESIAN_POINT('Ctrl Pts',(-0.590566362811514,0.495424056770332,
2.1475));
#53933=CARTESIAN_POINT('Ctrl Pts',(-0.596976043364239,0.486651310852331,
2.1475));
#53934=CARTESIAN_POINT('Ctrl Pts',(-0.603524360378642,0.477688817185865,
2.1475));
#53935=CARTESIAN_POINT('Ctrl Pts',(-0.609869779183852,0.468592114455762,
2.1475));
#53936=CARTESIAN_POINT('Ctrl Pts',(-0.616006748809266,0.459366327752623,
2.1475));
#53937=CARTESIAN_POINT('Ctrl Pts',(-0.636008881653145,0.429296859841088,
2.1475));
#53938=CARTESIAN_POINT('Ctrl Pts',(-0.653800269885214,0.397857951627114,
2.1475));
#53939=CARTESIAN_POINT('Ctrl Pts',(-0.66930133326429,0.365313993663925,
2.1475));
#53940=CARTESIAN_POINT('Ctrl Pts',(-0.679860140869924,0.343146134436731,
2.1475));
#53941=CARTESIAN_POINT('Ctrl Pts',(-0.689355332541431,0.320464886542413,
2.1475));
#53942=CARTESIAN_POINT('Ctrl Pts',(-0.697748537607775,0.2973497108852,2.1475));
#53943=CARTESIAN_POINT('Ctrl Pts',(-0.70436467793553,0.279128632686827,
2.1475));
#53944=CARTESIAN_POINT('Ctrl Pts',(-0.710295869028216,0.26063783511346,
2.1475));
#53945=CARTESIAN_POINT('Ctrl Pts',(-0.715518243297554,0.241916050684857,
2.1475));
#53946=CARTESIAN_POINT('Ctrl Pts',(-0.717479128438073,0.23488643790785,
2.1475));
#53947=CARTESIAN_POINT('Ctrl Pts',(-0.719339678282086,0.2278250821791,2.1475));
#53948=CARTESIAN_POINT('Ctrl Pts',(-0.721095798426092,0.220746636408961,
2.1475));
#53949=CARTESIAN_POINT('Ctrl Pts',(-0.729648138435318,0.186274464804014,
2.1475));
#53950=CARTESIAN_POINT('Ctrl Pts',(-0.735750164426192,0.151319796048384,
2.1475));
#53951=CARTESIAN_POINT('Ctrl Pts',(-0.739309420613415,0.116128196525184,
2.1475));
#53952=CARTESIAN_POINT('Ctrl Pts',(-0.739584191889496,0.113411437685793,
2.1475));
#53953=CARTESIAN_POINT('Ctrl Pts',(-0.739843783453088,0.110693263463404,
2.1475));
#53954=CARTESIAN_POINT('Ctrl Pts',(-0.740088139783114,0.107973785712775,
2.1475));
#53955=CARTESIAN_POINT('Ctrl Pts',(-0.742817047135923,0.0776033720276509,
2.1475));
#53956=CARTESIAN_POINT('Ctrl Pts',(-0.74364816402632,0.0470699923217768,
2.1475));
#53957=CARTESIAN_POINT('Ctrl Pts',(-0.742599986958386,0.0165488238822319,
2.1475));
#53958=CARTESIAN_POINT('Ctrl Pts',(-0.7419704156394,-0.00178324315047445,
2.1475));
#53959=CARTESIAN_POINT('Ctrl Pts',(-0.740662321376881,-0.020110842121331,
2.1475));
#53960=CARTESIAN_POINT('Ctrl Pts',(-0.738674988083457,-0.038394449672262,
2.1475));
#53961=CARTESIAN_POINT('Ctrl Pts',(-0.737624385864582,-0.0480600647583613,
2.1475));
#53962=CARTESIAN_POINT('Ctrl Pts',(-0.736383083229925,-0.0577174697986878,
2.1475));
#53963=CARTESIAN_POINT('Ctrl Pts',(-0.734955315195305,-0.0673329290467907,
2.1475));
#53964=CARTESIAN_POINT('Ctrl Pts',(-0.729825818210465,-0.101878084859947,
2.1475));
#53965=CARTESIAN_POINT('Ctrl Pts',(-0.722288379849397,-0.13594922305856,
2.1475));
#53966=CARTESIAN_POINT('Ctrl Pts',(-0.712387643908391,-0.169286210566026,
2.1475));
#53967=CARTESIAN_POINT('Ctrl Pts',(-0.704219970383048,-0.196787765188011,
2.1475));
#53968=CARTESIAN_POINT('Ctrl Pts',(-0.694442927041613,-0.223789957726689,
2.1475));
#53969=CARTESIAN_POINT('Ctrl Pts',(-0.683056846723072,-0.250136548529342,
2.1475));
#53970=CARTESIAN_POINT('Ctrl Pts',(-0.676729068714859,-0.264778582768371,
2.1475));
#53971=CARTESIAN_POINT('Ctrl Pts',(-0.669903919231193,-0.279217909485822,
2.1475));
#53972=CARTESIAN_POINT('Ctrl Pts',(-0.662594838107065,-0.293431932187759,
2.1475));
#53973=CARTESIAN_POINT('Ctrl Pts',(-0.658703530129136,-0.300999386837555,
2.1475));
#53974=CARTESIAN_POINT('Ctrl Pts',(-0.654675027469965,-0.308502953737097,
2.1475));
#53975=CARTESIAN_POINT('Ctrl Pts',(-0.650511183593094,-0.315939021603285,
2.1475));
#53976=CARTESIAN_POINT('Ctrl Pts',(-0.647373225960974,-0.321542993943189,
2.1475));
#53977=CARTESIAN_POINT('Ctrl Pts',(-0.644159097881625,-0.327107209853852,
2.1475));
#53978=CARTESIAN_POINT('Ctrl Pts',(-0.640874688920018,-0.332622176281529,
2.1475));
#53979=CARTESIAN_POINT('Ctrl Pts',(-0.623260408432555,-0.36219893321759,
2.1475));
#53980=CARTESIAN_POINT('Ctrl Pts',(-0.60359160098753,-0.390427811114693,
2.1475));
#53981=CARTESIAN_POINT('Ctrl Pts',(-0.58204045909045,-0.417108106849397,
2.1475));
#53982=CARTESIAN_POINT('Ctrl Pts',(-0.560812811764996,-0.443387916573627,
2.1475));
#53983=CARTESIAN_POINT('Ctrl Pts',(-0.537758021946897,-0.46816609483233,
2.1475));
#53984=CARTESIAN_POINT('Ctrl Pts',(-0.513006243791438,-0.491215307380577,
2.1475));
#53985=CARTESIAN_POINT('Ctrl Pts',(-0.498618300449934,-0.504613567583442,
2.1475));
#53986=CARTESIAN_POINT('Ctrl Pts',(-0.483656376131934,-0.517426889096619,
2.1475));
#53987=CARTESIAN_POINT('Ctrl Pts',(-0.468142317532559,-0.529603335559025,
2.1475));
#53988=CARTESIAN_POINT('Ctrl Pts',(-0.308141029750816,0.636149375763356,
0.750549949443909));
#53989=CARTESIAN_POINT('Ctrl Pts',(-0.413294916605362,0.585214440963209,
0.7544961360274));
#53990=CARTESIAN_POINT('Ctrl Pts',(-0.597758033783181,0.430253045149882,
0.762388509194384));
#53991=CARTESIAN_POINT('Ctrl Pts',(-0.730464614175445,0.0939443613281403,
0.774227068944859));
#53992=CARTESIAN_POINT('Ctrl Pts',(-0.687181523831969,-0.264910506517124,
0.786065628695335));
#53993=CARTESIAN_POINT('Ctrl Pts',(-0.478355287135876,-0.559987389938686,
0.79790418844581));
#53994=CARTESIAN_POINT('Ctrl Pts',(-0.154284606478325,-0.720136019609621,
0.809742748196285));
#53995=CARTESIAN_POINT('Ctrl Pts',(0.206953274654826,-0.706806483749897,
0.821581307946761));
#53996=CARTESIAN_POINT('Ctrl Pts',(0.518334654870034,-0.523194014936019,
0.833419867697235));
#53997=CARTESIAN_POINT('Ctrl Pts',(0.704843009111363,-0.213540991323109,
0.845258427447713));
#53998=CARTESIAN_POINT('Ctrl Pts',(0.72154704261594,0.147557810200025,0.857096987198186));
#53999=CARTESIAN_POINT('Ctrl Pts',(0.564422240537776,0.473107596474913,
0.868935546948663));
#54000=CARTESIAN_POINT('Ctrl Pts',(0.271321884484909,0.684680839711599,
0.880774106699136));
#54001=CARTESIAN_POINT('Ctrl Pts',(-0.0871429660742197,0.731306659067973,
0.892612666449614));
#54002=CARTESIAN_POINT('Ctrl Pts',(-0.424614090524265,0.601752641869639,
0.904451226200088));
#54003=CARTESIAN_POINT('Ctrl Pts',(-0.659790954477945,0.327229660076594,
0.916289785950563));
#54004=CARTESIAN_POINT('Ctrl Pts',(-0.736016819052472,-0.026126571618046,
0.928128345701039));
#54005=CARTESIAN_POINT('Ctrl Pts',(-0.63492802922278,-0.373188632550485,
0.939966905451515));
#54006=CARTESIAN_POINT('Ctrl Pts',(-0.380877998557793,-0.630345386040242,
0.951805465201989));
#54007=CARTESIAN_POINT('Ctrl Pts',(-0.0350702127852755,-0.735644912405828,
0.963644024952465));
#54008=CARTESIAN_POINT('Ctrl Pts',(0.319186378418513,-0.663719377496494,
0.97548258470294));
#54009=CARTESIAN_POINT('Ctrl Pts',(0.596547412907388,-0.43189644669194,
0.987321144453416));
#54010=CARTESIAN_POINT('Ctrl Pts',(0.730193525854251,-0.0960248470611938,
0.99915970420389));
#54011=CARTESIAN_POINT('Ctrl Pts',(0.68792787877927,0.262980208441528,1.01099826395437));
#54012=CARTESIAN_POINT('Ctrl Pts',(0.47993273725243,0.558630400335474,1.02283682370484));
#54013=CARTESIAN_POINT('Ctrl Pts',(0.156316449407645,0.71970030157465,1.03467538345532));
#54014=CARTESIAN_POINT('Ctrl Pts',(-0.204958213586156,0.707386377546527,
1.04651394320579));
#54015=CARTESIAN_POINT('Ctrl Pts',(-0.516856158218931,0.524655189777677,
1.05835250295627));
#54016=CARTESIAN_POINT('Ctrl Pts',(-0.704237692836986,0.215528718361633,
1.07019106270674));
#54017=CARTESIAN_POINT('Ctrl Pts',(-0.721960516972989,-0.145521023852598,
1.08202962245722));
#54018=CARTESIAN_POINT('Ctrl Pts',(-0.565755004731942,-0.471513129267208,
1.09386818220769));
#54019=CARTESIAN_POINT('Ctrl Pts',(-0.273252805267132,-0.683912465791199,
1.10570674195817));
#54020=CARTESIAN_POINT('Ctrl Pts',(0.0850790409901614,-0.7315496655969,
1.11754530170865));
#54021=CARTESIAN_POINT('Ctrl Pts',(0.422914397879838,-0.602948396230368,
1.12938386145912));
#54022=CARTESIAN_POINT('Ctrl Pts',(0.658864962009067,-0.329090137025705,
1.14122242120959));
#54023=CARTESIAN_POINT('Ctrl Pts',(0.736087612291053,0.0240496046218443,
1.15306098096007));
#54024=CARTESIAN_POINT('Ctrl Pts',(0.635978551456582,0.371395528430276,
1.16489954071055));
#54025=CARTESIAN_POINT('Ctrl Pts',(0.382655168196356,0.629268129419748,
1.17673810046102));
#54026=CARTESIAN_POINT('Ctrl Pts',(0.0371458893840861,0.735543023454563,
1.1885766602115));
#54027=CARTESIAN_POINT('Ctrl Pts',(-0.317312248253455,0.664617403894264,
1.20041521996197));
#54028=CARTESIAN_POINT('Ctrl Pts',(-0.595326328143767,0.433578043112969,
1.21225377971245));
#54029=CARTESIAN_POINT('Ctrl Pts',(-0.729919659362832,0.0980848985647673,
1.22409233946292));
#54030=CARTESIAN_POINT('Ctrl Pts',(-0.688667208081245,-0.26103799141963,
1.2359308992134));
#54031=CARTESIAN_POINT('Ctrl Pts',(-0.481507149662053,-0.557273919428443,
1.24776945896388));
#54032=CARTESIAN_POINT('Ctrl Pts',(-0.158346651432958,-0.719256348203324,
1.25960801871435));
#54033=CARTESIAN_POINT('Ctrl Pts',(0.202961320248067,-0.707961905001939,
1.27144657846483));
#54034=CARTESIAN_POINT('Ctrl Pts',(0.515373647430983,-0.526111547092912,
1.2832851382153));
#54035=CARTESIAN_POINT('Ctrl Pts',(0.703626717974851,-0.217515052818769,
1.29512369796578));
#54036=CARTESIAN_POINT('Ctrl Pts',(0.722368268691099,0.143483242363127,
1.30696225771625));
#54037=CARTESIAN_POINT('Ctrl Pts',(0.567083251096378,0.469914825023403,
1.31880081746673));
#54038=CARTESIAN_POINT('Ctrl Pts',(0.275181556922342,0.683138688101186,
1.3306393772172));
#54039=CARTESIAN_POINT('Ctrl Pts',(-0.0830144418180345,0.731786826132074,
1.34247793696768));
#54040=CARTESIAN_POINT('Ctrl Pts',(-0.421211336145891,0.604139360373918,
1.35431649671815));
#54041=CARTESIAN_POINT('Ctrl Pts',(-0.657933724269358,0.33094798823964,
1.36615505646863));
#54042=CARTESIAN_POINT('Ctrl Pts',(-0.736152544097779,-0.0219724434048499,
1.3779936162191));
#54043=CARTESIAN_POINT('Ctrl Pts',(-0.637024010013693,-0.3695994685019,
1.38983217596958));
#54044=CARTESIAN_POINT('Ctrl Pts',(-0.384429290883511,-0.62818586163779,
1.40167073572005));
#54045=CARTESIAN_POINT('Ctrl Pts',(-0.0392212702694481,-0.735435278191946,
1.41350929547053));
#54046=CARTESIAN_POINT('Ctrl Pts',(0.315435591559856,-0.665510138185811,
1.425347855221));
#54047=CARTESIAN_POINT('Ctrl Pts',(0.594100503158886,-0.435256187316358,
1.43718641497148));
#54048=CARTESIAN_POINT('Ctrl Pts',(0.729639980990038,-0.100144169034792,
1.44902497472195));
#54049=CARTESIAN_POINT('Ctrl Pts',(0.689401053958178,0.259093695894295,
1.46086353447243));
#54050=CARTESIAN_POINT('Ctrl Pts',(0.483077728136633,0.555913001313301,
1.47270209422291));
#54051=CARTESIAN_POINT('Ctrl Pts',(0.160375592643109,0.718806667842741,
1.48454065397338));
#54052=CARTESIAN_POINT('Ctrl Pts',(-0.200962810856885,0.708531795407456,
1.49637921372385));
#54053=CARTESIAN_POINT('Ctrl Pts',(-0.51388703304889,0.527563715313158,
1.50821777347433));
#54054=CARTESIAN_POINT('Ctrl Pts',(-0.70301014057808,0.219499655341875,
1.52005633322481));
#54055=CARTESIAN_POINT('Ctrl Pts',(-0.722770268647641,-0.141444318407737,
1.53189489297528));
#54056=CARTESIAN_POINT('Ctrl Pts',(-0.568406982135528,-0.468312779144872,
1.54373345272576));
#54057=CARTESIAN_POINT('Ctrl Pts',(-0.277108117480876,-0.682359471009978,
1.55557201247623));
#54058=CARTESIAN_POINT('Ctrl Pts',(0.0809491816544183,-0.732018159911551,
1.56741057222671));
#54059=CARTESIAN_POINT('Ctrl Pts',(0.419504920572478,-0.605325514137882,
1.57924913197718));
#54060=CARTESIAN_POINT('Ctrl Pts',(0.656997247819542,-0.33280320432406,
1.59108769172766));
#54061=CARTESIAN_POINT('Ctrl Pts',(0.736211614387408,0.0198951072351811,
1.60292625147813));
#54062=CARTESIAN_POINT('Ctrl Pts',(0.638064396351524,0.367800465686733,
1.61476481122861));
#54063=CARTESIAN_POINT('Ctrl Pts',(0.386200352603368,0.62709859200914,1.62660337097908));
#54064=CARTESIAN_POINT('Ctrl Pts',(0.0412963388606396,0.735321677123366,
1.63844193072956));
#54065=CARTESIAN_POINT('Ctrl Pts',(-0.313556423252151,0.666397573441058,
1.65028049048004));
#54066=CARTESIAN_POINT('Ctrl Pts',(-0.59286994772746,0.436930865850026,
1.66211905023051));
#54067=CARTESIAN_POINT('Ctrl Pts',(-0.729354492955569,0.102202642120141,
1.67395760998099));
#54068=CARTESIAN_POINT('Ctrl Pts',(-0.69012941057056,-0.257147337369736,
1.68579616973146));
#54069=CARTESIAN_POINT('Ctrl Pts',(-0.484644460168804,-0.554547656814542,
1.69763472948194));
#54070=CARTESIAN_POINT('Ctrl Pts',(-0.162403256883848,-0.718351264079303,
1.70947328923241));
#54071=CARTESIAN_POINT('Ctrl Pts',(0.198962701325951,-0.709096044222425,
1.72131184898289));
#54072=CARTESIAN_POINT('Ctrl Pts',(0.512396326909379,-0.529011682877222,
1.73315040873336));
#54073=CARTESIAN_POINT('Ctrl Pts',(0.702387965556207,-0.221482510128057,
1.74498896848384));
#54074=CARTESIAN_POINT('Ctrl Pts',(0.723166513641681,0.139404268220684,
1.75682752823431));
#54075=CARTESIAN_POINT('Ctrl Pts',(0.569726187309398,0.46670700438791,1.76866608798479));
#54076=CARTESIAN_POINT('Ctrl Pts',(0.279032471602733,0.681574820721842,
1.78050464773527));
#54077=CARTESIAN_POINT('Ctrl Pts',(-0.0788832769436621,0.732243665093515,
1.79234320748574));
#54078=CARTESIAN_POINT('Ctrl Pts',(-0.417795164746744,0.606506848077444,
1.80418176723622));
#54079=CARTESIAN_POINT('Ctrl Pts',(-0.656055540116142,0.334655770507442,
1.81602032698669));
#54080=CARTESIAN_POINT('Ctrl Pts',(-0.736264822689689,-0.0178176126541187,
1.82785888673717));
#54081=CARTESIAN_POINT('Ctrl Pts',(-0.639099702185964,-0.365998534307576,
1.83969744648764));
#54082=CARTESIAN_POINT('Ctrl Pts',(-0.387968339254434,-0.626006329194029,
1.85153600623812));
#54083=CARTESIAN_POINT('Ctrl Pts',(-0.043371078634514,-0.735202221147443,
1.86337456598859));
#54084=CARTESIAN_POINT('Ctrl Pts',(0.311674758291609,-0.667279702605622,
1.87521312573907));
#54085=CARTESIAN_POINT('Ctrl Pts',(0.591634671650319,-0.438602065356417,
1.88705168548954));
#54086=CARTESIAN_POINT('Ctrl Pts',(0.729063197527252,-0.104260301476294,
1.89889024524002));
#54087=CARTESIAN_POINT('Ctrl Pts',(0.690852272129496,0.255198931434154,
1.91072880499049));
#54088=CARTESIAN_POINT('Ctrl Pts',(0.486207333262819,0.553177896624332,
1.92256736474097));
#54089=CARTESIAN_POINT('Ctrl Pts',(0.16442962805144,0.71789014089361,1.93440592449145));
#54090=CARTESIAN_POINT('Ctrl Pts',(-0.196961007662504,0.709654646252797,
1.94624448424192));
#54091=CARTESIAN_POINT('Ctrl Pts',(-0.51090154072052,0.530455439643165,
1.9580830439924));
#54092=CARTESIAN_POINT('Ctrl Pts',(-0.701760198182685,0.223463598644677,
1.96992160374287));
#54093=CARTESIAN_POINT('Ctrl Pts',(-0.723556999886197,-0.137363102616563,
1.98176016349335));
#54094=CARTESIAN_POINT('Ctrl Pts',(-0.571040857364167,-0.465097524278119,
1.99359872324382));
#54095=CARTESIAN_POINT('Ctrl Pts',(-0.280954601492375,-0.680784722238707,
2.0054372829943));
#54096=CARTESIAN_POINT('Ctrl Pts',(0.0768167392428667,-0.732463381911148,
2.01727584274477));
#54097=CARTESIAN_POINT('Ctrl Pts',(0.416082091960603,-0.607683269644344,
2.02911440249525));
#54098=CARTESIAN_POINT('Ctrl Pts',(0.655108589511754,-0.336505836512168,
2.04095296224572));
#54099=CARTESIAN_POINT('Ctrl Pts',(0.736312206455239,0.0157403015675272,
2.0527915219962));
#54100=CARTESIAN_POINT('Ctrl Pts',(0.640129844349537,0.364193045069704,
2.06463008174667));
#54101=CARTESIAN_POINT('Ctrl Pts',(0.389733384979782,0.624910355165805,
2.07646864149715));
#54102=CARTESIAN_POINT('Ctrl Pts',(0.0454451798068112,0.735074392267673,
2.08830720124762));
#54103=CARTESIAN_POINT('Ctrl Pts',(-0.309790030899746,0.668161503213349,
2.1001457609981));
#54104=CARTESIAN_POINT('Ctrl Pts',(-0.590395841023348,0.440259893769033,
2.11198432074857));
#54105=CARTESIAN_POINT('Ctrl Pts',(-0.728763721120245,0.106336890902483,
2.12382288049905));
#54106=CARTESIAN_POINT('Ctrl Pts',(-0.691575347498768,-0.253290127215884,
2.13566144024952));
#54107=CARTESIAN_POINT('Ctrl Pts',(-0.555684412749315,-0.452220591560317,
2.14355381341651));
#54108=CARTESIAN_POINT('Ctrl Pts',(-0.468142317532544,-0.529603335559038,
2.1475));
#54109=CARTESIAN_POINT('Ctrl Pts',(-0.320586989147272,0.661843744693177,
0.767033299629272));
#54110=CARTESIAN_POINT('Ctrl Pts',(-0.429988090360872,0.608851524205057,
0.770979486212764));
#54111=CARTESIAN_POINT('Ctrl Pts',(-0.621901758568509,0.447631165598393,
0.778871859379747));
#54112=CARTESIAN_POINT('Ctrl Pts',(-0.759968419416597,0.0977388177416922,
0.790710419130224));
#54113=CARTESIAN_POINT('Ctrl Pts',(-0.714937104938856,-0.275610364989308,
0.802548978880698));
#54114=CARTESIAN_POINT('Ctrl Pts',(-0.497676279493137,-0.582605540865684,
0.814387538631174));
#54115=CARTESIAN_POINT('Ctrl Pts',(-0.160516233435894,-0.749222648116171,
0.826226098381648));
#54116=CARTESIAN_POINT('Ctrl Pts',(0.215312213597169,-0.735354726108332,
0.838064658132125));
#54117=CARTESIAN_POINT('Ctrl Pts',(0.539270432470003,-0.544326064347384,
0.8499032178826));
#54118=CARTESIAN_POINT('Ctrl Pts',(0.733311945816648,-0.222166011203247,
0.861741777633075));
#54119=CARTESIAN_POINT('Ctrl Pts',(0.75069066299747,0.153517738729713,0.873580337383551));
#54120=CARTESIAN_POINT('Ctrl Pts',(0.587219517141517,0.492216632167575,
0.885418897134026));
#54121=CARTESIAN_POINT('Ctrl Pts',(0.282280701492824,0.7123354170247,0.897257456884501));
#54122=CARTESIAN_POINT('Ctrl Pts',(-0.0906627109725972,0.760844474893665,
0.909096016634976));
#54123=CARTESIAN_POINT('Ctrl Pts',(-0.441764450974809,0.626057710732026,
0.920934576385453));
#54124=CARTESIAN_POINT('Ctrl Pts',(-0.686440217759186,0.34044661812312,
0.932773136135927));
#54125=CARTESIAN_POINT('Ctrl Pts',(-0.765744880428929,-0.0271818359877063,
0.944611695886403));
#54126=CARTESIAN_POINT('Ctrl Pts',(-0.660573067398221,-0.388261894854107,
0.956450255636878));
#54127=CARTESIAN_POINT('Ctrl Pts',(-0.396261837927992,-0.655805329127812,
0.968288815387354));
#54128=CARTESIAN_POINT('Ctrl Pts',(-0.0364867149781318,-0.765357952299986,
0.980127375137828));
#54129=CARTESIAN_POINT('Ctrl Pts',(0.33207846458085,-0.690527311609143,
0.991965934888305));
#54130=CARTESIAN_POINT('Ctrl Pts',(0.620642240152921,-0.449340944892484,
1.00380449463878));
#54131=CARTESIAN_POINT('Ctrl Pts',(0.759686381712126,-0.0999033352603849,
1.01564305438925));
#54132=CARTESIAN_POINT('Ctrl Pts',(0.715713605509338,0.273602101277356,
1.02748161413973));
#54133=CARTESIAN_POINT('Ctrl Pts',(0.499317443552999,0.581193741821753,
1.03932017389021));
#54134=CARTESIAN_POINT('Ctrl Pts',(0.162630143445403,0.748769331227273,
1.05115873364068));
#54135=CARTESIAN_POINT('Ctrl Pts',(-0.213236571084754,0.735958042084906,
1.06299729339116));
#54136=CARTESIAN_POINT('Ctrl Pts',(-0.53773221865205,0.545846256719961,
1.07483585314163));
#54137=CARTESIAN_POINT('Ctrl Pts',(-0.732682180536634,0.224234023460629,
1.08667441289211));
#54138=CARTESIAN_POINT('Ctrl Pts',(-0.751120837775958,-0.151398685635141,
1.09851297264258));
#54139=CARTESIAN_POINT('Ctrl Pts',(-0.588606112300871,-0.490557763688342,
1.11035153239306));
#54140=CARTESIAN_POINT('Ctrl Pts',(-0.284289613062813,-0.711536008124563,
1.12219009214353));
#54141=CARTESIAN_POINT('Ctrl Pts',(0.0885154229952094,-0.761097296569231,
1.13402865189401));
#54142=CARTESIAN_POINT('Ctrl Pts',(0.439996106954563,-0.627301762167098,
1.14586721164448));
#54143=CARTESIAN_POINT('Ctrl Pts',(0.685476824024146,-0.342382240600841,
1.15770577139496));
#54144=CARTESIAN_POINT('Ctrl Pts',(0.765818533039317,0.0250209793292831,
1.16954433114543));
#54145=CARTESIAN_POINT('Ctrl Pts',(0.661666020713264,0.386396366425159,
1.18138289089591));
#54146=CARTESIAN_POINT('Ctrl Pts',(0.398110788274175,0.654684561611774,
1.19322145064639));
#54147=CARTESIAN_POINT('Ctrl Pts',(0.0386462291194138,0.765251948006628,
1.20506001039686));
#54148=CARTESIAN_POINT('Ctrl Pts',(-0.330128637427446,0.691461609710464,
1.21689857014734));
#54149=CARTESIAN_POINT('Ctrl Pts',(-0.619371835208214,0.451090461774462,
1.22873712989781));
#54150=CARTESIAN_POINT('Ctrl Pts',(-0.759401453625842,0.102046593201571,
1.24057568964829));
#54151=CARTESIAN_POINT('Ctrl Pts',(-0.716482796665414,-0.271581437207322,
1.25241424939876));
#54152=CARTESIAN_POINT('Ctrl Pts',(-0.500955447211536,-0.57978247202048,
1.26425280914924));
#54153=CARTESIAN_POINT('Ctrl Pts',(-0.164742346274029,-0.748307446372957,
1.27609136889971));
#54154=CARTESIAN_POINT('Ctrl Pts',(0.211159022296708,-0.736556815361711,
1.28792992865019));
#54155=CARTESIAN_POINT('Ctrl Pts',(0.536189828564398,-0.547361436983983,
1.29976848840066));
#54156=CARTESIAN_POINT('Ctrl Pts',(0.732046528115873,-0.226300586889613,
1.31160704815114));
#54157=CARTESIAN_POINT('Ctrl Pts',(0.751545058775462,0.149278597204277,
1.32344560790161));
#54158=CARTESIAN_POINT('Ctrl Pts',(0.589988007153253,0.488894903193336,
1.33528416765209));
#54159=CARTESIAN_POINT('Ctrl Pts',(0.286296267893741,0.710730977194047,
1.34712272740256));
#54160=CARTESIAN_POINT('Ctrl Pts',(-0.0863674337030227,0.761344036128637,
1.35896128715304));
#54161=CARTESIAN_POINT('Ctrl Pts',(-0.438224257765704,0.628540829905892,
1.37079984690351));
#54162=CARTESIAN_POINT('Ctrl Pts',(-0.684507973159348,0.344315131288721,
1.38263840665399));
#54163=CARTESIAN_POINT('Ctrl Pts',(-0.765886087471892,-0.0228599206053984,
1.39447696640446));
#54164=CARTESIAN_POINT('Ctrl Pts',(-0.662753705827361,-0.38452776280158,
1.40631552615494));
#54165=CARTESIAN_POINT('Ctrl Pts',(-0.399956568601167,-0.653558580531132,
1.41815408590542));
#54166=CARTESIAN_POINT('Ctrl Pts',(-0.0408054356032438,-0.765139850862781,
1.42999264565589));
#54167=CARTESIAN_POINT('Ctrl Pts',(0.328176181697839,-0.692390401954935,
1.44183120540637));
#54168=CARTESIAN_POINT('Ctrl Pts',(0.618096498582505,-0.452836387002122,
1.45366976515684));
#54169=CARTESIAN_POINT('Ctrl Pts',(0.759110478913594,-0.104189038562902,
1.46550832490732));
#54170=CARTESIAN_POINT('Ctrl Pts',(0.717246282918362,0.269558610682131,
1.47734688465779));
#54171=CARTESIAN_POINT('Ctrl Pts',(0.502589462080611,0.578366585790198,
1.48918544440827));
#54172=CARTESIAN_POINT('Ctrl Pts',(0.166853237362585,0.747839603213625,
1.50102400415874));
#54173=CARTESIAN_POINT('Ctrl Pts',(-0.209079792182433,0.737149723905558,
1.51286256390922));
#54174=CARTESIAN_POINT('Ctrl Pts',(-0.534643169136526,0.548872258953521,
1.5247011236597));
#54175=CARTESIAN_POINT('Ctrl Pts',(-0.731405046871499,0.228365348430948,
1.53653968341017));
#54176=CARTESIAN_POINT('Ctrl Pts',(-0.751963295697072,-0.147157320162763,
1.54837824316065));
#54177=CARTESIAN_POINT('Ctrl Pts',(-0.591365204304262,-0.487228149937241,
1.56021680291112));
#54178=CARTESIAN_POINT('Ctrl Pts',(-0.288300643128581,-0.709920287162393,
1.5720553626616));
#54179=CARTESIAN_POINT('Ctrl Pts',(0.0842187567215935,-0.761584713586976,
1.58389392241207));
#54180=CARTESIAN_POINT('Ctrl Pts',(0.436448919274245,-0.629774892971634,
1.59573248216255));
#54181=CARTESIAN_POINT('Ctrl Pts',(0.683533671990508,-0.346245280412978,
1.60757104191302));
#54182=CARTESIAN_POINT('Ctrl Pts',(0.765947543637971,0.0206986798624194,
1.6194096016635));
#54183=CARTESIAN_POINT('Ctrl Pts',(0.663836113852885,0.382656097426644,
1.63124816141397));
#54184=CARTESIAN_POINT('Ctrl Pts',(0.401799164326967,0.652427395576886,
1.64308672116445));
#54185=CARTESIAN_POINT('Ctrl Pts',(0.042964317179197,0.765021661394247,
1.65492528091492));
#54186=CARTESIAN_POINT('Ctrl Pts',(-0.326221112908865,0.693313681132567,
1.6667638406654));
#54187=CARTESIAN_POINT('Ctrl Pts',(-0.616816240445319,0.454578706580051,
1.67860240041587));
#54188=CARTESIAN_POINT('Ctrl Pts',(-0.758813459884736,0.106330654332819,
1.69044096016635));
#54189=CARTESIAN_POINT('Ctrl Pts',(-0.718004058192813,-0.267533637832218,
1.70227951991683));
#54190=CARTESIAN_POINT('Ctrl Pts',(-0.504219475147683,-0.576946094392606,
1.7141180796673));
#54191=CARTESIAN_POINT('Ctrl Pts',(-0.168962799904339,-0.74736580548054,
1.72595663941778));
#54192=CARTESIAN_POINT('Ctrl Pts',(0.206998897298017,-0.73773676299239,
1.73779519916825));
#54193=CARTESIAN_POINT('Ctrl Pts',(0.533092252683253,-0.550378710600425,
1.74963375891873));
#54194=CARTESIAN_POINT('Ctrl Pts',(0.730757741911345,-0.230428291643451,
1.7614723186692));
#54195=CARTESIAN_POINT('Ctrl Pts',(0.752375545210572,0.145034871400566,
1.77331087841968));
#54196=CARTESIAN_POINT('Ctrl Pts',(0.592737692788189,0.485557517191581,
1.78514943817015));
#54197=CARTESIAN_POINT('Ctrl Pts',(0.29030272280774,0.709103944484463,1.79698799792063));
#54198=CARTESIAN_POINT('Ctrl Pts',(-0.0820694091594656,0.761819327028042,
1.8088265576711));
#54199=CARTESIAN_POINT('Ctrl Pts',(-0.434670105616121,0.631003941538025,
1.82066511742158));
#54200=CARTESIAN_POINT('Ctrl Pts',(-0.68255392827532,0.348172672605466,
1.83250367717205));
#54201=CARTESIAN_POINT('Ctrl Pts',(-0.76600290104831,-0.0185372743097382,
1.84434223692253));
#54202=CARTESIAN_POINT('Ctrl Pts',(-0.664913236171123,-0.380781385201656,
1.856180796673));
#54203=CARTESIAN_POINT('Ctrl Pts',(-0.403638560780521,-0.651291015759056,
1.86801935642348));
#54204=CARTESIAN_POINT('Ctrl Pts',(-0.045122856656748,-0.76489738053594,
1.87985791617396));
#54205=CARTESIAN_POINT('Ctrl Pts',(0.324263446626085,-0.694231439904046,
1.89169647592443));
#54206=CARTESIAN_POINT('Ctrl Pts',(0.615531070993343,-0.456317406611175,
1.90353503567491));
#54207=CARTESIAN_POINT('Ctrl Pts',(0.758510398898692,-0.108471423506639,
1.91537359542538));
#54208=CARTESIAN_POINT('Ctrl Pts',(0.718756116466056,0.2655065348754,1.92721215517586));
#54209=CARTESIAN_POINT('Ctrl Pts',(0.505845473412291,0.575521008951734,
1.93905071492633));
#54210=CARTESIAN_POINT('Ctrl Pts',(0.171071017145122,0.746886057315075,
1.95088927467681));
#54211=CARTESIAN_POINT('Ctrl Pts',(-0.204916354297241,0.738317927218373,
1.96272783442729));
#54212=CARTESIAN_POINT('Ctrl Pts',(-0.53153709138554,0.551880781373112,
1.97456639417776));
#54213=CARTESIAN_POINT('Ctrl Pts',(-0.73010461872186,0.232489397245945,
1.98640495392823));
#54214=CARTESIAN_POINT('Ctrl Pts',(-0.752781803375976,-0.142911262169087,
1.99824351367871));
#54215=CARTESIAN_POINT('Ctrl Pts',(-0.594105462977449,-0.483883029432169,
2.01008207342919));
#54216=CARTESIAN_POINT('Ctrl Pts',(-0.29230248841691,-0.708281933556404,
2.02192063317966));
#54217=CARTESIAN_POINT('Ctrl Pts',(0.0799194030405367,-0.76204791831005,
2.03375919293014));
#54218=CARTESIAN_POINT('Ctrl Pts',(0.432887841024017,-0.632227879318738,
2.04559775268061));
#54219=CARTESIAN_POINT('Ctrl Pts',(0.681568729895938,-0.35009746363592,
2.05743631243109));
#54220=CARTESIAN_POINT('Ctrl Pts',(0.76605219866617,0.0163760596629542,
2.06927487218156));
#54221=CARTESIAN_POINT('Ctrl Pts',(0.665984986255429,0.378902971414387,
2.08111343193203));
#54222=CARTESIAN_POINT('Ctrl Pts',(0.405474897523,0.650150774830491,2.09295199168251));
#54223=CARTESIAN_POINT('Ctrl Pts',(0.0472807317393077,0.764764388588309,
2.10479055143299));
#54224=CARTESIAN_POINT('Ctrl Pts',(-0.32230259421896,0.695148856848125,
2.11662911118346));
#54225=CARTESIAN_POINT('Ctrl Pts',(-0.614242203421617,0.458042195483833,
2.12846767093394));
#54226=CARTESIAN_POINT('Ctrl Pts',(-0.758198826500429,0.110631887344821,
2.14030623068441));
#54227=CARTESIAN_POINT('Ctrl Pts',(-0.719508397185533,-0.263520633167659,
2.15214479043489));
#54228=CARTESIAN_POINT('Ctrl Pts',(-0.578128764427879,-0.470485991417495,
2.16003716360187));
#54229=CARTESIAN_POINT('Ctrl Pts',(-0.487050803301172,-0.55099426040902,
2.16398335018536));
#54230=CARTESIAN_POINT('Ctrl Pts',(-0.333032948543728,0.687538113622998,
0.783516649814636));
#54231=CARTESIAN_POINT('Ctrl Pts',(-0.446681264116382,0.632488607446904,
0.787462836398128));
#54232=CARTESIAN_POINT('Ctrl Pts',(-0.646045483353837,0.465009286046903,
0.795355209565111));
#54233=CARTESIAN_POINT('Ctrl Pts',(-0.78947222465775,0.101533274155245,
0.807193769315587));
#54234=CARTESIAN_POINT('Ctrl Pts',(-0.742692686045743,-0.286310223461493,
0.819032329066061));
#54235=CARTESIAN_POINT('Ctrl Pts',(-0.516997271850398,-0.605223691792682,
0.830870888816538));
#54236=CARTESIAN_POINT('Ctrl Pts',(-0.166747860393462,-0.778309276622721,
0.842709448567012));
#54237=CARTESIAN_POINT('Ctrl Pts',(0.223671152539511,-0.763902968466767,
0.854548008317489));
#54238=CARTESIAN_POINT('Ctrl Pts',(0.560206210069973,-0.56545811375875,
0.866386568067964));
#54239=CARTESIAN_POINT('Ctrl Pts',(0.761780882521931,-0.230791031083385,
0.878225127818439));
#54240=CARTESIAN_POINT('Ctrl Pts',(0.779834283379,0.159477667259401,0.890063687568915));
#54241=CARTESIAN_POINT('Ctrl Pts',(0.610016793745258,0.511325667860236,
0.901902247319389));
#54242=CARTESIAN_POINT('Ctrl Pts',(0.293239518500739,0.739989994337803,
0.913740807069865));
#54243=CARTESIAN_POINT('Ctrl Pts',(-0.0941824558709746,0.790382290719356,
0.925579366820341));
#54244=CARTESIAN_POINT('Ctrl Pts',(-0.458914811425353,0.650362779594414,
0.937417926570816));
#54245=CARTESIAN_POINT('Ctrl Pts',(-0.713089481040427,0.353663576169647,
0.949256486321291));
#54246=CARTESIAN_POINT('Ctrl Pts',(-0.795472941805385,-0.0282371003573665,
0.961095046071767));
#54247=CARTESIAN_POINT('Ctrl Pts',(-0.686218105573663,-0.40333515715773,
0.972933605822241));
#54248=CARTESIAN_POINT('Ctrl Pts',(-0.411645677298192,-0.681265272215381,
0.984772165572718));
#54249=CARTESIAN_POINT('Ctrl Pts',(-0.0379032171709881,-0.795070992194145,
0.996610725323191));
#54250=CARTESIAN_POINT('Ctrl Pts',(0.344970550743188,-0.717335245721791,
1.00844928507367));
#54251=CARTESIAN_POINT('Ctrl Pts',(0.644737067398454,-0.46678544309303,
1.02028784482414));
#54252=CARTESIAN_POINT('Ctrl Pts',(0.789179237570002,-0.103781823459575,
1.03212640457462));
#54253=CARTESIAN_POINT('Ctrl Pts',(0.743499332239405,0.284223994113184,
1.04396496432509));
#54254=CARTESIAN_POINT('Ctrl Pts',(0.518702149853569,0.603757083308034,
1.05580352407557));
#54255=CARTESIAN_POINT('Ctrl Pts',(0.16894383748316,0.777838360879895,1.06764208382604));
#54256=CARTESIAN_POINT('Ctrl Pts',(-0.221514928583353,0.764529706623286,
1.07948064357652));
#54257=CARTESIAN_POINT('Ctrl Pts',(-0.558608279085167,0.567037323662244,
1.091319203327));
#54258=CARTESIAN_POINT('Ctrl Pts',(-0.761126668236282,0.232939328559625,
1.10315776307747));
#54259=CARTESIAN_POINT('Ctrl Pts',(-0.780281158578927,-0.157276347417685,
1.11499632282795));
#54260=CARTESIAN_POINT('Ctrl Pts',(-0.6114572198698,-0.509602398109476,
1.12683488257842));
#54261=CARTESIAN_POINT('Ctrl Pts',(-0.295326420858495,-0.739159550457927,
1.1386734423289));
#54262=CARTESIAN_POINT('Ctrl Pts',(0.0919518050002577,-0.790644927541561,
1.15051200207937));
#54263=CARTESIAN_POINT('Ctrl Pts',(0.457077816029287,-0.651655128103828,
1.16235056182985));
#54264=CARTESIAN_POINT('Ctrl Pts',(0.712088686039225,-0.355674344175977,
1.17418912158032));
#54265=CARTESIAN_POINT('Ctrl Pts',(0.79554945378758,0.0259923540367214,
1.1860276813308));
#54266=CARTESIAN_POINT('Ctrl Pts',(0.687353489969946,0.401397204420044,
1.19786624108127));
#54267=CARTESIAN_POINT('Ctrl Pts',(0.413566408351994,0.6801009938038,1.20970480083175));
#54268=CARTESIAN_POINT('Ctrl Pts',(0.0401465688547416,0.794960872558695,
1.22154336058222));
#54269=CARTESIAN_POINT('Ctrl Pts',(-0.342945026601437,0.718305815526664,
1.2333819203327));
#54270=CARTESIAN_POINT('Ctrl Pts',(-0.643417342272661,0.468602880435955,
1.24522048008317));
#54271=CARTESIAN_POINT('Ctrl Pts',(-0.788883247888852,0.106008287838375,
1.25705903983365));
#54272=CARTESIAN_POINT('Ctrl Pts',(-0.744298385249583,-0.282124882995013,
1.26889759958412));
#54273=CARTESIAN_POINT('Ctrl Pts',(-0.520403744761019,-0.602291024612518,
1.2807361593346));
#54274=CARTESIAN_POINT('Ctrl Pts',(-0.171138041115101,-0.777358544542589,
1.29257471908508));
#54275=CARTESIAN_POINT('Ctrl Pts',(0.219356724345348,-0.765151725721485,
1.30441327883555));
#54276=CARTESIAN_POINT('Ctrl Pts',(0.557006009697813,-0.568611326875053,
1.31625183858603));
#54277=CARTESIAN_POINT('Ctrl Pts',(0.760466338256896,-0.235086120960459,
1.3280903983365));
#54278=CARTESIAN_POINT('Ctrl Pts',(0.780721848859823,0.155073952045427,
1.33992895808698));
#54279=CARTESIAN_POINT('Ctrl Pts',(0.612892763210127,0.507874981363269,
1.35176751783745));
#54280=CARTESIAN_POINT('Ctrl Pts',(0.29741097886514,0.738323266286908,1.36360607758793));
#54281=CARTESIAN_POINT('Ctrl Pts',(-0.0897204255880114,0.7909012461252,
1.37544463733841));
#54282=CARTESIAN_POINT('Ctrl Pts',(-0.455237179385516,0.652942299437866,
1.38728319708888));
#54283=CARTESIAN_POINT('Ctrl Pts',(-0.711082222049339,0.357682274337801,
1.39912175683936));
#54284=CARTESIAN_POINT('Ctrl Pts',(-0.795619630846004,-0.0237473978059473,
1.41096031658983));
#54285=CARTESIAN_POINT('Ctrl Pts',(-0.68848340164103,-0.399456057101259,
1.42279887634031));
#54286=CARTESIAN_POINT('Ctrl Pts',(-0.415483846318822,-0.678931299424474,
1.43463743609078));
#54287=CARTESIAN_POINT('Ctrl Pts',(-0.0423896009370397,-0.794844423533616,
1.44647599584126));
#54288=CARTESIAN_POINT('Ctrl Pts',(0.340916771835822,-0.719270665724059,
1.45831455559173));
#54289=CARTESIAN_POINT('Ctrl Pts',(0.642092494006125,-0.470416586687887,
1.47015311534221));
#54290=CARTESIAN_POINT('Ctrl Pts',(0.78858097683715,-0.108233908091011,
1.48199167509268));
#54291=CARTESIAN_POINT('Ctrl Pts',(0.745091511878546,0.280023525469966,
1.49383023484316));
#54292=CARTESIAN_POINT('Ctrl Pts',(0.52210119602459,0.600820170267094,1.50566879459363));
#54293=CARTESIAN_POINT('Ctrl Pts',(0.173330882082061,0.77687253858451,1.51750735434411));
#54294=CARTESIAN_POINT('Ctrl Pts',(-0.217196773507981,0.765767652403659,
1.52934591409458));
#54295=CARTESIAN_POINT('Ctrl Pts',(-0.555399305224161,0.570180802593885,
1.54118447384506));
#54296=CARTESIAN_POINT('Ctrl Pts',(-0.75979995316492,0.237231041520021,
1.55302303359554));
#54297=CARTESIAN_POINT('Ctrl Pts',(-0.781156322746504,-0.152870321917789,
1.56486159334601));
#54298=CARTESIAN_POINT('Ctrl Pts',(-0.614323426472996,-0.506143520729609,
1.57670015309648));
#54299=CARTESIAN_POINT('Ctrl Pts',(-0.299493168776285,-0.737481103314809,
1.58853871284696));
#54300=CARTESIAN_POINT('Ctrl Pts',(0.0874883317887688,-0.791151267262402,
1.60037727259743));
#54301=CARTESIAN_POINT('Ctrl Pts',(0.453392917976011,-0.654224271805385,
1.61221583234791));
#54302=CARTESIAN_POINT('Ctrl Pts',(0.710070096161475,-0.359687356501897,
1.62405439209839));
#54303=CARTESIAN_POINT('Ctrl Pts',(0.795683472888534,0.0215022524896584,
1.63589295184886));
#54304=CARTESIAN_POINT('Ctrl Pts',(0.689607831354245,0.397511729166553,
1.64773151159934));
#54305=CARTESIAN_POINT('Ctrl Pts',(0.417397976050568,0.677756199144631,
1.65957007134981));
#54306=CARTESIAN_POINT('Ctrl Pts',(0.044632295497754,0.794721645665126,
1.67140863110029));
#54307=CARTESIAN_POINT('Ctrl Pts',(-0.338885802565579,0.720229788824076,
1.68324719085077));
#54308=CARTESIAN_POINT('Ctrl Pts',(-0.640762533163177,0.472226547310077,
1.69508575060124));
#54309=CARTESIAN_POINT('Ctrl Pts',(-0.788272426813903,0.110458666545496,
1.70692431035172));
#54310=CARTESIAN_POINT('Ctrl Pts',(-0.745878705815066,-0.2779199382947,
1.71876287010219));
#54311=CARTESIAN_POINT('Ctrl Pts',(-0.523794490126561,-0.59934453197067,
1.73060142985267));
#54312=CARTESIAN_POINT('Ctrl Pts',(-0.175522342924831,-0.776380346881776,
1.74243998960314));
#54313=CARTESIAN_POINT('Ctrl Pts',(0.215035093270084,-0.766377481762356,
1.75427854935362));
#54314=CARTESIAN_POINT('Ctrl Pts',(0.553788178457126,-0.571745738323627,
1.76611710910409));
#54315=CARTESIAN_POINT('Ctrl Pts',(0.759127518266483,-0.239374073158846,
1.77795566885457));
#54316=CARTESIAN_POINT('Ctrl Pts',(0.781584576779461,0.150665474580448,
1.78979422860504));
#54317=CARTESIAN_POINT('Ctrl Pts',(0.61574919826698,0.504408029995251,1.80163278835552));
#54318=CARTESIAN_POINT('Ctrl Pts',(0.301572974012746,0.736633068247083,
1.81347134810599));
#54319=CARTESIAN_POINT('Ctrl Pts',(-0.0852555413752697,0.791394988962569,
1.82530990785647));
#54320=CARTESIAN_POINT('Ctrl Pts',(-0.451545046485497,0.655501034998605,
1.83714846760694));
#54321=CARTESIAN_POINT('Ctrl Pts',(-0.7090523164345,0.36168957470349,1.84898702735742));
#54322=CARTESIAN_POINT('Ctrl Pts',(-0.795740979406929,-0.0192569359653573,
1.86082558710789));
#54323=CARTESIAN_POINT('Ctrl Pts',(-0.690726770156282,-0.395564236095736,
1.87266414685837));
#54324=CARTESIAN_POINT('Ctrl Pts',(-0.419308782306608,-0.676575702324082,
1.88450270660884));
#54325=CARTESIAN_POINT('Ctrl Pts',(-0.0468746346789825,-0.794592539924437,
1.89634126635932));
#54326=CARTESIAN_POINT('Ctrl Pts',(0.336852134960562,-0.721183177202469,
1.90817982610979));
#54327=CARTESIAN_POINT('Ctrl Pts',(0.639427470336365,-0.474032747865934,
1.92001838586027));
#54328=CARTESIAN_POINT('Ctrl Pts',(0.787957600270134,-0.112682545536983,
1.93185694561074));
#54329=CARTESIAN_POINT('Ctrl Pts',(0.746659960802614,0.275814138316646,
1.94369550536122));
#54330=CARTESIAN_POINT('Ctrl Pts',(0.525483613561763,0.597864121279136,
1.9555340651117));
#54331=CARTESIAN_POINT('Ctrl Pts',(0.177712406238804,0.77588197373654,1.96737262486217));
#54332=CARTESIAN_POINT('Ctrl Pts',(-0.212871700931978,0.766981208183949,
1.97921118461265));
#54333=CARTESIAN_POINT('Ctrl Pts',(-0.552172642050561,0.573306123103059,
1.99104974436312));
#54334=CARTESIAN_POINT('Ctrl Pts',(-0.758449039261035,0.241515195847213,
2.0028883041136));
#54335=CARTESIAN_POINT('Ctrl Pts',(-0.782006606865756,-0.148459421721612,
2.01472686386407));
#54336=CARTESIAN_POINT('Ctrl Pts',(-0.61717006859073,-0.502668534586218,
2.02656542361455));
#54337=CARTESIAN_POINT('Ctrl Pts',(-0.303650375341446,-0.735779144874103,
2.03840398336502));
#54338=CARTESIAN_POINT('Ctrl Pts',(0.0830220668382067,-0.79163245470895,
2.0502425431155));
#54339=CARTESIAN_POINT('Ctrl Pts',(0.449693590087432,-0.656772488993135,
2.06208110286597));
#54340=CARTESIAN_POINT('Ctrl Pts',(0.708028870280121,-0.36368909075967,
2.07391966261645));
#54341=CARTESIAN_POINT('Ctrl Pts',(0.795792190877101,0.0170118177583804,
2.08575822236693));
#54342=CARTESIAN_POINT('Ctrl Pts',(0.691840128161321,0.39361289775907,2.0975967821174));
#54343=CARTESIAN_POINT('Ctrl Pts',(0.421216410066217,0.675391194495178,
2.10943534186788));
#54344=CARTESIAN_POINT('Ctrl Pts',(0.0491162836718048,0.794454384908945,
2.12127390161835));
#54345=CARTESIAN_POINT('Ctrl Pts',(-0.334815157538176,0.722136210482901,
2.13311246136883));
#54346=CARTESIAN_POINT('Ctrl Pts',(-0.638088565819885,0.475824497198633,
2.1449510211193));
#54347=CARTESIAN_POINT('Ctrl Pts',(-0.787633931880613,0.114926883787159,
2.15678958086977));
#54348=CARTESIAN_POINT('Ctrl Pts',(-0.747441446872298,-0.273751139119435,
2.16862814062026));
#54349=CARTESIAN_POINT('Ctrl Pts',(-0.600573116106444,-0.488751391274673,
2.17652051378724));
#54350=CARTESIAN_POINT('Ctrl Pts',(-0.5059592890698,-0.572385185259003,
2.18046670037073));
#54351=CARTESIAN_POINT('Ctrl Pts',(-0.345478907940185,0.713232482552819,
0.8));
#54352=CARTESIAN_POINT('Ctrl Pts',(-0.463374437871893,0.656125690688752,
0.803946186583492));
#54353=CARTESIAN_POINT('Ctrl Pts',(-0.670189208139166,0.482387406495414,
0.811838559750475));
#54354=CARTESIAN_POINT('Ctrl Pts',(-0.818976029898903,0.105327730568796,
0.82367711950095));
#54355=CARTESIAN_POINT('Ctrl Pts',(-0.77044826715263,-0.297010081933676,
0.835515679251426));
#54356=CARTESIAN_POINT('Ctrl Pts',(-0.536318264207659,-0.627841842719682,
0.847354239001901));
#54357=CARTESIAN_POINT('Ctrl Pts',(-0.172979487351029,-0.807395905129269,
0.859192798752377));
#54358=CARTESIAN_POINT('Ctrl Pts',(0.232030091481853,-0.792451210825201,
0.871031358502853));
#54359=CARTESIAN_POINT('Ctrl Pts',(0.581141987669944,-0.586590163170117,
0.882869918253326));
#54360=CARTESIAN_POINT('Ctrl Pts',(0.790249819227213,-0.239416050963522,
0.894708478003804));
#54361=CARTESIAN_POINT('Ctrl Pts',(0.808977903760532,0.165437595789089,
0.906547037754277));
#54362=CARTESIAN_POINT('Ctrl Pts',(0.632814070348998,0.530434703552899,
0.918385597504754));
#54363=CARTESIAN_POINT('Ctrl Pts',(0.304198335508654,0.767644571650904,
0.930224157255228));
#54364=CARTESIAN_POINT('Ctrl Pts',(-0.0977022007693522,0.819920106545049,
0.942062717005705));
#54365=CARTESIAN_POINT('Ctrl Pts',(-0.476065171875897,0.674667848456801,
0.953901276756179));
#54366=CARTESIAN_POINT('Ctrl Pts',(-0.739738744321667,0.366880534216174,
0.965739836506655));
#54367=CARTESIAN_POINT('Ctrl Pts',(-0.825201003181842,-0.0292923647270269,
0.97757839625713));
#54368=CARTESIAN_POINT('Ctrl Pts',(-0.711863143749104,-0.418408419461353,
0.989416956007606));
#54369=CARTESIAN_POINT('Ctrl Pts',(-0.427029516668392,-0.70672521530295,
1.00125551575808));
#54370=CARTESIAN_POINT('Ctrl Pts',(-0.039319719363844,-0.824784032088305,
1.01309407550856));
#54371=CARTESIAN_POINT('Ctrl Pts',(0.357862636905524,-0.744143179834439,
1.02493263525903));
#54372=CARTESIAN_POINT('Ctrl Pts',(0.668831894643988,-0.484229941293575,
1.03677119500951));
#54373=CARTESIAN_POINT('Ctrl Pts',(0.818672093427876,-0.107660311658766,
1.04860975475998));
#54374=CARTESIAN_POINT('Ctrl Pts',(0.771285058969472,0.294845886949012,
1.06044831451046));
#54375=CARTESIAN_POINT('Ctrl Pts',(0.538086856154138,0.626320424794314,
1.07228687426093));
#54376=CARTESIAN_POINT('Ctrl Pts',(0.175257531520918,0.806907390532518,
1.08412543401141));
#54377=CARTESIAN_POINT('Ctrl Pts',(-0.229793286081951,0.793101371161665,
1.09596399376188));
#54378=CARTESIAN_POINT('Ctrl Pts',(-0.579484339518286,0.588228390604528,
1.10780255351236));
#54379=CARTESIAN_POINT('Ctrl Pts',(-0.789571155935928,0.241644633658621,
1.11964111326283));
#54380=CARTESIAN_POINT('Ctrl Pts',(-0.809441479381897,-0.163154009200229,
1.13147967301331));
#54381=CARTESIAN_POINT('Ctrl Pts',(-0.634308327438729,-0.528647032530609,
1.14331823276378));
#54382=CARTESIAN_POINT('Ctrl Pts',(-0.306363228654176,-0.766783092791291,
1.15515679251426));
#54383=CARTESIAN_POINT('Ctrl Pts',(0.0953881870053064,-0.820192558513891,
1.16699535226474));
#54384=CARTESIAN_POINT('Ctrl Pts',(0.474159525104011,-0.676008494040558,
1.17883391201521));
#54385=CARTESIAN_POINT('Ctrl Pts',(0.738700548054304,-0.368966447751112,
1.19067247176569));
#54386=CARTESIAN_POINT('Ctrl Pts',(0.825280374535842,0.0269637287441597,
1.20251103151616));
#54387=CARTESIAN_POINT('Ctrl Pts',(0.713040959226628,0.416398042414927,
1.21434959126664));
#54388=CARTESIAN_POINT('Ctrl Pts',(0.429022028429814,0.705517425995826,
1.22618815101711));
#54389=CARTESIAN_POINT('Ctrl Pts',(0.0416469085900688,0.82466979711076,
1.23802671076759));
#54390=CARTESIAN_POINT('Ctrl Pts',(-0.355761415775427,0.745150021342865,
1.24986527051806));
#54391=CARTESIAN_POINT('Ctrl Pts',(-0.667462849337108,0.486115299097447,
1.26170383026854));
#54392=CARTESIAN_POINT('Ctrl Pts',(-0.818365042151861,0.109969982475179,
1.27354239001902));
#54393=CARTESIAN_POINT('Ctrl Pts',(-0.772113973833753,-0.292668328782704,
1.28538094976949));
#54394=CARTESIAN_POINT('Ctrl Pts',(-0.539852042310501,-0.624799577204556,
1.29721950951997));
#54395=CARTESIAN_POINT('Ctrl Pts',(-0.177533735956174,-0.806409642712222,
1.30905806927044));
#54396=CARTESIAN_POINT('Ctrl Pts',(0.227554426393989,-0.793746636081258,
1.32089662902092));
#54397=CARTESIAN_POINT('Ctrl Pts',(0.577822190831226,-0.589861216766124,
1.33273518877139));
#54398=CARTESIAN_POINT('Ctrl Pts',(0.788886148397919,-0.243871655031303,
1.34457374852187));
#54399=CARTESIAN_POINT('Ctrl Pts',(0.809898638944184,0.160869306886576,
1.35641230827234));
#54400=CARTESIAN_POINT('Ctrl Pts',(0.635797519267003,0.526855059533203,
1.36825086802281));
#54401=CARTESIAN_POINT('Ctrl Pts',(0.308525689836539,0.765915555379768,
1.38008942777329));
#54402=CARTESIAN_POINT('Ctrl Pts',(-0.0930734174729996,0.820458456121764,
1.39192798752377));
#54403=CARTESIAN_POINT('Ctrl Pts',(-0.472250101005329,0.677343768969839,
1.40376654727424));
#54404=CARTESIAN_POINT('Ctrl Pts',(-0.737656470939329,0.371049417386882,
1.41560510702472));
#54405=CARTESIAN_POINT('Ctrl Pts',(-0.825353174220117,-0.0246348750064956,
1.42744366677519));
#54406=CARTESIAN_POINT('Ctrl Pts',(-0.714213097454698,-0.414384351400939,
1.43928222652567));
#54407=CARTESIAN_POINT('Ctrl Pts',(-0.431011124036478,-0.704304018317815,
1.45112078627615));
#54408=CARTESIAN_POINT('Ctrl Pts',(-0.0439737662708354,-0.824548996204452,
1.46295934602662));
#54409=CARTESIAN_POINT('Ctrl Pts',(0.353657361973805,-0.746150929493183,
1.4747979057771));
#54410=CARTESIAN_POINT('Ctrl Pts',(0.666088489429745,-0.487996786373651,
1.48663646552757));
#54411=CARTESIAN_POINT('Ctrl Pts',(0.818051474760706,-0.11227877761912,
1.49847502527805));
#54412=CARTESIAN_POINT('Ctrl Pts',(0.772936740838731,0.290488440257801,
1.51031358502852));
#54413=CARTESIAN_POINT('Ctrl Pts',(0.541612929968569,0.62327375474399,1.522152144779));
#54414=CARTESIAN_POINT('Ctrl Pts',(0.179808526801536,0.805905473955396,
1.53399070452947));
#54415=CARTESIAN_POINT('Ctrl Pts',(-0.225313754833528,0.794385580901761,
1.54582926427995));
#54416=CARTESIAN_POINT('Ctrl Pts',(-0.576155441311798,0.591489346234249,
1.55766782403042));
#54417=CARTESIAN_POINT('Ctrl Pts',(-0.788194859458339,0.246096734609094,
1.5695063837809));
#54418=CARTESIAN_POINT('Ctrl Pts',(-0.810349349795935,-0.158583323672815,
1.58134494353137));
#54419=CARTESIAN_POINT('Ctrl Pts',(-0.63728164864173,-0.525058891521977,
1.59318350328185));
#54420=CARTESIAN_POINT('Ctrl Pts',(-0.310685694423989,-0.765041919467224,
1.60502206303233));
#54421=CARTESIAN_POINT('Ctrl Pts',(0.0907579068559442,-0.820717820937828,
1.6168606227828));
#54422=CARTESIAN_POINT('Ctrl Pts',(0.470336916677778,-0.678673650639136,
1.62869918253328));
#54423=CARTESIAN_POINT('Ctrl Pts',(0.736606520332441,-0.373129432590817,
1.64053774228375));
#54424=CARTESIAN_POINT('Ctrl Pts',(0.825419402139098,0.022305825116897,
1.65237630203423));
#54425=CARTESIAN_POINT('Ctrl Pts',(0.715379548855604,0.412367360906464,
1.6642148617847));
#54426=CARTESIAN_POINT('Ctrl Pts',(0.432996787774168,0.703085002712376,
1.67605342153518));
#54427=CARTESIAN_POINT('Ctrl Pts',(0.0463002738163106,0.824421629936008,
1.68789198128565));
#54428=CARTESIAN_POINT('Ctrl Pts',(-0.351550492222292,0.747145896515582,
1.69973054103613));
#54429=CARTESIAN_POINT('Ctrl Pts',(-0.664708825881036,0.489874388040104,
1.7115691007866));
#54430=CARTESIAN_POINT('Ctrl Pts',(-0.817731393743069,0.114586678758172,
1.72340766053708));
#54431=CARTESIAN_POINT('Ctrl Pts',(-0.773753353437319,-0.288306238757181,
1.73524622028755));
#54432=CARTESIAN_POINT('Ctrl Pts',(-0.543369505105439,-0.621742969548736,
1.74708478003803));
#54433=CARTESIAN_POINT('Ctrl Pts',(-0.182081885945323,-0.805394888283011,
1.7589233397885));
#54434=CARTESIAN_POINT('Ctrl Pts',(0.223071289242151,-0.795018200532323,
1.77076189953898));
#54435=CARTESIAN_POINT('Ctrl Pts',(0.574484104230999,-0.593112766046828,
1.78260045928945));
#54436=CARTESIAN_POINT('Ctrl Pts',(0.787497294621621,-0.248319854674241,
1.79443901903993));
#54437=CARTESIAN_POINT('Ctrl Pts',(0.810793608348351,0.156296077760331,
1.80627757879041));
#54438=CARTESIAN_POINT('Ctrl Pts',(0.638760703745772,0.523258542798921,
1.81811613854088));
#54439=CARTESIAN_POINT('Ctrl Pts',(0.312843225217752,0.764162192009703,
1.82995469829136));
#54440=CARTESIAN_POINT('Ctrl Pts',(-0.0884416735910731,0.820970650897095,
1.84179325804183));
#54441=CARTESIAN_POINT('Ctrl Pts',(-0.468419987354874,0.679998128459186,
1.85363181779231));
#54442=CARTESIAN_POINT('Ctrl Pts',(-0.735550704593678,0.375206476801514,
1.86547037754278));
#54443=CARTESIAN_POINT('Ctrl Pts',(-0.82547905776555,-0.0199765976209763,
1.87730893729326));
#54444=CARTESIAN_POINT('Ctrl Pts',(-0.71654030414144,-0.410347086989817,
1.88914749704373));
#54445=CARTESIAN_POINT('Ctrl Pts',(-0.434979003832696,-0.701860388889109,
1.90098605679421));
#54446=CARTESIAN_POINT('Ctrl Pts',(-0.0486264127012158,-0.824287699312935,
1.91282461654468));
#54447=CARTESIAN_POINT('Ctrl Pts',(0.349440823295038,-0.748134914500893,
1.92466317629516));
#54448=CARTESIAN_POINT('Ctrl Pts',(0.66332386967939,-0.491748089120693,
1.93650173604564));
#54449=CARTESIAN_POINT('Ctrl Pts',(0.817404801641573,-0.116893667567328,
1.94834029579611));
#54450=CARTESIAN_POINT('Ctrl Pts',(0.774563805139175,0.286121741757891,
1.96017885554659));
#54451=CARTESIAN_POINT('Ctrl Pts',(0.545121753711234,0.620207233606538,
1.97201741529706));
#54452=CARTESIAN_POINT('Ctrl Pts',(0.184353795332487,0.804877890158005,
1.98385597504754));
#54453=CARTESIAN_POINT('Ctrl Pts',(-0.220827047566715,0.795644489149525,
1.99569453479801));
#54454=CARTESIAN_POINT('Ctrl Pts',(-0.572808192715582,0.594731464833006,
2.00753309454849));
#54455=CARTESIAN_POINT('Ctrl Pts',(-0.786793459800209,0.250540994448481,
2.01937165429896));
#54456=CARTESIAN_POINT('Ctrl Pts',(-0.811231410355536,-0.154007581274137,
2.03121021404944));
#54457=CARTESIAN_POINT('Ctrl Pts',(-0.64023467420401,-0.521454039740266,
2.04304877379992));
#54458=CARTESIAN_POINT('Ctrl Pts',(-0.314998262265981,-0.763276356191801,
2.05488733355038));
#54459=CARTESIAN_POINT('Ctrl Pts',(0.0861247306358769,-0.821216991107851,
2.06672589330087));
#54460=CARTESIAN_POINT('Ctrl Pts',(0.466499339150846,-0.681317098667531,
2.07856445305134));
#54461=CARTESIAN_POINT('Ctrl Pts',(0.734489010664305,-0.37728071788342,
2.09040301280181));
#54462=CARTESIAN_POINT('Ctrl Pts',(0.825532183088033,0.0176475758538063,
2.10224157255229));
#54463=CARTESIAN_POINT('Ctrl Pts',(0.717695270067213,0.408322824103754,
2.11408013230276));
#54464=CARTESIAN_POINT('Ctrl Pts',(0.436957922609435,0.700631614159863,
2.12591869205324));
#54465=CARTESIAN_POINT('Ctrl Pts',(0.0509518356043011,0.824144381229582,
2.13775725180371));
#54466=CARTESIAN_POINT('Ctrl Pts',(-0.34732772085739,0.749123564117677,
2.14959581155419));
#54467=CARTESIAN_POINT('Ctrl Pts',(-0.661934928218153,0.493606798913433,
2.16143437130467));
#54468=CARTESIAN_POINT('Ctrl Pts',(-0.817069037260797,0.119221880229497,
2.17327293105514));
#54469=CARTESIAN_POINT('Ctrl Pts',(-0.775374496559064,-0.283981645071211,
2.18511149080562));
#54470=CARTESIAN_POINT('Ctrl Pts',(-0.623017467785008,-0.507016791131852,
2.1930038639726));
#54471=CARTESIAN_POINT('Ctrl Pts',(-0.524867774838428,-0.593776110108985,
2.19695005055609));
#54472=CARTESIAN_POINT('Ctrl Pts',(-0.792449256123249,-1.33074723724148E-5,
2.02673131746348));
#54473=CARTESIAN_POINT('Ctrl Pts',(-0.792479308861568,-0.049582192157152,
2.02822428299213));
#54474=CARTESIAN_POINT('Ctrl Pts',(-0.787900256251548,-0.099145593031894,
2.02971724852078));
#54475=CARTESIAN_POINT('Ctrl Pts',(-0.778658962571061,-0.14782389506472,
2.03121021404944));
#54476=CARTESIAN_POINT('Ctrl Pts',(-0.754232498305028,-0.276489734096178,
2.03515640063293));
#54477=CARTESIAN_POINT('Ctrl Pts',(-0.697233586254521,-0.398971886918219,
2.03910258721642));
#54478=CARTESIAN_POINT('Ctrl Pts',(-0.61452806157293,-0.50051668273783,
2.04304877379991));
#54479=CARTESIAN_POINT('Ctrl Pts',(-0.531822536891337,-0.602061478557442,
2.04699496038341));
#54480=CARTESIAN_POINT('Ctrl Pts',(-0.423410399578662,-0.682668917374621,
2.0509411469669));
#54481=CARTESIAN_POINT('Ctrl Pts',(-0.302350498772013,-0.732629409269219,
2.05488733355039));
#54482=CARTESIAN_POINT('Ctrl Pts',(-0.181290597965366,-0.782589901163817,
2.05883352013388));
#54483=CARTESIAN_POINT('Ctrl Pts',(-0.0475829336647421,-0.801903446135835,
2.06277970671737));
#54484=CARTESIAN_POINT('Ctrl Pts',(0.0826666665713958,-0.78824356988179,
2.06672589330087));
#54485=CARTESIAN_POINT('Ctrl Pts',(0.212916266807534,-0.774583693627745,
2.07067207988436));
#54486=CARTESIAN_POINT('Ctrl Pts',(0.33970780297919,-0.727950396147638,
2.07461826646785));
#54487=CARTESIAN_POINT('Ctrl Pts',(0.447768516317261,-0.653961017276899,
2.07856445305134));
#54488=CARTESIAN_POINT('Ctrl Pts',(0.555829229655333,-0.57997163840616,
2.08251063963483));
#54489=CARTESIAN_POINT('Ctrl Pts',(0.645159120159819,-0.47862617814479,
2.08645682621832));
#54490=CARTESIAN_POINT('Ctrl Pts',(0.704997927482683,-0.362132065724567,
2.09040301280181));
#54491=CARTESIAN_POINT('Ctrl Pts',(0.764836734805548,-0.245637953304344,
2.09434919938531));
#54492=CARTESIAN_POINT('Ctrl Pts',(0.79518445894679,-0.113995188725269,
2.0982953859688));
#54493=CARTESIAN_POINT('Ctrl Pts',(0.792385502180608,0.01693873493926,2.10224157255229));
#54494=CARTESIAN_POINT('Ctrl Pts',(0.789586545414427,0.147872658603789,
2.10618775913578));
#54495=CARTESIAN_POINT('Ctrl Pts',(0.75364090774082,0.278097741353771,2.11013394571927));
#54496=CARTESIAN_POINT('Ctrl Pts',(0.688878530994387,0.391928414404781,
2.11408013230276));
#54497=CARTESIAN_POINT('Ctrl Pts',(0.624116154247955,0.50575908745579,2.11802631888626));
#54498=CARTESIAN_POINT('Ctrl Pts',(0.530537038428692,0.603195350807828,
2.12197250546975));
#54499=CARTESIAN_POINT('Ctrl Pts',(0.419413132684874,0.672498943662132,
2.12591869205324));
#54500=CARTESIAN_POINT('Ctrl Pts',(0.308289226941054,0.741802536516437,
2.12986487863673));
#54501=CARTESIAN_POINT('Ctrl Pts',(0.179620531272676,0.782973458873009,
2.13381106522022));
#54502=CARTESIAN_POINT('Ctrl Pts',(0.0489062573615377,0.791055450532645,
2.13775725180372));
#54503=CARTESIAN_POINT('Ctrl Pts',(-0.0586673228051905,0.797706665826054,
2.14100483453581));
#54504=CARTESIAN_POINT('Ctrl Pts',(-0.167626322520823,0.7819475667733,2.1442524172679));
#54505=CARTESIAN_POINT('Ctrl Pts',(-0.26905776807643,0.745453775914814,
2.1475));
#54506=CARTESIAN_POINT('',(-0.410244091002541,-0.575644225023336,0.8));
#54507=CARTESIAN_POINT('Ctrl Pts',(-0.410244091002539,-0.575644225023337,
0.8));
#54508=CARTESIAN_POINT('Ctrl Pts',(-0.427865382519306,-0.564603183918701,
0.8));
#54509=CARTESIAN_POINT('Ctrl Pts',(-0.444970629642914,-0.552798572830416,
0.8));
#54510=CARTESIAN_POINT('Ctrl Pts',(-0.461505849283383,-0.540259693735842,
0.8));
#54511=CARTESIAN_POINT('Ctrl Pts',(-0.485257387055636,-0.522248583698476,
0.8));
#54512=CARTESIAN_POINT('Ctrl Pts',(-0.507833747975836,-0.502723524946606,
0.8));
#54513=CARTESIAN_POINT('Ctrl Pts',(-0.529139522554897,-0.481836862385063,
0.8));
#54514=CARTESIAN_POINT('Ctrl Pts',(-0.536263390677962,-0.474853129920079,
0.8));
#54515=CARTESIAN_POINT('Ctrl Pts',(-0.543245068841058,-0.467716959459887,
0.8));
#54516=CARTESIAN_POINT('Ctrl Pts',(-0.55008052571286,-0.460433451983989,
0.8));
#54517=CARTESIAN_POINT('Ctrl Pts',(-0.556729564362481,-0.453348582074,0.8));
#54518=CARTESIAN_POINT('Ctrl Pts',(-0.563234833433516,-0.446129922658457,
0.8));
#54519=CARTESIAN_POINT('Ctrl Pts',(-0.569588353878728,-0.438788486260154,
0.8));
#54520=CARTESIAN_POINT('Ctrl Pts',(-0.592447670772818,-0.412374748784406,
0.8));
#54521=CARTESIAN_POINT('Ctrl Pts',(-0.613365866820692,-0.384353037236454,
0.8));
#54522=CARTESIAN_POINT('Ctrl Pts',(-0.632187162640585,-0.354957378738931,
0.8));
#54523=CARTESIAN_POINT('Ctrl Pts',(-0.641845472764862,-0.339872743292293,
0.8));
#54524=CARTESIAN_POINT('Ctrl Pts',(-0.650951053702501,-0.324425624633106,
0.8));
#54525=CARTESIAN_POINT('Ctrl Pts',(-0.659478734205941,-0.308644066268824,
0.8));
#54526=CARTESIAN_POINT('Ctrl Pts',(-0.663690016950242,-0.300850551444848,
0.8));
#54527=CARTESIAN_POINT('Ctrl Pts',(-0.667756705771111,-0.292981910079593,
0.8));
#54528=CARTESIAN_POINT('Ctrl Pts',(-0.671672822458712,-0.285049256379356,
0.8));
#54529=CARTESIAN_POINT('Ctrl Pts',(-0.675279999292623,-0.277742404479482,
0.8));
#54530=CARTESIAN_POINT('Ctrl Pts',(-0.678760443753924,-0.270379362225497,
0.8));
#54531=CARTESIAN_POINT('Ctrl Pts',(-0.682112403616848,-0.262963134400256,
0.8));
#54532=CARTESIAN_POINT('Ctrl Pts',(-0.696491101098182,-0.231150194892449,
0.8));
#54533=CARTESIAN_POINT('Ctrl Pts',(-0.708509103401211,-0.198361084298674,
0.8));
#54534=CARTESIAN_POINT('Ctrl Pts',(-0.71816700906694,-0.164874557004865,
0.8));
#54535=CARTESIAN_POINT('Ctrl Pts',(-0.725096186175765,-0.140849257275371,
0.8));
#54536=CARTESIAN_POINT('Ctrl Pts',(-0.730809623242255,-0.116464099854586,
0.8));
#54537=CARTESIAN_POINT('Ctrl Pts',(-0.73529274404788,-0.0918147743273888,
0.8));
#54538=CARTESIAN_POINT('Ctrl Pts',(-0.737389184126333,-0.0802880195994795,
0.8));
#54539=CARTESIAN_POINT('Ctrl Pts',(-0.739216399251251,-0.0687034374573978,
0.8));
#54540=CARTESIAN_POINT('Ctrl Pts',(-0.74077190957322,-0.0570706015003154,
0.8));
#54541=CARTESIAN_POINT('Ctrl Pts',(-0.741799324663645,-0.0493871094411838,
0.8));
#54542=CARTESIAN_POINT('Ctrl Pts',(-0.7427081925385,-0.0416825640362764,
0.8));
#54543=CARTESIAN_POINT('Ctrl Pts',(-0.743497641662436,-0.0339597144281698,
0.8));
#54544=CARTESIAN_POINT('Ctrl Pts',(-0.744231464389403,-0.0267810345265218,
0.8));
#54545=CARTESIAN_POINT('Ctrl Pts',(-0.744861106235136,-0.0195961998053866,
0.8));
#54546=CARTESIAN_POINT('Ctrl Pts',(-0.745386565611995,-0.0124084559110833,
0.8));
#54547=CARTESIAN_POINT('Ctrl Pts',(-0.748026655936726,0.0237052646687871,
0.8));
#54548=CARTESIAN_POINT('Ctrl Pts',(-0.74804166046495,0.0598982256610108,
0.8));
#54549=CARTESIAN_POINT('Ctrl Pts',(-0.74541198023048,0.0958822642309481,
0.8));
#54550=CARTESIAN_POINT('Ctrl Pts',(-0.743118296207274,0.127268595267087,
0.8));
#54551=CARTESIAN_POINT('Ctrl Pts',(-0.738811956202042,0.158496935357709,
0.8));
#54552=CARTESIAN_POINT('Ctrl Pts',(-0.732567679777806,0.189394981218774,
0.8));
#54553=CARTESIAN_POINT('Ctrl Pts',(-0.728871602747368,0.207683978987875,
0.8));
#54554=CARTESIAN_POINT('Ctrl Pts',(-0.724495919547074,0.225857276064614,
0.8));
#54555=CARTESIAN_POINT('Ctrl Pts',(-0.719450927062176,0.243878325627313,
0.8));
#54556=CARTESIAN_POINT('Ctrl Pts',(-0.716942162599312,0.25283979957633,
0.8));
#54557=CARTESIAN_POINT('Ctrl Pts',(-0.7142667112202,0.261766480726714,0.8));
#54558=CARTESIAN_POINT('Ctrl Pts',(-0.711433641154155,0.270630156805554,
0.8));
#54559=CARTESIAN_POINT('Ctrl Pts',(-0.700362437871719,0.305268043412969,
0.8));
#54560=CARTESIAN_POINT('Ctrl Pts',(-0.686869620567715,0.339017637772264,
0.8));
#54561=CARTESIAN_POINT('Ctrl Pts',(-0.671084494453807,0.371624233448503,
0.8));
#54562=CARTESIAN_POINT('Ctrl Pts',(-0.657862557602499,0.398936169118597,
0.8));
#54563=CARTESIAN_POINT('Ctrl Pts',(-0.643031245141321,0.425446637465682,
0.8));
#54564=CARTESIAN_POINT('Ctrl Pts',(-0.626639134868092,0.450999679702338,
0.8));
#54565=CARTESIAN_POINT('Ctrl Pts',(-0.617718019074226,0.464906470522983,
0.8));
#54566=CARTESIAN_POINT('Ctrl Pts',(-0.608334186215446,0.478529525381889,
0.8));
#54567=CARTESIAN_POINT('Ctrl Pts',(-0.598506201793284,0.491852341465841,
0.8));
#54568=CARTESIAN_POINT('Ctrl Pts',(-0.59296152296404,0.49936870831315,0.8));
#54569=CARTESIAN_POINT('Ctrl Pts',(-0.58727544055949,0.506789488860121,
0.8));
#54570=CARTESIAN_POINT('Ctrl Pts',(-0.581451041194421,0.514111518781399,
0.8));
#54571=CARTESIAN_POINT('Ctrl Pts',(-0.576846734062576,0.519899733577986,
0.8));
#54572=CARTESIAN_POINT('Ctrl Pts',(-0.572157004628658,0.525624771374302,
0.8));
#54573=CARTESIAN_POINT('Ctrl Pts',(-0.56739138065304,0.531276185837925,
0.8));
#54574=CARTESIAN_POINT('Ctrl Pts',(-0.543777984951897,0.55927862301791,
0.8));
#54575=CARTESIAN_POINT('Ctrl Pts',(-0.518255565866718,0.585538394849063,
0.8));
#54576=CARTESIAN_POINT('Ctrl Pts',(-0.491061458562882,0.609904318648996,
0.8));
#54577=CARTESIAN_POINT('Ctrl Pts',(-0.463733518954985,0.634390156211358,
0.8));
#54578=CARTESIAN_POINT('Ctrl Pts',(-0.434716576426148,0.656964357819938,
0.8));
#54579=CARTESIAN_POINT('Ctrl Pts',(-0.404209754469363,0.677442878107525,
0.8));
#54580=CARTESIAN_POINT('Ctrl Pts',(-0.385198137815666,0.690204934341835,
0.8));
#54581=CARTESIAN_POINT('Ctrl Pts',(-0.365607118174303,0.702152441062861,
0.8));
#54582=CARTESIAN_POINT('Ctrl Pts',(-0.345478907940185,0.713232482552819,
0.8));
#54583=CARTESIAN_POINT('Ctrl Pts',(-0.410244091002541,-0.575644225023336,
0.8));
#54584=CARTESIAN_POINT('Ctrl Pts',(-0.331890193452863,-0.631365139834126,
0.803247582732095));
#54585=CARTESIAN_POINT('Ctrl Pts',(-0.132967640534065,-0.719349431943114,
0.810441352047681));
#54586=CARTESIAN_POINT('Ctrl Pts',(0.206953274654826,-0.706806483749897,
0.821581307946761));
#54587=CARTESIAN_POINT('Ctrl Pts',(0.518334654870034,-0.523194014936019,
0.833419867697235));
#54588=CARTESIAN_POINT('Ctrl Pts',(0.704843009111363,-0.213540991323109,
0.845258427447713));
#54589=CARTESIAN_POINT('Ctrl Pts',(0.72154704261594,0.147557810200025,0.857096987198186));
#54590=CARTESIAN_POINT('Ctrl Pts',(0.564422240537776,0.473107596474913,
0.868935546948663));
#54591=CARTESIAN_POINT('Ctrl Pts',(0.271321884484909,0.684680839711599,
0.880774106699136));
#54592=CARTESIAN_POINT('Ctrl Pts',(-0.0871429660742197,0.731306659067973,
0.892612666449614));
#54593=CARTESIAN_POINT('Ctrl Pts',(-0.424614090524265,0.601752641869639,
0.904451226200088));
#54594=CARTESIAN_POINT('Ctrl Pts',(-0.654181788655658,0.333777263871536,
0.91600742635268));
#54595=CARTESIAN_POINT('Ctrl Pts',(-0.706836463769599,0.10844725711356,
0.92361743992178));
#54596=CARTESIAN_POINT('Ctrl Pts',(-0.70690109581483,-8.28105672094105E-6,
0.927281266907388));
#54597=CARTESIAN_POINT('Origin',(0.,0.,0.522718733092613));
#54598=CARTESIAN_POINT('',(0.410219162127156,-0.575636310115765,0.8));
#54599=CARTESIAN_POINT('Origin',(0.,0.,0.8));
#54600=CARTESIAN_POINT('Ctrl Pts',(0.410219162127157,-0.575636310115765,
0.8));
#54601=CARTESIAN_POINT('Ctrl Pts',(0.50537039190027,-0.507828117569598,
0.803946186583492));
#54602=CARTESIAN_POINT('Ctrl Pts',(0.661310874189135,-0.324192005087297,
0.811838559750475));
#54603=CARTESIAN_POINT('Ctrl Pts',(0.735886669498874,0.0295778738072663,
0.82367711950095));
#54604=CARTESIAN_POINT('Ctrl Pts',(0.633181296569113,0.376134898320248,
0.835515679251426));
#54605=CARTESIAN_POINT('Ctrl Pts',(0.377934853131171,0.632119386061258,
0.847354239001902));
#54606=CARTESIAN_POINT('Ctrl Pts',(0.0316399747779213,0.735797878194255,
0.859192798752376));
#54607=CARTESIAN_POINT('Ctrl Pts',(-0.322277466664887,0.662225266491492,
0.871031358502852));
#54608=CARTESIAN_POINT('Ctrl Pts',(-0.598554603122584,0.429109740989168,
0.882869918253328));
#54609=CARTESIAN_POINT('Ctrl Pts',(-0.697801857104019,0.176262631310262,
0.891765709783247));
#54610=CARTESIAN_POINT('Ctrl Pts',(-0.70687082927169,0.0297279928167443,
0.896715314729675));
#54611=CARTESIAN_POINT('Ctrl Pts',(-0.706841592163942,1.7867609379222E-5,
0.897718733092612));
#54612=CARTESIAN_POINT('Ctrl Pts',(0.459925989935304,-0.645386964372562,
0.750549949443908));
#54613=CARTESIAN_POINT('Ctrl Pts',(0.56660682688118,-0.569362358596461,
0.7544961360274));
#54614=CARTESIAN_POINT('Ctrl Pts',(0.741442834823356,-0.363474802336684,
0.762388509194383));
#54615=CARTESIAN_POINT('Ctrl Pts',(0.825055083225377,0.0331618660143685,
0.77422706894486));
#54616=CARTESIAN_POINT('Ctrl Pts',(0.709904757064473,0.421711688362163,
0.786065628695334));
#54617=CARTESIAN_POINT('Ctrl Pts',(0.423729746207052,0.708714173379848,
0.79790418844581));
#54618=CARTESIAN_POINT('Ctrl Pts',(0.0354738346346534,0.824955532954583,
0.809742748196284));
#54619=CARTESIAN_POINT('Ctrl Pts',(-0.361328276624348,0.742468025315849,
0.821581307946761));
#54620=CARTESIAN_POINT('Ctrl Pts',(-0.671082298896012,0.481105566575535,
0.833419867697235));
#54621=CARTESIAN_POINT('Ctrl Pts',(-0.819165154783747,0.103842512917493,
0.845258427447712));
#54622=CARTESIAN_POINT('Ctrl Pts',(-0.769901973202423,-0.298438927106654,
0.857096987198186));
#54623=CARTESIAN_POINT('Ctrl Pts',(-0.535160834284934,-0.628822310037111,
0.868935546948663));
#54624=CARTESIAN_POINT('Ctrl Pts',(-0.171493479654568,-0.807715789857204,
0.880774106699136));
#54625=CARTESIAN_POINT('Ctrl Pts',(0.233488563272111,-0.792021329318452,
0.892612666449614));
#54626=CARTESIAN_POINT('Ctrl Pts',(0.582220609890365,-0.585520204307218,
0.904451226200087));
#54627=CARTESIAN_POINT('Ctrl Pts',(0.790689220785267,-0.237960683284075,
0.916289785950564));
#54628=CARTESIAN_POINT('Ctrl Pts',(0.808671984762012,0.166926192695345,
0.928128345701038));
#54629=CARTESIAN_POINT('Ctrl Pts',(0.631836653009791,0.531598701367769,
0.939966905451514));
#54630=CARTESIAN_POINT('Ctrl Pts',(0.302784828425095,0.7682031503306,0.951805465201989));
#54631=CARTESIAN_POINT('Ctrl Pts',(-0.0992112365740696,0.819738900460409,
0.963644024952465));
#54632=CARTESIAN_POINT('Ctrl Pts',(-0.47730620873286,0.673790409958764,
0.97548258470294));
#54633=CARTESIAN_POINT('Ctrl Pts',(-0.740412794591558,0.365518299690486,
0.987321144453415));
#54634=CARTESIAN_POINT('Ctrl Pts',(-0.825145684698249,-0.0308112439180193,
0.999159704203891));
#54635=CARTESIAN_POINT('Ctrl Pts',(-0.71109178130035,-0.419718015185374,
1.01099826395437));
#54636=CARTESIAN_POINT('Ctrl Pts',(-0.425727941103712,-0.70751003802647,
1.02283682370484));
#54637=CARTESIAN_POINT('Ctrl Pts',(-0.0378014942215861,-0.824855005894519,
1.03467538345532));
#54638=CARTESIAN_POINT('Ctrl Pts',(0.359231753999693,-0.74348320804793,
1.04651394320579));
#54639=CARTESIAN_POINT('Ctrl Pts',(0.66972206825419,-0.482998017612323,
1.05835250295627));
#54640=CARTESIAN_POINT('Ctrl Pts',(0.818868870740767,-0.106153220665947,
1.07019106270674));
#54641=CARTESIAN_POINT('Ctrl Pts',(0.770741034171086,0.296265070453716,
1.08202962245722));
#54642=CARTESIAN_POINT('Ctrl Pts',(0.536933090865458,0.627309803573318,
1.09386818220769));
#54643=CARTESIAN_POINT('Ctrl Pts',(0.173771980669987,0.807228612265459,
1.10570674195817));
#54644=CARTESIAN_POINT('Ctrl Pts',(-0.231252736739835,0.792677049923898,
1.11754530170865));
#54645=CARTESIAN_POINT('Ctrl Pts',(-0.580566092048616,0.587160750126607,
1.12938386145912));
#54646=CARTESIAN_POINT('Ctrl Pts',(-0.790014604096767,0.240190880425609,
1.14122242120959));
#54647=CARTESIAN_POINT('Ctrl Pts',(-0.809139791567519,-0.164643649825546,
1.15306098096007));
#54648=CARTESIAN_POINT('Ctrl Pts',(-0.633334183606886,-0.529813689518128,
1.16489954071054));
#54649=CARTESIAN_POINT('Ctrl Pts',(-0.304951310912786,-0.767345705466825,
1.17673810046102));
#54650=CARTESIAN_POINT('Ctrl Pts',(0.0968977319333379,-0.820015587212819,
1.1885766602115));
#54651=CARTESIAN_POINT('Ctrl Pts',(0.475403031018361,-0.675134573121806,
1.20041521996197));
#54652=CARTESIAN_POINT('Ctrl Pts',(0.739378440518577,-0.3676061145059,1.21225377971245));
#54653=CARTESIAN_POINT('Ctrl Pts',(0.825229341698803,0.0284827548732166,
1.22409233946292));
#54654=CARTESIAN_POINT('Ctrl Pts',(0.712273295467589,0.41770981110042,1.2359308992134));
#54655=CARTESIAN_POINT('Ctrl Pts',(0.427722672505628,0.706305917538889,
1.24776945896387));
#54656=CARTESIAN_POINT('Ctrl Pts',(0.0401288898270517,0.824745055109187,
1.25960801871435));
#54657=CARTESIAN_POINT('Ctrl Pts',(-0.357132389735606,0.744493915305923,
1.27144657846482));
#54658=CARTESIAN_POINT('Ctrl Pts',(-0.668356495584918,0.484885892283179,
1.2832851382153));
#54659=CARTESIAN_POINT('Ctrl Pts',(-0.818566071344556,0.108463452689587,
1.29512369796577));
#54660=CARTESIAN_POINT('Ctrl Pts',(-0.771573955797898,-0.294089041720683,
1.30696225771625));
#54661=CARTESIAN_POINT('Ctrl Pts',(-0.538701073410628,-0.625792207711191,
1.31880081746672));
#54662=CARTESIAN_POINT('Ctrl Pts',(-0.176049097430337,-0.806735055033417,
1.3306393772172));
#54663=CARTESIAN_POINT('Ctrl Pts',(0.229015068575353,-0.793326434761401,
1.34247793696768));
#54664=CARTESIAN_POINT('Ctrl Pts',(0.578906951684556,-0.588796632987233,
1.35431649671815));
#54665=CARTESIAN_POINT('Ctrl Pts',(0.7893336969416,-0.242419158892843,1.36615505646863));
#54666=CARTESIAN_POINT('Ctrl Pts',(0.809601155745132,0.162359792873586,
1.3779936162191));
#54667=CARTESIAN_POINT('Ctrl Pts',(0.634826671343973,0.528024460679748,
1.38983217596958));
#54668=CARTESIAN_POINT('Ctrl Pts',(0.307115365276427,0.766482149914096,
1.40167073572005));
#54669=CARTESIAN_POINT('Ctrl Pts',(-0.0945834557624904,0.820285745104614,
1.41350929547053));
#54670=CARTESIAN_POINT('Ctrl Pts',(-0.473496067967565,0.676473360410492,
1.425347855221));
#54671=CARTESIAN_POINT('Ctrl Pts',(-0.738338199244068,0.369691002409899,
1.43718641497148));
#54672=CARTESIAN_POINT('Ctrl Pts',(-0.825306427919384,-0.0261540390906397,
1.44902497472195));
#54673=CARTESIAN_POINT('Ctrl Pts',(-0.713449138253425,-0.415698281029946,
1.46086353447243));
#54674=CARTESIAN_POINT('Ctrl Pts',(-0.429713998222261,-0.705096173197421,
1.4727020942229));
#54675=CARTESIAN_POINT('Ctrl Pts',(-0.0424559659116393,-0.824628537393848,
1.48454065397338));
#54676=CARTESIAN_POINT('Ctrl Pts',(0.355030181852222,-0.745498694633187,
1.49637921372386));
#54677=CARTESIAN_POINT('Ctrl Pts',(0.666985601215579,-0.486769906112632,
1.50821777347433));
#54678=CARTESIAN_POINT('Ctrl Pts',(0.818256754224468,-0.110772821088234,
1.52005633322481));
#54679=CARTESIAN_POINT('Ctrl Pts',(0.772400733869309,0.291910671343068,
1.53189489297528));
#54680=CARTESIAN_POINT('Ctrl Pts',(0.540464766619871,0.624269629061302,
1.54373345272576));
#54681=CARTESIAN_POINT('Ctrl Pts',(0.178324812423069,0.806235074280501,
1.55557201247623));
#54682=CARTESIAN_POINT('Ctrl Pts',(-0.22677557690873,0.793969502842219,
1.56741057222671));
#54683=CARTESIAN_POINT('Ctrl Pts',(-0.577243201850593,0.590427827632711,
1.57924913197718));
#54684=CARTESIAN_POINT('Ctrl Pts',(-0.788646504821451,0.244645507129634,
1.59108769172766));
#54685=CARTESIAN_POINT('Ctrl Pts',(-0.810056073580812,-0.160074643153275,
1.60292625147813));
#54686=CARTESIAN_POINT('Ctrl Pts',(-0.636314104357801,-0.526231027516561,
1.61476481122861));
#54687=CARTESIAN_POINT('Ctrl Pts',(-0.309276974274663,-0.765612491348801,
1.62660337097908));
#54688=CARTESIAN_POINT('Ctrl Pts',(0.0922684264834133,-0.820549371579847,
1.63844193072956));
#54689=CARTESIAN_POINT('Ctrl Pts',(0.471585334767065,-0.677806761369672,
1.65028049048004));
#54690=CARTESIAN_POINT('Ctrl Pts',(0.737292079049471,-0.371772946698273,
1.66211905023051));
#54691=CARTESIAN_POINT('Ctrl Pts',(0.82537694274688,0.0238251150599866,
1.67395760998099));
#54692=CARTESIAN_POINT('Ctrl Pts',(0.714619300295028,0.413683441016981,
1.68579616973146));
#54693=CARTESIAN_POINT('Ctrl Pts',(0.431701902398121,0.703880814621091,
1.69763472948194));
#54694=CARTESIAN_POINT('Ctrl Pts',(0.0447827039462235,0.824505453683039,
1.70947328923241));
#54695=CARTESIAN_POINT('Ctrl Pts',(-0.352925147088058,0.746497538025865,
1.72131184898289));
#54696=CARTESIAN_POINT('Ctrl Pts',(-0.665609396061764,0.4886500441012,1.73315040873336));
#54697=CARTESIAN_POINT('Ctrl Pts',(-0.817940921843388,0.113081307472958,
1.74498896848384));
#54698=CARTESIAN_POINT('Ctrl Pts',(-0.773221361802213,-0.289729976665395,
1.75682752823431));
#54699=CARTESIAN_POINT('Ctrl Pts',(-0.542224156450018,-0.622742079747232,
1.76866608798479));
#54700=CARTESIAN_POINT('Ctrl Pts',(-0.180599107528113,-0.805728673987568,
1.78050464773526));
#54701=CARTESIAN_POINT('Ctrl Pts',(0.224534279571627,-0.794606249046181,
1.79234320748574));
#54702=CARTESIAN_POINT('Ctrl Pts',(0.575574855794106,-0.592054321074615,
1.80418176723621));
#54703=CARTESIAN_POINT('Ctrl Pts',(0.787953033208021,-0.246869907409427,
1.81602032698669));
#54704=CARTESIAN_POINT('Ctrl Pts',(0.810504541452285,0.157788218860708,
1.82785888673717));
#54705=CARTESIAN_POINT('Ctrl Pts',(0.637796470804967,0.524433404306811,
1.83969744648764));
#54706=CARTESIAN_POINT('Ctrl Pts',(0.311436120695792,0.764736736698907,
1.85153600623812));
#54707=CARTESIAN_POINT('Ctrl Pts',(-0.0899526625288732,0.820806464532657,
1.86337456598859));
#54708=CARTESIAN_POINT('Ctrl Pts',(-0.469670846631493,0.679134765395703,
1.87521312573907));
#54709=CARTESIAN_POINT('Ctrl Pts',(-0.736240088263044,0.373851930767355,
1.88705168548954));
#54710=CARTESIAN_POINT('Ctrl Pts',(-0.825440885622466,-0.0214960012726903,
1.89889024524002));
#54711=CARTESIAN_POINT('Ctrl Pts',(-0.715783772269915,-0.411665307207877,
1.91072880499049));
#54712=CARTESIAN_POINT('Ctrl Pts',(-0.433686369215096,-0.702659851282511,
1.92256736474097));
#54713=CARTESIAN_POINT('Ctrl Pts',(-0.0471090853840522,-0.824375805361169,
1.93440592449144));
#54714=CARTESIAN_POINT('Ctrl Pts',(0.350817302163829,-0.747490436731311,
1.94624448424192));
#54715=CARTESIAN_POINT('Ctrl Pts',(0.664227891161086,-0.490526292859221,
1.95808304399239));
#54716=CARTESIAN_POINT('Ctrl Pts',(0.817618576558387,-0.115388890337554,
1.96992160374287));
#54717=CARTESIAN_POINT('Ctrl Pts',(0.774035833374271,0.287546968872276,
1.98176016349334));
#54718=CARTESIAN_POINT('Ctrl Pts',(0.543979228275698,0.621209584148259,
1.99359872324382));
#54719=CARTESIAN_POINT('Ctrl Pts',(0.182871965855505,0.805215834033574,
2.00543728299429));
#54720=CARTESIAN_POINT('Ctrl Pts',(-0.222291196819829,0.795236716056979,
2.01727584274477));
#54721=CARTESIAN_POINT('Ctrl Pts',(-0.573901922034738,0.593676005947508,
2.02911440249525));
#54722=CARTESIAN_POINT('Ctrl Pts',(-0.787253297042653,0.249092528689698,
2.04095296224572));
#54723=CARTESIAN_POINT('Ctrl Pts',(-0.810946537164922,-0.155500907267836,
2.0527915219962));
#54724=CARTESIAN_POINT('Ctrl Pts',(-0.63927379570346,-0.522630875674616,
2.06463008174667));
#54725=CARTESIAN_POINT('Ctrl Pts',(-0.313592714551083,-0.763856335632048,
2.07646864149715));
#54726=CARTESIAN_POINT('Ctrl Pts',(0.0876360384442657,-0.821054169383398,
2.08830720124762));
#54727=CARTESIAN_POINT('Ctrl Pts',(0.467752902891962,-0.680463003554431,
2.1001457609981));
#54728=CARTESIAN_POINT('Ctrl Pts',(0.735181678416232,-0.375916761963503,
2.11198432074857));
#54729=CARTESIAN_POINT('Ctrl Pts',(0.825499299349533,0.0191443591436184,
2.12382288049905));
#54730=CARTESIAN_POINT('Ctrl Pts',(0.716941133028235,0.409691128799217,
2.13566144024952));
#54731=CARTESIAN_POINT('Ctrl Pts',(0.529419834375704,0.604095547595317,
2.14355381341651));
#54732=CARTESIAN_POINT('Ctrl Pts',(0.418139433688274,0.673212941048261,
2.1475));
#54733=CARTESIAN_POINT('Ctrl Pts',(0.443357047332588,-0.622136746286963,
0.767033299629272));
#54734=CARTESIAN_POINT('Ctrl Pts',(0.546194681887543,-0.54885094492084,
0.770979486212764));
#54735=CARTESIAN_POINT('Ctrl Pts',(0.714732181278616,-0.350380536586888,
0.778871859379748));
#54736=CARTESIAN_POINT('Ctrl Pts',(0.795332278649875,0.0319672019453344,
0.790710419130223));
#54737=CARTESIAN_POINT('Ctrl Pts',(0.684330270232686,0.406519425014858,
0.802548978880699));
#54738=CARTESIAN_POINT('Ctrl Pts',(0.408464781848425,0.683182577606985,
0.814387538631174));
#54739=CARTESIAN_POINT('Ctrl Pts',(0.0341958813490759,0.795236314701139,
0.826226098381649));
#54740=CARTESIAN_POINT('Ctrl Pts',(-0.348311339971194,0.715720439041064,
0.838064658132124));
#54741=CARTESIAN_POINT('Ctrl Pts',(-0.64690640030487,0.463773624713412,
0.849903217882599));
#54742=CARTESIAN_POINT('Ctrl Pts',(-0.789654536273872,0.100101561821222,
0.861741777633075));
#54743=CARTESIAN_POINT('Ctrl Pts',(-0.742166072464343,-0.287687594149059,
0.873580337383551));
#54744=CARTESIAN_POINT('Ctrl Pts',(-0.515881538614479,-0.60616883754303,
0.885418897134026));
#54745=CARTESIAN_POINT('Ctrl Pts',(-0.165315386475844,-0.778617637427649,
0.8972574568845));
#54746=CARTESIAN_POINT('Ctrl Pts',(0.225077082538461,-0.763488573543004,
0.909096016634978));
#54747=CARTESIAN_POINT('Ctrl Pts',(0.561245974669709,-0.564426700417032,
0.920934576385451));
#54748=CARTESIAN_POINT('Ctrl Pts',(0.762204454534896,-0.229388093368919,
0.932773136135928));
#54749=CARTESIAN_POINT('Ctrl Pts',(0.779539385184779,0.160912637109918,
0.944611695886402));
#54750=CARTESIAN_POINT('Ctrl Pts',(0.609074588096946,0.512447732378433,
0.956450255636878));
#54751=CARTESIAN_POINT('Ctrl Pts',(0.291876933344291,0.740528450088406,
0.968288815387353));
#54752=CARTESIAN_POINT('Ctrl Pts',(-0.0956371283037994,0.790207612626788,
0.980127375137829));
#54753=CARTESIAN_POINT('Ctrl Pts',(-0.460111139635923,0.649516951025863,
0.991965934888304));
#54754=CARTESIAN_POINT('Ctrl Pts',(-0.713739248489869,0.352350416465043,
1.00380449463878));
#54755=CARTESIAN_POINT('Ctrl Pts',(-0.795419616183252,-0.0297012615661471,
1.01564305438926));
#54756=CARTESIAN_POINT('Ctrl Pts',(-0.685474531639624,-0.404597574385953,
1.02748161413973));
#54757=CARTESIAN_POINT('Ctrl Pts',(-0.410390991301174,-0.682021821514602,
1.03932017389021));
#54758=CARTESIAN_POINT('Ctrl Pts',(-0.0364396864486812,-0.795139409152199,
1.05115873364068));
#54759=CARTESIAN_POINT('Ctrl Pts',(0.346290345070115,-0.716699049575036,
1.06299729339116));
#54760=CARTESIAN_POINT('Ctrl Pts',(0.645595172293739,-0.465597899753859,
1.07483585314163));
#54761=CARTESIAN_POINT('Ctrl Pts',(0.789368925933639,-0.10232902577634,
1.08667441289211));
#54762=CARTESIAN_POINT('Ctrl Pts',(0.742974906063093,0.285592051196362,
1.09851297264258));
#54763=CARTESIAN_POINT('Ctrl Pts',(0.517589949232386,0.604710819482443,
1.11035153239306));
#54764=CARTESIAN_POINT('Ctrl Pts',(0.167511803953105,0.778148010523909,
1.12219009214353));
#54765=CARTESIAN_POINT('Ctrl Pts',(-0.222921802185991,0.7641206716585,1.13402865189401));
#54766=CARTESIAN_POINT('Ctrl Pts',(-0.559651061224657,0.566008145185137,
1.14586721164448));
#54767=CARTESIAN_POINT('Ctrl Pts',(-0.761554141072209,0.23153794713078,
1.15770577139496));
#54768=CARTESIAN_POINT('Ctrl Pts',(-0.779990339139439,-0.158712323387036,
1.16954433114543));
#54769=CARTESIAN_POINT('Ctrl Pts',(-0.610518169799975,-0.510727026002996,
1.18138289089591));
#54770=CARTESIAN_POINT('Ctrl Pts',(-0.293965367787789,-0.739701894878714,
1.19322145064639));
#54771=CARTESIAN_POINT('Ctrl Pts',(0.0934069682151096,-0.79047433167348,
1.20506001039686));
#54772=CARTESIAN_POINT('Ctrl Pts',(0.458276524348867,-0.650812690392937,
1.21689857014734));
#54773=CARTESIAN_POINT('Ctrl Pts',(0.712742157267088,-0.354363017257769,
1.22873712989781));
#54774=CARTESIAN_POINT('Ctrl Pts',(0.795500259420569,0.0274566568900879,
1.24057568964829));
#54775=CARTESIAN_POINT('Ctrl Pts',(0.68661348147945,0.402661716328286,1.25241424939876));
#54776=CARTESIAN_POINT('Ctrl Pts',(0.412313862032396,0.680861079752473,
1.26425280914924));
#54777=CARTESIAN_POINT('Ctrl Pts',(0.0386832370768144,0.795033419369922,
1.27609136889971));
#54778=CARTESIAN_POINT('Ctrl Pts',(-0.344266610900337,0.717673345864933,
1.28792992865019));
#54779=CARTESIAN_POINT('Ctrl Pts',(-0.644278794702964,0.46741776329304,
1.29976848840066));
#54780=CARTESIAN_POINT('Ctrl Pts',(-0.789077034957317,0.104556031144744,
1.31160704815114));
#54781=CARTESIAN_POINT('Ctrl Pts',(-0.743777821491236,-0.28349441441327,
1.32344560790161));
#54782=CARTESIAN_POINT('Ctrl Pts',(-0.519294239788073,-0.603247895370303,
1.33528416765209));
#54783=CARTESIAN_POINT('Ctrl Pts',(-0.169706887043414,-0.777672233807923,
1.34712272740256));
#54784=CARTESIAN_POINT('Ctrl Pts',(0.220764746546551,-0.764746662253593,
1.35896128715304));
#54785=CARTESIAN_POINT('Ctrl Pts',(0.558051691784754,-0.56758509497867,
1.37079984690351));
#54786=CARTESIAN_POINT('Ctrl Pts',(0.760897763758405,-0.233685951339037,
1.38263840665399));
#54787=CARTESIAN_POINT('Ctrl Pts',(0.780435082563398,0.156510742922116,
1.39447696640446));
#54788=CARTESIAN_POINT('Ctrl Pts',(0.611956890313221,0.509002254556838,
1.40631552615494));
#54789=CARTESIAN_POINT('Ctrl Pts',(0.296051461580979,0.738869449119083,
1.41815408590542));
#54790=CARTESIAN_POINT('Ctrl Pts',(-0.0911760643908585,0.790734757063307,
1.42999264565589));
#54791=CARTESIAN_POINT('Ctrl Pts',(-0.45643826009315,0.652103247552801,
1.44183120540637));
#54792=CARTESIAN_POINT('Ctrl Pts',(-0.711739390930608,0.356372796581756,
1.45366976515684));
#54793=CARTESIAN_POINT('Ctrl Pts',(-0.795574568591815,-0.0252118336445362,
1.46550832490732));
#54794=CARTESIAN_POINT('Ctrl Pts',(-0.687746964250731,-0.400722652104515,
1.47734688465779));
#54795=CARTESIAN_POINT('Ctrl Pts',(-0.414233449768953,-0.679694916737122,
1.48918544440827));
#54796=CARTESIAN_POINT('Ctrl Pts',(-0.0409264796948852,-0.794921099232845,
1.50102400415875));
#54797=CARTESIAN_POINT('Ctrl Pts',(0.34224013555332,-0.718641927779209,
1.51286256390922));
#54798=CARTESIAN_POINT('Ctrl Pts',(0.642957287127624,-0.469233905078542,
1.5247011236597));
#54799=CARTESIAN_POINT('Ctrl Pts',(0.788778861059663,-0.106782204000449,
1.53653968341017));
#54800=CARTESIAN_POINT('Ctrl Pts',(0.744574814687013,0.281394520343896,
1.54837824316065));
#54801=CARTESIAN_POINT('Ctrl Pts',(0.520994395532177,0.601780167976507,
1.56021680291112));
#54802=CARTESIAN_POINT('Ctrl Pts',(0.171900618865114,0.777190264979923,
1.5720553626616));
#54803=CARTESIAN_POINT('Ctrl Pts',(-0.218605933097067,0.765366563654654,
1.58389392241207));
#54804=CARTESIAN_POINT('Ctrl Pts',(-0.556447878932191,0.569157525451115,
1.59573248216255));
#54805=CARTESIAN_POINT('Ctrl Pts',(-0.760235327896969,0.235832094853859,
1.60757104191302));
#54806=CARTESIAN_POINT('Ctrl Pts',(-0.780873611876416,-0.15430791626113,
1.6194096016635));
#54807=CARTESIAN_POINT('Ctrl Pts',(-0.613390738200811,-0.507273430247668,
1.63124816141397));
#54808=CARTESIAN_POINT('Ctrl Pts',(-0.29813519810363,-0.73803112020936,
1.64308672116445));
#54809=CARTESIAN_POINT('Ctrl Pts',(0.0889444345892795,-0.790988886332396,
1.65492528091492));
#54810=CARTESIAN_POINT('Ctrl Pts',(0.454596361508265,-0.653388612426953,
1.6667638406654));
#54811=CARTESIAN_POINT('Ctrl Pts',(0.710730957463525,-0.358379738334567,
1.67860240041587));
#54812=CARTESIAN_POINT('Ctrl Pts',(0.795642543105968,0.0229668096530947,
1.69044096016635));
#54813=CARTESIAN_POINT('Ctrl Pts',(0.688874970927933,0.398780397179714,
1.70227951991682));
#54814=CARTESIAN_POINT('Ctrl Pts',(0.416149739226554,0.678523341741051,
1.7141180796673));
#54815=CARTESIAN_POINT('Ctrl Pts',(0.0431693964412828,0.79480244964184,
1.72595663941777));
#54816=CARTESIAN_POINT('Ctrl Pts',(-0.340210935164571,0.719604787602345,
1.73779519916825));
#54817=CARTESIAN_POINT('Ctrl Pts',(-0.641630660090076,0.471046310651245,
1.74963375891873));
#54818=CARTESIAN_POINT('Ctrl Pts',(-0.788474406614834,0.109007526616991,
1.7614723186692));
#54819=CARTESIAN_POINT('Ctrl Pts',(-0.745365879304481,-0.279292385707923,
1.77331087841968));
#54820=CARTESIAN_POINT('Ctrl Pts',(-0.522690402927433,-0.600307648987884,
1.78514943817015));
#54821=CARTESIAN_POINT('Ctrl Pts',(-0.174092981950916,-0.776702107877354,
1.79698799792063));
#54822=CARTESIAN_POINT('Ctrl Pts',(0.216445379026807,-0.765980370925967,
1.8088265576711));
#54823=CARTESIAN_POINT('Ctrl Pts',(0.554839635437107,-0.570725424081958,
1.82066511742158));
#54824=CARTESIAN_POINT('Ctrl Pts',(0.759566838762484,-0.237976360587295,
1.83250367717205));
#54825=CARTESIAN_POINT('Ctrl Pts',(0.781305923586716,0.152103860944654,
1.84434223692253));
#54826=CARTESIAN_POINT('Ctrl Pts',(0.614819702046,0.505540566839355,1.856180796673));
#54827=CARTESIAN_POINT('Ctrl Pts',(0.300216560764099,0.737186914827925,
1.86801935642348));
#54828=CARTESIAN_POINT('Ctrl Pts',(-0.086712096579095,0.791236717450754,
1.87985791617396));
#54829=CARTESIAN_POINT('Ctrl Pts',(-0.452750843260733,0.654668774793751,
1.89169647592443));
#54830=CARTESIAN_POINT('Ctrl Pts',(-0.709716864894072,0.360383826510688,
1.90353503567491));
#54831=CARTESIAN_POINT('Ctrl Pts',(-0.795704182424333,-0.0207216027410379,
1.91537359542538));
#54832=CARTESIAN_POINT('Ctrl Pts',(-0.689997492524418,-0.396834967118559,
1.92721215517585));
#54833=CARTESIAN_POINT('Ctrl Pts',(-0.418062715156936,-0.677346363895615,
1.93905071492633));
#54834=CARTESIAN_POINT('Ctrl Pts',(-0.045411969437408,-0.794677471931438,
1.95088927467681));
#54835=CARTESIAN_POINT('Ctrl Pts',(0.338179025852439,-0.720561916897015,
1.96272783442728));
#54836=CARTESIAN_POINT('Ctrl Pts',(0.640298924230299,-0.47285496710385,
1.97456639417776));
#54837=CARTESIAN_POINT('Ctrl Pts',(0.78816367389499,-0.111231978262933,
1.98640495392823));
#54838=CARTESIAN_POINT('Ctrl Pts',(0.746151009345457,0.277188021287037,
1.99824351367871));
#54839=CARTESIAN_POINT('Ctrl Pts',(0.524382247875355,0.598830361905442,
2.01008207342918));
#54840=CARTESIAN_POINT('Ctrl Pts',(0.176283960019321,0.776207743104037,
2.02192063317966));
#54841=CARTESIAN_POINT('Ctrl Pts',(-0.214283103861841,0.766588125213539,
2.03375919293014));
#54842=CARTESIAN_POINT('Ctrl Pts',(-0.553226969512226,0.572288687373625,
2.04559775268061));
#54843=CARTESIAN_POINT('Ctrl Pts',(-0.758892310758026,0.240118911410088,
2.05743631243109));
#54844=CARTESIAN_POINT('Ctrl Pts',(-0.781731996299233,-0.149898950293078,
2.06927487218156));
#54845=CARTESIAN_POINT('Ctrl Pts',(-0.616243805965499,-0.5038029747276,
2.08111343193204));
#54846=CARTESIAN_POINT('Ctrl Pts',(-0.302295462815519,-0.736338230417797,
2.09295199168251));
#54847=CARTESIAN_POINT('Ctrl Pts',(0.0844789294252334,-0.791475498675642,
2.10479055143299));
#54848=CARTESIAN_POINT('Ctrl Pts',(0.450901993898189,-0.655949162858557,
2.11662911118346));
#54849=CARTESIAN_POINT('Ctrl Pts',(0.708696584512405,-0.36237427167447,
2.12846767093394));
#54850=CARTESIAN_POINT('Ctrl Pts',(0.795760491783062,0.0184546790760481,
2.14030623068441));
#54851=CARTESIAN_POINT('Ctrl Pts',(0.691113159087595,0.394931908954148,
2.15214479043489));
#54852=CARTESIAN_POINT('Ctrl Pts',(0.51034735958526,0.582332862568382,2.16003716360187));
#54853=CARTESIAN_POINT('Ctrl Pts',(0.403075861660766,0.648960285569488,
2.16398335018536));
#54854=CARTESIAN_POINT('Ctrl Pts',(0.426788104729872,-0.598886528201364,
0.783516649814636));
#54855=CARTESIAN_POINT('Ctrl Pts',(0.525782536893907,-0.528339531245219,
0.787462836398128));
#54856=CARTESIAN_POINT('Ctrl Pts',(0.688021527733875,-0.337286270837092,
0.795355209565113));
#54857=CARTESIAN_POINT('Ctrl Pts',(0.765609474074376,0.0307725378763002,
0.807193769315585));
#54858=CARTESIAN_POINT('Ctrl Pts',(0.658755783400898,0.391327161667553,
0.819032329066062));
#54859=CARTESIAN_POINT('Ctrl Pts',(0.393199817489799,0.657650981834122,
0.830870888816538));
#54860=CARTESIAN_POINT('Ctrl Pts',(0.0329179280634981,0.765517096447697,
0.842709448567012));
#54861=CARTESIAN_POINT('Ctrl Pts',(-0.33529440331804,0.688972852766278,
0.854548008317488));
#54862=CARTESIAN_POINT('Ctrl Pts',(-0.622730501713728,0.44644168285129,
0.866386568067963));
#54863=CARTESIAN_POINT('Ctrl Pts',(-0.760143917763996,0.0963606107249503,
0.878225127818438));
#54864=CARTESIAN_POINT('Ctrl Pts',(-0.714430171726262,-0.276936261191463,
0.890063687568915));
#54865=CARTESIAN_POINT('Ctrl Pts',(-0.496602242944024,-0.583515365048949,
0.90190224731939));
#54866=CARTESIAN_POINT('Ctrl Pts',(-0.15913729329712,-0.749519484998093,
0.913740807069864));
#54867=CARTESIAN_POINT('Ctrl Pts',(0.21666560180481,-0.734955817767558,
0.925579366820341));
#54868=CARTESIAN_POINT('Ctrl Pts',(0.540271339449054,-0.543333196526847,
0.937417926570815));
#54869=CARTESIAN_POINT('Ctrl Pts',(0.733719688284525,-0.220815503453764,
0.949256486321292));
#54870=CARTESIAN_POINT('Ctrl Pts',(0.750406785607549,0.15489908152449,0.961095046071766));
#54871=CARTESIAN_POINT('Ctrl Pts',(0.586312523184101,0.493296763389096,
0.972933605822241));
#54872=CARTESIAN_POINT('Ctrl Pts',(0.280969038263487,0.712853749846213,
0.984772165572717));
#54873=CARTESIAN_POINT('Ctrl Pts',(-0.0920630200335293,0.760676324793167,
0.996610725323192));
#54874=CARTESIAN_POINT('Ctrl Pts',(-0.442916070538986,0.625243492092964,
1.00844928507367));
#54875=CARTESIAN_POINT('Ctrl Pts',(-0.68706570238818,0.3391825332396,1.02028784482414));
#54876=CARTESIAN_POINT('Ctrl Pts',(-0.765693547668255,-0.0285912792142752,
1.03212640457462));
#54877=CARTESIAN_POINT('Ctrl Pts',(-0.659857281978897,-0.38947713358653,
1.04396496432509));
#54878=CARTESIAN_POINT('Ctrl Pts',(-0.395054041498636,-0.656533605002734,
1.05580352407557));
#54879=CARTESIAN_POINT('Ctrl Pts',(-0.0350778786757769,-0.76542381240988,
1.06764208382604));
#54880=CARTESIAN_POINT('Ctrl Pts',(0.333348936140538,-0.689914891102141,
1.07948064357652));
#54881=CARTESIAN_POINT('Ctrl Pts',(0.621468276333288,-0.448197781895396,
1.091319203327));
#54882=CARTESIAN_POINT('Ctrl Pts',(0.759868981126513,-0.0985048308867328,
1.10315776307747));
#54883=CARTESIAN_POINT('Ctrl Pts',(0.715208777955099,0.274919031939008,
1.11499632282795));
#54884=CARTESIAN_POINT('Ctrl Pts',(0.498246807599315,0.582111835391569,
1.12683488257842));
#54885=CARTESIAN_POINT('Ctrl Pts',(0.161251627236223,0.749067408782359,
1.13867344232889));
#54886=CARTESIAN_POINT('Ctrl Pts',(-0.214590867632146,0.735564293393103,
1.15051200207937));
#54887=CARTESIAN_POINT('Ctrl Pts',(-0.538736030400698,0.544855540243667,
1.16235056182985));
#54888=CARTESIAN_POINT('Ctrl Pts',(-0.733093678047651,0.222885013835951,
1.17418912158032));
#54889=CARTESIAN_POINT('Ctrl Pts',(-0.75084088671136,-0.152780996948527,
1.1860276813308));
#54890=CARTESIAN_POINT('Ctrl Pts',(-0.587702155993064,-0.491640362487864,
1.19786624108127));
#54891=CARTESIAN_POINT('Ctrl Pts',(-0.28297942466279,-0.712058084290603,
1.20970480083175));
#54892=CARTESIAN_POINT('Ctrl Pts',(0.0899162044968808,-0.760933076134142,
1.22154336058222));
#54893=CARTESIAN_POINT('Ctrl Pts',(0.441150017679374,-0.626490807664069,
1.2333819203327));
#54894=CARTESIAN_POINT('Ctrl Pts',(0.686105874015599,-0.341119920009637,
1.24522048008317));
#54895=CARTESIAN_POINT('Ctrl Pts',(0.765771177142334,0.0264305589069589,
1.25705903983365));
#54896=CARTESIAN_POINT('Ctrl Pts',(0.660953667491311,0.387613621556152,
1.26889759958413));
#54897=CARTESIAN_POINT('Ctrl Pts',(0.396905051559164,0.655416241966056,
1.2807361593346));
#54898=CARTESIAN_POINT('Ctrl Pts',(0.0372375843265769,0.765321783630658,
1.29257471908508));
#54899=CARTESIAN_POINT('Ctrl Pts',(-0.331400832065067,0.690852776423943,
1.30441327883555));
#54900=CARTESIAN_POINT('Ctrl Pts',(-0.620201093821009,0.449949634302901,
1.31625183858603));
#54901=CARTESIAN_POINT('Ctrl Pts',(-0.759587998570078,0.1006486095999,1.3280903983365));
#54902=CARTESIAN_POINT('Ctrl Pts',(-0.715981687184573,-0.272899787105857,
1.33992895808698));
#54903=CARTESIAN_POINT('Ctrl Pts',(-0.49988740616552,-0.580703583029415,
1.35176751783745));
#54904=CARTESIAN_POINT('Ctrl Pts',(-0.163364676656491,-0.748609412582429,
1.36360607758793));
#54905=CARTESIAN_POINT('Ctrl Pts',(0.212514424517749,-0.736166889745784,
1.3754446373384));
#54906=CARTESIAN_POINT('Ctrl Pts',(0.537196431884951,-0.546373556970108,
1.38728319708888));
#54907=CARTESIAN_POINT('Ctrl Pts',(0.732461830575209,-0.22495274378523,
1.39912175683935));
#54908=CARTESIAN_POINT('Ctrl Pts',(0.751269009381666,0.150661692970645,
1.41096031658983));
#54909=CARTESIAN_POINT('Ctrl Pts',(0.589087109282469,0.489980048433928,
1.4227988763403));
#54910=CARTESIAN_POINT('Ctrl Pts',(0.284987557885531,0.711256748324071,
1.43463743609078));
#54911=CARTESIAN_POINT('Ctrl Pts',(-0.0877686730192269,0.761183769021999,
1.44647599584126));
#54912=CARTESIAN_POINT('Ctrl Pts',(-0.439380452218736,0.627733134695109,
1.45831455559173));
#54913=CARTESIAN_POINT('Ctrl Pts',(-0.685140582617146,0.343054590753614,
1.47015311534221));
#54914=CARTESIAN_POINT('Ctrl Pts',(-0.765842709264246,-0.0242696281984333,
1.48199167509268));
#54915=CARTESIAN_POINT('Ctrl Pts',(-0.662044790248036,-0.385747023179083,
1.49383023484316));
#54916=CARTESIAN_POINT('Ctrl Pts',(-0.398752901315645,-0.654293660276825,
1.50566879459363));
#54917=CARTESIAN_POINT('Ctrl Pts',(-0.0393969934781305,-0.765213661071844,
1.51750735434411));
#54918=CARTESIAN_POINT('Ctrl Pts',(0.329450089254417,-0.69178516092523,
1.52934591409458));
#54919=CARTESIAN_POINT('Ctrl Pts',(0.618928973039669,-0.451697904044452,
1.54118447384506));
#54920=CARTESIAN_POINT('Ctrl Pts',(0.759300967894857,-0.102791586912663,
1.55302303359553));
#54921=CARTESIAN_POINT('Ctrl Pts',(0.716748895504719,0.270878369344724,
1.56486159334601));
#54922=CARTESIAN_POINT('Ctrl Pts',(0.501524024444482,0.579290706891713,
1.57670015309648));
#54923=CARTESIAN_POINT('Ctrl Pts',(0.165476425307159,0.748145455679345,
1.58853871284696));
#54924=CARTESIAN_POINT('Ctrl Pts',(-0.210436289285403,0.736763624467089,
1.60037727259744));
#54925=CARTESIAN_POINT('Ctrl Pts',(-0.535652556013789,0.54788722326952,
1.61221583234791));
#54926=CARTESIAN_POINT('Ctrl Pts',(-0.731824150972487,0.227018682578084,
1.62405439209838));
#54927=CARTESIAN_POINT('Ctrl Pts',(-0.751691150172023,-0.148541189368984,
1.63589295184886));
#54928=CARTESIAN_POINT('Ctrl Pts',(-0.59046737204382,-0.488315832978776,
1.64773151159934));
#54929=CARTESIAN_POINT('Ctrl Pts',(-0.286993421932599,-0.710449749069916,
1.65957007134981));
#54930=CARTESIAN_POINT('Ctrl Pts',(0.0856204426951459,-0.761428401084946,
1.67140863110029));
#54931=CARTESIAN_POINT('Ctrl Pts',(0.437607388249466,-0.628970463484234,
1.68324719085076));
#54932=CARTESIAN_POINT('Ctrl Pts',(0.684169835877579,-0.344986529970863,
1.69508575060124));
#54933=CARTESIAN_POINT('Ctrl Pts',(0.765908143465054,0.0221085042462033,
1.70692431035171));
#54934=CARTESIAN_POINT('Ctrl Pts',(0.663130641560838,0.383877353342446,
1.71876287010219));
#54935=CARTESIAN_POINT('Ctrl Pts',(0.400597576054987,0.653165868861011,
1.73060142985266));
#54936=CARTESIAN_POINT('Ctrl Pts',(0.0415560889363424,0.765099445600639,
1.74243998960314));
#54937=CARTESIAN_POINT('Ctrl Pts',(-0.327496723241085,0.692712037178827,
1.75427854935361));
#54938=CARTESIAN_POINT('Ctrl Pts',(-0.617651924118387,0.453442577201289,
1.76611710910409));
#54939=CARTESIAN_POINT('Ctrl Pts',(-0.759007891386282,0.104933745761025,
1.77795566885456));
#54940=CARTESIAN_POINT('Ctrl Pts',(-0.717510396806747,-0.268854794750451,
1.78979422860504));
#54941=CARTESIAN_POINT('Ctrl Pts',(-0.503156649404848,-0.577873218228538,
1.80163278835552));
#54942=CARTESIAN_POINT('Ctrl Pts',(-0.16758685637372,-0.747675541767138,
1.81347134810599));
#54943=CARTESIAN_POINT('Ctrl Pts',(0.208356478481988,-0.737354492805756,
1.82530990785647));
#54944=CARTESIAN_POINT('Ctrl Pts',(0.534104415080109,-0.549396527089301,
1.83714846760694));
#54945=CARTESIAN_POINT('Ctrl Pts',(0.731180644316946,-0.229082813765163,
1.84898702735742));
#54946=CARTESIAN_POINT('Ctrl Pts',(0.752107305721148,0.146419503028601,
1.86082558710789));
#54947=CARTESIAN_POINT('Ctrl Pts',(0.591842933287032,0.486647729371899,
1.87266414685837));
#54948=CARTESIAN_POINT('Ctrl Pts',(0.288997000832408,0.709637092956943,
1.88450270660884));
#54949=CARTESIAN_POINT('Ctrl Pts',(-0.0834715306293183,0.761666970368852,
1.89634126635932));
#54950=CARTESIAN_POINT('Ctrl Pts',(-0.43583083988997,0.630202784191798,
1.90817982610979));
#54951=CARTESIAN_POINT('Ctrl Pts',(-0.683193641525102,0.346915722254021,
1.92001838586027));
#54952=CARTESIAN_POINT('Ctrl Pts',(-0.765967479226197,-0.0199472042093853,
1.93185694561075));
#54953=CARTESIAN_POINT('Ctrl Pts',(-0.664211212778921,-0.382004627029242,
1.94369550536122));
#54954=CARTESIAN_POINT('Ctrl Pts',(-0.402439061098776,-0.652032876508719,
1.9555340651117));
#54955=CARTESIAN_POINT('Ctrl Pts',(-0.043714853490764,-0.764979138501708,
1.96737262486217));
#54956=CARTESIAN_POINT('Ctrl Pts',(0.325540749541049,-0.69363339706272,
1.97921118461265));
#54957=CARTESIAN_POINT('Ctrl Pts',(0.616369957299513,-0.45518364134848,
1.99104974436312));
#54958=CARTESIAN_POINT('Ctrl Pts',(0.758708771231593,-0.10707506618831,
2.0028883041136));
#54959=CARTESIAN_POINT('Ctrl Pts',(0.718266185316642,0.266829073701797,
2.01472686386407));
#54960=CARTESIAN_POINT('Ctrl Pts',(0.504785267475012,0.576451139662625,
2.02656542361455));
#54961=CARTESIAN_POINT('Ctrl Pts',(0.169695954183138,0.747199652174499,
2.03840398336502));
#54962=CARTESIAN_POINT('Ctrl Pts',(-0.206275010903853,0.737939534370098,
2.0502425431155));
#54963=CARTESIAN_POINT('Ctrl Pts',(-0.532552016989714,0.550901368799743,
2.06208110286597));
#54964=CARTESIAN_POINT('Ctrl Pts',(-0.730531324473397,0.231145294130476,
2.07391966261645));
#54965=CARTESIAN_POINT('Ctrl Pts',(-0.752517455433544,-0.144296993318319,
2.08575822236692));
#54966=CARTESIAN_POINT('Ctrl Pts',(-0.593213816227538,-0.484975073780585,
2.09759678211741));
#54967=CARTESIAN_POINT('Ctrl Pts',(-0.290998211079956,-0.708820125203544,
2.10943534186787));
#54968=CARTESIAN_POINT('Ctrl Pts',(0.0813218204062015,-0.761896827967887,
2.12127390161836));
#54969=CARTESIAN_POINT('Ctrl Pts',(0.434051084904416,-0.631435322162685,
2.13311246136882));
#54970=CARTESIAN_POINT('Ctrl Pts',(0.682211490608578,-0.348831781385437,
2.1449510211193));
#54971=CARTESIAN_POINT('Ctrl Pts',(0.766021684216589,0.0177649990084773,
2.15678958086977));
#54972=CARTESIAN_POINT('Ctrl Pts',(0.665285185146957,0.38017268910908,2.16862814062025));
#54973=CARTESIAN_POINT('Ctrl Pts',(0.491274884794816,0.560570177541447,
2.17652051378724));
#54974=CARTESIAN_POINT('Ctrl Pts',(0.388012289633257,0.624707630090715,
2.18046670037073));
#54975=CARTESIAN_POINT('Ctrl Pts',(0.410219162127157,-0.575636310115765,
0.8));
#54976=CARTESIAN_POINT('Ctrl Pts',(0.50537039190027,-0.507828117569598,
0.803946186583492));
#54977=CARTESIAN_POINT('Ctrl Pts',(0.661310874189135,-0.324192005087297,
0.811838559750475));
#54978=CARTESIAN_POINT('Ctrl Pts',(0.735886669498874,0.0295778738072663,
0.82367711950095));
#54979=CARTESIAN_POINT('Ctrl Pts',(0.633181296569113,0.376134898320248,
0.835515679251426));
#54980=CARTESIAN_POINT('Ctrl Pts',(0.377934853131171,0.632119386061258,
0.847354239001902));
#54981=CARTESIAN_POINT('Ctrl Pts',(0.0316399747779213,0.735797878194255,
0.859192798752376));
#54982=CARTESIAN_POINT('Ctrl Pts',(-0.322277466664887,0.662225266491492,
0.871031358502852));
#54983=CARTESIAN_POINT('Ctrl Pts',(-0.598554603122584,0.429109740989168,
0.882869918253328));
#54984=CARTESIAN_POINT('Ctrl Pts',(-0.730633299254123,0.0926196596286783,
0.894708478003802));
#54985=CARTESIAN_POINT('Ctrl Pts',(-0.686694270988179,-0.266184928233867,
0.906547037754278));
#54986=CARTESIAN_POINT('Ctrl Pts',(-0.47732294727357,-0.560861892554869,
0.918385597504754));
#54987=CARTESIAN_POINT('Ctrl Pts',(-0.152959200118396,-0.720421332568536,
0.930224157255227));
#54988=CARTESIAN_POINT('Ctrl Pts',(0.20825412107116,-0.70642306199211,0.942062717005705));
#54989=CARTESIAN_POINT('Ctrl Pts',(0.519296704228398,-0.522239692636662,
0.953901276756179));
#54990=CARTESIAN_POINT('Ctrl Pts',(0.705234922034154,-0.212242913538608,
0.965739836506655));
#54991=CARTESIAN_POINT('Ctrl Pts',(0.721274186030318,0.148885525939063,
0.97757839625713));
#54992=CARTESIAN_POINT('Ctrl Pts',(0.563550458271255,0.474145794399759,
0.989416956007605));
#54993=CARTESIAN_POINT('Ctrl Pts',(0.270061143182683,0.68517904960402,1.00125551575808));
#54994=CARTESIAN_POINT('Ctrl Pts',(-0.0884889117632597,0.731145036959546,
1.01309407550856));
#54995=CARTESIAN_POINT('Ctrl Pts',(-0.425721001442049,0.600970033160064,
1.02493263525903));
#54996=CARTESIAN_POINT('Ctrl Pts',(-0.660392156286491,0.326014650014156,
1.03677119500951));
#54997=CARTESIAN_POINT('Ctrl Pts',(-0.735967479153258,-0.0274812968624031,
1.04860975475998));
#54998=CARTESIAN_POINT('Ctrl Pts',(-0.634240032318171,-0.374356692787108,
1.06044831451046));
#54999=CARTESIAN_POINT('Ctrl Pts',(-0.379717091696098,-0.631045388490867,
1.07228687426093));
#55000=CARTESIAN_POINT('Ctrl Pts',(-0.0337160709028718,-0.73570821566756,
1.08412543401141));
#55001=CARTESIAN_POINT('Ctrl Pts',(0.320407527210959,-0.663130732629247,
1.09596399376188));
#55002=CARTESIAN_POINT('Ctrl Pts',(0.597341380372839,-0.430797664036932,
1.10780255351236));
#55003=CARTESIAN_POINT('Ctrl Pts',(0.730369036319385,-0.094680635997126,
1.11964111326283));
#55004=CARTESIAN_POINT('Ctrl Pts',(0.687442649847106,0.264246012681654,
1.13147967301331));
#55005=CARTESIAN_POINT('Ctrl Pts',(0.478903665966244,0.559512851300696,
1.14331823276378));
#55006=CARTESIAN_POINT('Ctrl Pts',(0.154991450519341,0.719986807040808,
1.15515679251426));
#55007=CARTESIAN_POINT('Ctrl Pts',(-0.206259933078302,0.707007915127706,
1.16699535226474));
#55008=CARTESIAN_POINT('Ctrl Pts',(-0.51782099957674,0.523702935302196,
1.17883391201521));
#55009=CARTESIAN_POINT('Ctrl Pts',(-0.704633215023091,0.214232080541122,
1.19067247176569));
#55010=CARTESIAN_POINT('Ctrl Pts',(-0.721691434283282,-0.146849670510018,
1.20251103151616));
#55011=CARTESIAN_POINT('Ctrl Pts',(-0.564886142186152,-0.472553698972733,
1.21434959126664));
#55012=CARTESIAN_POINT('Ctrl Pts',(-0.271993481537794,-0.684414273702493,
1.22618815101711));
#55013=CARTESIAN_POINT('Ctrl Pts',(0.0864254407786529,-0.731391820594802,
1.23802671076759));
#55014=CARTESIAN_POINT('Ctrl Pts',(0.42402351100988,-0.602168924935201,
1.24986527051806));
#55015=CARTESIAN_POINT('Ctrl Pts',(0.65946959076411,-0.327876822761505,
1.26170383026854));
#55016=CARTESIAN_POINT('Ctrl Pts',(0.7360420948641,0.02540446092383,1.27354239001901));
#55017=CARTESIAN_POINT('Ctrl Pts',(0.635293853503172,0.372565526784018,
1.28538094976949));
#55018=CARTESIAN_POINT('Ctrl Pts',(0.381496241085932,0.62997140417964,1.29721950951997));
#55019=CARTESIAN_POINT('Ctrl Pts',(0.0357919315763396,0.735610147891393,
1.30905806927044));
#55020=CARTESIAN_POINT('Ctrl Pts',(-0.318535053229798,0.664032206982953,
1.32089662902092));
#55021=CARTESIAN_POINT('Ctrl Pts',(-0.596123392939055,0.432481505312761,
1.33273518877139));
#55022=CARTESIAN_POINT('Ctrl Pts',(-0.730098962182839,0.0967411880550564,
1.34457374852187));
#55023=CARTESIAN_POINT('Ctrl Pts',(-0.68818555287791,-0.262305159798444,
1.35641230827234));
#55024=CARTESIAN_POINT('Ctrl Pts',(-0.480480572542965,-0.558159270688526,
1.36825086802282));
#55025=CARTESIAN_POINT('Ctrl Pts',(-0.157022466269567,-0.719546591356936,
1.38008942777329));
#55026=CARTESIAN_POINT('Ctrl Pts',(0.204264102488947,-0.707587117237976,
1.39192798752377));
#55027=CARTESIAN_POINT('Ctrl Pts',(0.516341171985148,-0.525162018961544,
1.40376654727424));
#55028=CARTESIAN_POINT('Ctrl Pts',(0.704025897392014,-0.216219536231424,
1.41560510702472));
#55029=CARTESIAN_POINT('Ctrl Pts',(0.722102936199932,0.144812643019176,
1.42744366677519));
#55030=CARTESIAN_POINT('Ctrl Pts',(0.566217328251717,0.470957842311017,
1.43928222652567));
#55031=CARTESIAN_POINT('Ctrl Pts',(0.273923654190083,0.683644047529059,
1.45112078627614));
#55032=CARTESIAN_POINT('Ctrl Pts',(-0.0843612816475947,0.73163278098069,
1.46295934602662));
#55033=CARTESIAN_POINT('Ctrl Pts',(-0.422322644344321,0.603363021837419,
1.4747979057771));
#55034=CARTESIAN_POINT('Ctrl Pts',(-0.658541774303685,0.32973638492547,
1.48663646552757));
#55035=CARTESIAN_POINT('Ctrl Pts',(-0.736110849936677,-0.0233274227523295,
1.49847502527805));
#55036=CARTESIAN_POINT('Ctrl Pts',(-0.636342616245341,-0.370771394253652,
1.51031358502852));
#55037=CARTESIAN_POINT('Ctrl Pts',(-0.383272352862338,-0.628892403816528,
1.522152144779));
#55038=CARTESIAN_POINT('Ctrl Pts',(-0.0378675072613757,-0.735506222910841,
1.53399070452947));
#55039=CARTESIAN_POINT('Ctrl Pts',(0.316660042955515,-0.664928394071252,
1.54582926427995));
#55040=CARTESIAN_POINT('Ctrl Pts',(0.594900658951714,-0.434161903010362,
1.55766782403042));
#55041=CARTESIAN_POINT('Ctrl Pts',(0.729823074730051,-0.0988009698248782,
1.5695063837809));
#55042=CARTESIAN_POINT('Ctrl Pts',(0.688922976322423,0.260362218345552,
1.58134494353137));
#55043=CARTESIAN_POINT('Ctrl Pts',(0.482053653356788,0.556801245806918,
1.59318350328185));
#55044=CARTESIAN_POINT('Ctrl Pts',(0.159052231749204,0.719100646378767,
1.60502206303232));
#55045=CARTESIAN_POINT('Ctrl Pts',(-0.202266645473739,0.708160685279523,
1.6168606227828));
#55046=CARTESIAN_POINT('Ctrl Pts',(-0.514857233095386,0.526616921087925,
1.62869918253327));
#55047=CARTESIAN_POINT('Ctrl Pts',(-0.703412974048005,0.218205270302308,
1.64053774228375));
#55048=CARTESIAN_POINT('Ctrl Pts',(-0.722508688467628,-0.142774462476838,
1.65237630203423));
#55049=CARTESIAN_POINT('Ctrl Pts',(-0.567544005886828,-0.469358235709884,
1.6642148617847));
#55050=CARTESIAN_POINT('Ctrl Pts',(-0.275851645761568,-0.682868377930474,
1.67605342153517));
#55051=CARTESIAN_POINT('Ctrl Pts',(0.0822964508010132,-0.731867915837495,
1.68789198128565));
#55052=CARTESIAN_POINT('Ctrl Pts',(0.420618414990665,-0.604552314541516,
1.69973054103613));
#55053=CARTESIAN_POINT('Ctrl Pts',(0.657608714291634,-0.331593321607157,
1.7115691007866));
#55054=CARTESIAN_POINT('Ctrl Pts',(0.736173743824141,0.0212501988393111,
1.72340766053708));
#55055=CARTESIAN_POINT('Ctrl Pts',(0.637386312193742,0.36897430950518,1.73524622028755));
#55056=CARTESIAN_POINT('Ctrl Pts',(0.38504541288342,0.627808395980971,1.74708478003803));
#55057=CARTESIAN_POINT('Ctrl Pts',(0.0399427814314016,0.735396441559441,
1.7589233397885));
#55058=CARTESIAN_POINT('Ctrl Pts',(-0.314782511317597,0.665819286755307,
1.77076189953898));
#55059=CARTESIAN_POINT('Ctrl Pts',(-0.5936731881467,0.435838843751334,1.78260045928945));
#55060=CARTESIAN_POINT('Ctrl Pts',(-0.729541376157727,0.100859964905057,
1.79443901903993));
#55061=CARTESIAN_POINT('Ctrl Pts',(-0.689654914309015,-0.258417203792979,
1.8062775787904));
#55062=CARTESIAN_POINT('Ctrl Pts',(-0.483622895882263,-0.55543878746919,
1.81811613854088));
#55063=CARTESIAN_POINT('Ctrl Pts',(-0.161080730796523,-0.718648975656924,
1.82995469829136));
#55064=CARTESIAN_POINT('Ctrl Pts',(0.200267577937169,-0.708728614685542,
1.84179325804183));
#55065=CARTESIAN_POINT('Ctrl Pts',(0.513369194723111,-0.528067630096644,
1.85363181779231));
#55066=CARTESIAN_POINT('Ctrl Pts',(0.702794449871408,-0.22018926694303,
1.86547037754278));
#55067=CARTESIAN_POINT('Ctrl Pts',(0.722908687855579,0.140735145112547,
1.87730893729326));
#55068=CARTESIAN_POINT('Ctrl Pts',(0.568866164528063,0.467754891904443,
1.88914749704373));
#55069=CARTESIAN_POINT('Ctrl Pts',(0.277777440900717,0.68208727108596,1.90098605679421));
#55070=CARTESIAN_POINT('Ctrl Pts',(-0.0802309646795408,0.732097223286951,
1.91282461654468));
#55071=CARTESIAN_POINT('Ctrl Pts',(-0.418910836519209,0.605736793589845,
1.92466317629516));
#55072=CARTESIAN_POINT('Ctrl Pts',(-0.656670418156131,0.333447617997354,
1.93650173604563));
#55073=CARTESIAN_POINT('Ctrl Pts',(-0.736230776028063,-0.0191728056777326,
1.94834029579611));
#55074=CARTESIAN_POINT('Ctrl Pts',(-0.638424933033424,-0.367174286939925,
1.96017885554658));
#55075=CARTESIAN_POINT('Ctrl Pts',(-0.386815407040617,-0.626719389121822,
1.97201741529706));
#55076=CARTESIAN_POINT('Ctrl Pts',(-0.0420177375441198,-0.735280805071978,
1.98385597504754));
#55077=CARTESIAN_POINT('Ctrl Pts',(0.312902473229659,-0.666704877228424,
1.99569453479801));
#55078=CARTESIAN_POINT('Ctrl Pts',(0.592440990368726,-0.437512315593109,
2.00753309454849));
#55079=CARTESIAN_POINT('Ctrl Pts',(0.729253868568196,-0.102918154113688,
2.01937165429896));
#55080=CARTESIAN_POINT('Ctrl Pts',(0.690381361287827,0.256470126116556,
2.03121021404944));
#55081=CARTESIAN_POINT('Ctrl Pts',(0.485188287074669,0.554071917419808,
2.04304877379991));
#55082=CARTESIAN_POINT('Ctrl Pts',(0.163107948346954,0.718191561244962,
2.05488733355038));
#55083=CARTESIAN_POINT('Ctrl Pts',(-0.198266917945865,0.709290943526656,
2.06672589330087));
#55084=CARTESIAN_POINT('Ctrl Pts',(-0.511877064467201,0.529514050225861,
2.07856445305133));
#55085=CARTESIAN_POINT('Ctrl Pts',(-0.70217033818877,0.222171676850865,
2.09040301280182));
#55086=CARTESIAN_POINT('Ctrl Pts',(-0.723302914567855,-0.138695036343561,
2.10224157255228));
#55087=CARTESIAN_POINT('Ctrl Pts',(-0.570183826489577,-0.466147172833569,
2.11408013230277));
#55088=CARTESIAN_POINT('Ctrl Pts',(-0.279700959344392,-0.681302019989293,
2.12591869205323));
#55089=CARTESIAN_POINT('Ctrl Pts',(0.078164711387169,-0.732318157260131,
2.13775725180372));
#55090=CARTESIAN_POINT('Ctrl Pts',(0.417200175910644,-0.606921481466812,
2.14959581155419));
#55091=CARTESIAN_POINT('Ctrl Pts',(0.655726396704751,-0.335289291096404,
2.16143437130467));
#55092=CARTESIAN_POINT('Ctrl Pts',(0.736282876650117,0.0170753189409072,
2.17327293105514));
#55093=CARTESIAN_POINT('Ctrl Pts',(0.639457211206318,0.365413469264011,
2.18511149080562));
#55094=CARTESIAN_POINT('Ctrl Pts',(0.472202410004372,0.538807492514513,
2.1930038639726));
#55095=CARTESIAN_POINT('Ctrl Pts',(0.372948717605748,0.600454974611942,
2.19695005055609));
#55096=CARTESIAN_POINT('Ctrl Pts',(0.345504974425206,0.713245911452249,
0.8));
#55097=CARTESIAN_POINT('Ctrl Pts',(0.36583353368801,0.702081547762358,0.8));
#55098=CARTESIAN_POINT('Ctrl Pts',(0.385637643802227,0.690039175705666,
0.8));
#55099=CARTESIAN_POINT('Ctrl Pts',(0.404853295913343,0.677138077406943,
0.8));
#55100=CARTESIAN_POINT('Ctrl Pts',(0.431589435756686,0.659187837349888,
0.8));
#55101=CARTESIAN_POINT('Ctrl Pts',(0.457187440867682,0.63957581308399,0.8));
#55102=CARTESIAN_POINT('Ctrl Pts',(0.481519180772095,0.618436888473522,
0.8));
#55103=CARTESIAN_POINT('Ctrl Pts',(0.490041012870151,0.611033292718694,
0.8));
#55104=CARTESIAN_POINT('Ctrl Pts',(0.498407317172348,0.603442222277882,
0.8));
#55105=CARTESIAN_POINT('Ctrl Pts',(0.506611886748092,0.595668956909438,
0.8));
#55106=CARTESIAN_POINT('Ctrl Pts',(0.512987438654641,0.589628559983995,
0.8));
#55107=CARTESIAN_POINT('Ctrl Pts',(0.519262318463782,0.583480863158659,
0.8));
#55108=CARTESIAN_POINT('Ctrl Pts',(0.525428333131113,0.577234389533608,
0.8));
#55109=CARTESIAN_POINT('Ctrl Pts',(0.552361828544955,0.549949444912184,
0.8));
#55110=CARTESIAN_POINT('Ctrl Pts',(0.577255825711188,0.520751087178113,
0.8));
#55111=CARTESIAN_POINT('Ctrl Pts',(0.599886914660718,0.48986502862222,0.8));
#55112=CARTESIAN_POINT('Ctrl Pts',(0.609541659734953,0.4766885958677,0.8));
#55113=CARTESIAN_POINT('Ctrl Pts',(0.618783914351497,0.463204566301741,
0.8));
#55114=CARTESIAN_POINT('Ctrl Pts',(0.627593177155457,0.449428880659182,
0.8));
#55115=CARTESIAN_POINT('Ctrl Pts',(0.633449833557471,0.440270400624467,
0.8));
#55116=CARTESIAN_POINT('Ctrl Pts',(0.639117093402895,0.43097907060152,0.8));
#55117=CARTESIAN_POINT('Ctrl Pts',(0.64457466299164,0.421584382346768,0.8));
#55118=CARTESIAN_POINT('Ctrl Pts',(0.650150271728973,0.411986500896801,
0.8));
#55119=CARTESIAN_POINT('Ctrl Pts',(0.655510064988793,0.402276354406898,
0.8));
#55120=CARTESIAN_POINT('Ctrl Pts',(0.660649057912794,0.392459620153433,
0.8));
#55121=CARTESIAN_POINT('Ctrl Pts',(0.677398500727402,0.360464084951061,
0.8));
#55122=CARTESIAN_POINT('Ctrl Pts',(0.691806162809588,0.327337699200768,
0.8));
#55123=CARTESIAN_POINT('Ctrl Pts',(0.703820537250413,0.29335172176486,0.8));
#55124=CARTESIAN_POINT('Ctrl Pts',(0.712004329212203,0.270201605183803,
0.8));
#55125=CARTESIAN_POINT('Ctrl Pts',(0.719076667813015,0.246652090573615,
0.8));
#55126=CARTESIAN_POINT('Ctrl Pts',(0.725007698830821,0.222786213838172,
0.8));
#55127=CARTESIAN_POINT('Ctrl Pts',(0.729682972771009,0.203973378223933,
0.8));
#55128=CARTESIAN_POINT('Ctrl Pts',(0.73364885638524,0.184963897214997,0.8));
#55129=CARTESIAN_POINT('Ctrl Pts',(0.73688566164746,0.165798785722696,0.8));
#55130=CARTESIAN_POINT('Ctrl Pts',(0.738101009586174,0.158602715258016,
0.8));
#55131=CARTESIAN_POINT('Ctrl Pts',(0.739213253909337,0.151385563578606,
0.8));
#55132=CARTESIAN_POINT('Ctrl Pts',(0.740219854302973,0.144162331267803,
0.8));
#55133=CARTESIAN_POINT('Ctrl Pts',(0.745122019678705,0.108985035929166,
0.8));
#55134=CARTESIAN_POINT('Ctrl Pts',(0.747536860054795,0.0735840120457708,
0.8));
#55135=CARTESIAN_POINT('Ctrl Pts',(0.747398095781194,0.038213143437428,
0.8));
#55136=CARTESIAN_POINT('Ctrl Pts',(0.747387383346823,0.0354825550893366,
0.8));
#55137=CARTESIAN_POINT('Ctrl Pts',(0.747361426528289,0.0327521458004539,
0.8));
#55138=CARTESIAN_POINT('Ctrl Pts',(0.747320181801601,0.030022032614301,
0.8));
#55139=CARTESIAN_POINT('Ctrl Pts',(0.746859569917307,-0.000467260926602417,
0.8));
#55140=CARTESIAN_POINT('Ctrl Pts',(0.744494531099263,-0.0309202575391632,
0.8));
#55141=CARTESIAN_POINT('Ctrl Pts',(0.740261770482073,-0.0611646713267921,
0.8));
#55142=CARTESIAN_POINT('Ctrl Pts',(0.737719428203378,-0.0793305112645305,
0.8));
#55143=CARTESIAN_POINT('Ctrl Pts',(0.734502747220283,-0.0974209830990813,
0.8));
#55144=CARTESIAN_POINT('Ctrl Pts',(0.730615146452625,-0.115396704760788,
0.8));
#55145=CARTESIAN_POINT('Ctrl Pts',(0.728559969813086,-0.124899553804686,
0.8));
#55146=CARTESIAN_POINT('Ctrl Pts',(0.72631599569988,-0.134374304191129,
0.8));
#55147=CARTESIAN_POINT('Ctrl Pts',(0.723890962231601,-0.143787847611887,
0.8));
#55148=CARTESIAN_POINT('Ctrl Pts',(0.71517862288476,-0.177607580745754,
0.8));
#55149=CARTESIAN_POINT('Ctrl Pts',(0.704121082802721,-0.210704194639309,
0.8));
#55150=CARTESIAN_POINT('Ctrl Pts',(0.690789930854426,-0.242823645553218,
0.8));
#55151=CARTESIAN_POINT('Ctrl Pts',(0.679792305406727,-0.269320807396919,
0.8));
#55152=CARTESIAN_POINT('Ctrl Pts',(0.667246321255119,-0.295153115200466,
0.8));
#55153=CARTESIAN_POINT('Ctrl Pts',(0.653168640005758,-0.320165218334144,
0.8));
#55154=CARTESIAN_POINT('Ctrl Pts',(0.645345018624938,-0.334065605861727,
0.8));
#55155=CARTESIAN_POINT('Ctrl Pts',(0.637047938644404,-0.347712405880769,
0.8));
#55156=CARTESIAN_POINT('Ctrl Pts',(0.628293128421847,-0.36108455082462,
0.8));
#55157=CARTESIAN_POINT('Ctrl Pts',(0.623632127364847,-0.368203789292754,
0.8));
#55158=CARTESIAN_POINT('Ctrl Pts',(0.618841361406744,-0.375245149184032,
0.8));
#55159=CARTESIAN_POINT('Ctrl Pts',(0.613923051360153,-0.382205232791639,
0.8));
#55160=CARTESIAN_POINT('Ctrl Pts',(0.610216510191735,-0.387450497157415,
0.8));
#55161=CARTESIAN_POINT('Ctrl Pts',(0.606438371485466,-0.392648260874719,
0.8));
#55162=CARTESIAN_POINT('Ctrl Pts',(0.602595484873438,-0.397789698506065,
0.8));
#55163=CARTESIAN_POINT('Ctrl Pts',(0.581986083819865,-0.425363228728034,
0.8));
#55164=CARTESIAN_POINT('Ctrl Pts',(0.559474301213147,-0.451381505199937,
0.8));
#55165=CARTESIAN_POINT('Ctrl Pts',(0.535252367285333,-0.475662926269611,
0.8));
#55166=CARTESIAN_POINT('Ctrl Pts',(0.511393995304302,-0.499579892513297,
0.8));
#55167=CARTESIAN_POINT('Ctrl Pts',(0.485875450752161,-0.521812462744942,
0.8));
#55168=CARTESIAN_POINT('Ctrl Pts',(0.458849939885056,-0.542148155172804,
0.8));
#55169=CARTESIAN_POINT('Ctrl Pts',(0.443140321239726,-0.55396905929933,
0.8));
#55170=CARTESIAN_POINT('Ctrl Pts',(0.426921009928925,-0.565148233479232,
0.8));
#55171=CARTESIAN_POINT('Ctrl Pts',(0.410219162127159,-0.575636310115764,
0.8));
#55172=CARTESIAN_POINT('Ctrl Pts',(0.418139433688274,0.673212941048261,
2.1475));
#55173=CARTESIAN_POINT('Ctrl Pts',(0.529419834375704,0.604095547595317,
2.14355381341651));
#55174=CARTESIAN_POINT('Ctrl Pts',(0.623180483701969,0.506893338197268,
2.13960762683302));
#55175=CARTESIAN_POINT('Ctrl Pts',(0.688153836085317,0.393201105222312,
2.13566144024952));
#55176=CARTESIAN_POINT('Ctrl Pts',(0.753127188468667,0.279508872247353,
2.13171525366603));
#55177=CARTESIAN_POINT('Ctrl Pts',(0.789313243909101,0.149326615695483,
2.12776906708254));
#55178=CARTESIAN_POINT('Ctrl Pts',(0.7923533348071,0.0183919672350275,2.12382288049905));
#55179=CARTESIAN_POINT('Ctrl Pts',(0.795393425705099,-0.112542681225426,
2.11987669391556));
#55180=CARTESIAN_POINT('Ctrl Pts',(0.765287552060666,-0.244229721594463,
2.11593050733207));
#55181=CARTESIAN_POINT('Ctrl Pts',(0.705663152651071,-0.360830948710805,
2.11198432074857));
#55182=CARTESIAN_POINT('Ctrl Pts',(0.646038753241476,-0.477432175827145,
2.10803813416508));
#55183=CARTESIAN_POINT('Ctrl Pts',(0.556895828066718,-0.578947589690789,
2.10409194758159));
#55184=CARTESIAN_POINT('Ctrl Pts',(0.448971554738058,-0.653137157594104,
2.1001457609981));
#55185=CARTESIAN_POINT('Ctrl Pts',(0.341047281409397,-0.72732672549742,
2.09619957441461));
#55186=CARTESIAN_POINT('Ctrl Pts',(0.214341659926831,-0.774190447440409,
2.09225338783112));
#55187=CARTESIAN_POINT('Ctrl Pts',(0.0841173903529904,-0.788089336120012,
2.08830720124762));
#55188=CARTESIAN_POINT('Ctrl Pts',(-0.04610687922085,-0.801988224799615,
2.08436101466413));
#55189=CARTESIAN_POINT('Ctrl Pts',(-0.179849796885967,-0.782922280215831,
2.08041482808064));
#55190=CARTESIAN_POINT('Ctrl Pts',(-0.301001435910588,-0.733185064597701,
2.07646864149715));
#55191=CARTESIAN_POINT('Ctrl Pts',(-0.42215307493521,-0.68344784897957,
2.07252245491366));
#55192=CARTESIAN_POINT('Ctrl Pts',(-0.530713435319334,-0.603039362327094,
2.06857626833016));
#55193=CARTESIAN_POINT('Ctrl Pts',(-0.613605739088308,-0.501646790933058,
2.06463008174667));
#55194=CARTESIAN_POINT('Ctrl Pts',(-0.696498042857281,-0.400254219539023,
2.06068389516318));
#55195=CARTESIAN_POINT('Ctrl Pts',(-0.753722290011102,-0.277877563403429,
2.05673770857969));
#55196=CARTESIAN_POINT('Ctrl Pts',(-0.778385540234301,-0.149256996009377,
2.0527915219962));
#55197=CARTESIAN_POINT('Ctrl Pts',(-0.787807963541229,-0.100118402312424,
2.05128390884297));
#55198=CARTESIAN_POINT('Ctrl Pts',(-0.792477884965536,-0.0500684667399751,
2.04977629568975));
#55199=CARTESIAN_POINT('Ctrl Pts',(-0.792448351156449,-1.30718296499355E-5,
2.04826868253652));
#55200=CARTESIAN_POINT('Origin',(0.,0.,1.095));
#55201=CARTESIAN_POINT('Origin',(0.,0.,2.1475));
#55202=CARTESIAN_POINT('Ctrl Pts',(0.82685,-1.18395083925468E-14,-1.12625));
#55203=CARTESIAN_POINT('Ctrl Pts',(0.826850000000002,0.135161967341259,
-1.12277201246584));
#55204=CARTESIAN_POINT('Ctrl Pts',(0.759329854291363,0.405358483866941,
-1.11581603739752));
#55205=CARTESIAN_POINT('Ctrl Pts',(0.478857035684602,0.715228292912721,
-1.10538207479504));
#55206=CARTESIAN_POINT('Ctrl Pts',(0.0855976892416321,0.856457731826549,
-1.09494811219256));
#55207=CARTESIAN_POINT('Ctrl Pts',(-0.327878991306288,0.795839011623238,
-1.08451414959008));
#55208=CARTESIAN_POINT('Ctrl Pts',(-0.664050737432057,0.547619885496967,
-1.0740801869876));
#55209=CARTESIAN_POINT('Ctrl Pts',(-0.843710039187729,0.170328555651523,
-1.06364622438512));
#55210=CARTESIAN_POINT('Ctrl Pts',(-0.82449358245641,-0.247114352893216,
-1.05321226178264));
#55211=CARTESIAN_POINT('Ctrl Pts',(-0.610938970960348,-0.606308285553778,
-1.04277829918016));
#55212=CARTESIAN_POINT('Ctrl Pts',(-0.253378910006028,-0.822590571742088,
-1.03234433657767));
#55213=CARTESIAN_POINT('Ctrl Pts',(0.163904234062427,-0.844980061330929,
-1.02191037397519));
#55214=CARTESIAN_POINT('Ctrl Pts',(0.542553969616093,-0.668200044521292,
-1.01147641137271));
#55215=CARTESIAN_POINT('Ctrl Pts',(0.793318450980055,-0.333918875136038,
-1.00104244877023));
#55216=CARTESIAN_POINT('Ctrl Pts',(0.857090409214356,0.0790700506594052,
-0.990608486167753));
#55217=CARTESIAN_POINT('Ctrl Pts',(0.718838053513714,0.473421453487905,
-0.980174523565272));
#55218=CARTESIAN_POINT('Ctrl Pts',(0.411148835382887,0.756182953459401,
-0.969740560962792));
#55219=CARTESIAN_POINT('Ctrl Pts',(0.00654795948644188,0.860705030962387,
-0.95930659836031));
#55220=CARTESIAN_POINT('Ctrl Pts',(-0.399596325757388,0.762350837560665,
-0.94887263575783));
#55221=CARTESIAN_POINT('Ctrl Pts',(-0.711552003832334,0.484303387427033,
-0.93843867315535));
#55222=CARTESIAN_POINT('Ctrl Pts',(-0.855788184097906,0.0921010751558536,
-0.928004710552868));
#55223=CARTESIAN_POINT('Ctrl Pts',(-0.798307045430397,-0.321810325775003,
-0.917570747950388));
#55224=CARTESIAN_POINT('Ctrl Pts',(-0.55265743131608,-0.65986800804578,
-0.907136785347908));
#55225=CARTESIAN_POINT('Ctrl Pts',(-0.176741265643775,-0.842388597645019,
-0.896702822745427));
#55226=CARTESIAN_POINT('Ctrl Pts',(0.240834477891071,-0.826350276046739,
-0.886268860142947));
#55227=CARTESIAN_POINT('Ctrl Pts',(0.601643270987137,-0.615533426310559,
-0.875834897540465));
#55228=CARTESIAN_POINT('Ctrl Pts',(0.820639089441999,-0.25962956174058,
-0.865400934937985));
#55229=CARTESIAN_POINT('Ctrl Pts',(0.846202560151337,0.157471431167258,
-0.854966972335505));
#55230=CARTESIAN_POINT('Ctrl Pts',(0.672308132783288,0.537454927447037,
-0.844533009733024));
#55231=CARTESIAN_POINT('Ctrl Pts',(0.33994435853765,0.790755245029512,-0.834099047130543));
#55232=CARTESIAN_POINT('Ctrl Pts',(-0.0725474966321811,0.857667117928168,
-0.823665084528063));
#55233=CARTESIAN_POINT('Ctrl Pts',(-0.467939224870042,0.722418788703158,
-0.813231121925582));
#55234=CARTESIAN_POINT('Ctrl Pts',(-0.753033278981657,0.416889559942566,
-0.802797159323102));
#55235=CARTESIAN_POINT('Ctrl Pts',(-0.860630310410645,0.0130955429679326,
-0.792363196720621));
#55236=CARTESIAN_POINT('Ctrl Pts',(-0.765368687391839,-0.393785216587891,
-0.78192923411814));
#55237=CARTESIAN_POINT('Ctrl Pts',(-0.489702469969954,-0.707847098848631,
-0.771495271515659));
#55238=CARTESIAN_POINT('Ctrl Pts',(-0.0986087769686523,-0.855062765852802,
-0.761061308913179));
#55239=CARTESIAN_POINT('Ctrl Pts',(0.315727931727777,-0.800732100998826,
-0.750627346310698));
#55240=CARTESIAN_POINT('Ctrl Pts',(0.655644598941732,-0.557661352723705,
-0.740193383708218));
#55241=CARTESIAN_POINT('Ctrl Pts',(0.841019670852427,-0.183144581362296,
-0.729759421105738));
#55242=CARTESIAN_POINT('Ctrl Pts',(0.828158500407521,0.234541089461656,
-0.719325458503256));
#55243=CARTESIAN_POINT('Ctrl Pts',(0.620092586381245,0.596943220715433,
-0.708891495900776));
#55244=CARTESIAN_POINT('Ctrl Pts',(0.265865020615963,0.818640223331329,
-0.698457533298295));
#55245=CARTESIAN_POINT('Ctrl Pts',(-0.151029429750584,0.847376029748488,
-0.688023570695815));
#55246=CARTESIAN_POINT('Ctrl Pts',(-0.532324823785285,0.676377340265816,
-0.677589608093333));
#55247=CARTESIAN_POINT('Ctrl Pts',(-0.788146252778425,0.345950153453387,
-0.667155645490855));
#55248=CARTESIAN_POINT('Ctrl Pts',(-0.858194201088189,-0.0660207366037404,
-0.656721682888372));
#55249=CARTESIAN_POINT('Ctrl Pts',(-0.725957708818034,-0.462429918420906,
-0.646287720285893));
#55250=CARTESIAN_POINT('Ctrl Pts',(-0.422606160274217,-0.749840021432158,
-0.635853757683411));
#55251=CARTESIAN_POINT('Ctrl Pts',(-0.0196423670795976,-0.860505782582898,
-0.625419795080932));
#55252=CARTESIAN_POINT('Ctrl Pts',(0.387951316682126,-0.768342241665588,
-0.61498583247845));
#55253=CARTESIAN_POINT('Ctrl Pts',(0.704101228197687,-0.495073211650161,
-0.604551869875971));
#55254=CARTESIAN_POINT('Ctrl Pts',(0.854287861381836,-0.105110771754112,
-0.594117907273489));
#55255=CARTESIAN_POINT('Ctrl Pts',(0.803110814976075,0.309627265129476,
-0.583683944671009));
#55256=CARTESIAN_POINT('Ctrl Pts',(0.562632999903826,0.651383244996612,
-0.573249982068529));
#55257=CARTESIAN_POINT('Ctrl Pts',(0.189537297769378,0.83960207074386,-0.562816019466047));
#55258=CARTESIAN_POINT('Ctrl Pts',(-0.228234127178966,0.829918795807126,
-0.552382056863567));
#55259=CARTESIAN_POINT('Ctrl Pts',(-0.592208622855237,0.624615859115824,
-0.541948094261086));
#55260=CARTESIAN_POINT('Ctrl Pts',(-0.816593979116471,0.272085092781327,
-0.531514131658605));
#55261=CARTESIAN_POINT('Ctrl Pts',(-0.848500458175958,-0.144578687635082,
-0.521080169056126));
#55262=CARTESIAN_POINT('Ctrl Pts',(-0.680407402985169,-0.527163912275939,
-0.510646206453644));
#55263=CARTESIAN_POINT('Ctrl Pts',(-0.351935926797396,-0.785491647232708,
-0.500212243851165));
#55264=CARTESIAN_POINT('Ctrl Pts',(0.0594901556810223,-0.858671616987626,
-0.489778281248683));
#55265=CARTESIAN_POINT('Ctrl Pts',(0.45689384923315,-0.729454614747216,
-0.479344318646203));
#55266=CARTESIAN_POINT('Ctrl Pts',(0.746603367528273,-0.42829830263327,
-0.468910356043722));
#55267=CARTESIAN_POINT('Ctrl Pts',(0.860331453713932,-0.0261880544059605,
-0.458476393441242));
#55268=CARTESIAN_POINT('Ctrl Pts',(0.771271328784714,0.382094964423429,
-0.448042430838761));
#55269=CARTESIAN_POINT('Ctrl Pts',(0.500415301388765,0.700314608286261,
-0.437608468236281));
#55270=CARTESIAN_POINT('Ctrl Pts',(0.111606683342926,0.853463515726458,
-0.427174505633799));
#55271=CARTESIAN_POINT('Ctrl Pts',(-0.303508679116197,0.80544304959721,
-0.41674054303132));
#55272=CARTESIAN_POINT('Ctrl Pts',(-0.647084192799489,0.567572085176711,
-0.406306580428838));
#55273=CARTESIAN_POINT('Ctrl Pts',(-0.838135879378581,0.195919044866881,
-0.395872617826358));
#55274=CARTESIAN_POINT('Ctrl Pts',(-0.831631060361417,-0.221913956041068,
-0.385438655223877));
#55275=CARTESIAN_POINT('Ctrl Pts',(-0.629102982738002,-0.587439751421957,
-0.375004692621397));
#55276=CARTESIAN_POINT('Ctrl Pts',(-0.278289418253274,-0.81450047522273,
-0.364570730018916));
#55277=CARTESIAN_POINT('Ctrl Pts',(0.138119578151266,-0.849575780352192,
-0.354136767416436));
#55278=CARTESIAN_POINT('Ctrl Pts',(0.521972491602115,-0.684398087719615,
-0.343702804813954));
#55279=CARTESIAN_POINT('Ctrl Pts',(0.782791582026743,-0.357901332117912,
-0.333268842211475));
#55280=CARTESIAN_POINT('Ctrl Pts',(0.859099337993372,0.0529561317558256,
-0.322834879608993));
#55281=CARTESIAN_POINT('Ctrl Pts',(0.732909304116489,0.45133133782035,-0.312400917006513));
#55282=CARTESIAN_POINT('Ctrl Pts',(0.433965657579441,0.74332350435601,-0.301966954404032));
#55283=CARTESIAN_POINT('Ctrl Pts',(0.0327322261453245,0.86010733435001,
-0.291532991801552));
#55284=CARTESIAN_POINT('Ctrl Pts',(-0.376216498791165,0.774155778332482,
-0.281099029199071));
#55285=CARTESIAN_POINT('Ctrl Pts',(-0.696487458167504,0.505728431782088,
-0.270665066596591));
#55286=CARTESIAN_POINT('Ctrl Pts',(-0.852589776780192,0.118096132321047,
-0.26023110399411));
#55287=CARTESIAN_POINT('Ctrl Pts',(-0.807728669522175,-0.297372520979868,
-0.249797141391629));
#55288=CARTESIAN_POINT('Ctrl Pts',(-0.572478323412175,-0.64274770454798,
-0.239363178789149));
#55289=CARTESIAN_POINT('Ctrl Pts',(-0.202289451911256,-0.836621155292499,
-0.228929216186668));
#55290=CARTESIAN_POINT('Ctrl Pts',(0.215580939060973,-0.833295246691126,
-0.218495253584188));
#55291=CARTESIAN_POINT('Ctrl Pts',(0.582636887836437,-0.633553595935407,
-0.208061290981707));
#55292=CARTESIAN_POINT('Ctrl Pts',(0.812359822146789,-0.284477837654277,
-0.197627328379227));
#55293=CARTESIAN_POINT('Ctrl Pts',(0.850601954996978,0.131652867513664,
-0.187193365776746));
#55294=CARTESIAN_POINT('Ctrl Pts',(0.688349122337913,0.51675009114103,-0.176759403174265));
#55295=CARTESIAN_POINT('Ctrl Pts',(0.363846105084824,0.780047728610944,
-0.166325440571784));
#55296=CARTESIAN_POINT('Ctrl Pts',(-0.0464192020363373,0.859474361780549,
-0.155891477969304));
#55297=CARTESIAN_POINT('Ctrl Pts',(-0.445742392858137,0.736327430271739,
-0.145457515366823));
#55298=CARTESIAN_POINT('Ctrl Pts',(-0.740001245121636,0.439596369442942,
-0.135023552764343));
#55299=CARTESIAN_POINT('Ctrl Pts',(-0.859832124525603,0.0392974457347477,
-0.124589590161862));
#55300=CARTESIAN_POINT('Ctrl Pts',(-0.776998977184778,-0.370364573784881,
-0.114155627559381));
#55301=CARTESIAN_POINT('Ctrl Pts',(-0.599661254481017,-0.585112006191819,
-0.107199652491061));
#55302=CARTESIAN_POINT('Ctrl Pts',(-0.490897892427236,-0.665357183556695,
-0.103721664956901));
#55303=CARTESIAN_POINT('Ctrl Pts',(0.82685,-1.18395083925468E-14,-1.12910983122651));
#55304=CARTESIAN_POINT('Ctrl Pts',(0.826850000000002,0.13516238059478,-1.12563184369235));
#55305=CARTESIAN_POINT('Ctrl Pts',(0.759329891769109,0.405358236621008,
-1.11867586862402));
#55306=CARTESIAN_POINT('Ctrl Pts',(0.478857042724253,0.715228435638399,
-1.10824190602155));
#55307=CARTESIAN_POINT('Ctrl Pts',(0.0855976953161874,0.85645769610236,
-1.09780794341906));
#55308=CARTESIAN_POINT('Ctrl Pts',(-0.327879002777259,0.795839066043269,
-1.08737398081658));
#55309=CARTESIAN_POINT('Ctrl Pts',(-0.664050756097952,0.547619885902207,
-1.0769400182141));
#55310=CARTESIAN_POINT('Ctrl Pts',(-0.84371006453472,0.170328568685808,
-1.06650605561162));
#55311=CARTESIAN_POINT('Ctrl Pts',(-0.824493606532929,-0.247114364257438,
-1.05607209300914));
#55312=CARTESIAN_POINT('Ctrl Pts',(-0.610938989097409,-0.606308301358728,
-1.04563813040666));
#55313=CARTESIAN_POINT('Ctrl Pts',(-0.253378917416567,-0.8225905970557,
-1.03520416780418));
#55314=CARTESIAN_POINT('Ctrl Pts',(0.163904238864593,-0.844980085711621,
-1.0247702052017));
#55315=CARTESIAN_POINT('Ctrl Pts',(0.542553985631643,-0.668200064499605,
-1.01433624259922));
#55316=CARTESIAN_POINT('Ctrl Pts',(0.793318474366497,-0.333918884843972,
-1.00390227999674));
#55317=CARTESIAN_POINT('Ctrl Pts',(0.857090434493622,0.0790700529203221,
-0.993468317394257));
#55318=CARTESIAN_POINT('Ctrl Pts',(0.718838074709771,0.473421467484893,
-0.983034354791779));
#55319=CARTESIAN_POINT('Ctrl Pts',(0.411148847508517,0.756182975740498,
-0.972600392189296));
#55320=CARTESIAN_POINT('Ctrl Pts',(0.00654795967899482,0.860705056353458,
-0.962166429586817));
#55321=CARTESIAN_POINT('Ctrl Pts',(-0.399596337540997,0.76235086003724,
-0.951732466984335));
#55322=CARTESIAN_POINT('Ctrl Pts',(-0.711552024815767,0.484303401711301,
-0.941298504381855));
#55323=CARTESIAN_POINT('Ctrl Pts',(-0.855788209334577,0.0921010778706362,
-0.930864541779374));
#55324=CARTESIAN_POINT('Ctrl Pts',(-0.798307068972087,-0.321810335264394,
-0.920430579176894));
#55325=CARTESIAN_POINT('Ctrl Pts',(-0.552657447613637,-0.659868027505257,
-0.909996616574414));
#55326=CARTESIAN_POINT('Ctrl Pts',(-0.176741270855791,-0.842388622486454,
-0.899562653971932));
#55327=CARTESIAN_POINT('Ctrl Pts',(0.240834484993158,-0.826350300415455,
-0.889128691369453));
#55328=CARTESIAN_POINT('Ctrl Pts',(0.601643288729277,-0.615533444462273,
-0.878694728766971));
#55329=CARTESIAN_POINT('Ctrl Pts',(0.820639113642215,-0.25962956939694,
-0.868260766164491));
#55330=CARTESIAN_POINT('Ctrl Pts',(0.846202585105403,0.157471435811019,
-0.857826803562011));
#55331=CARTESIAN_POINT('Ctrl Pts',(0.672308152609301,0.537454943296294,
-0.847392840959529));
#55332=CARTESIAN_POINT('Ctrl Pts',(0.33994436856243,0.79075526834847,-0.83695887835705));
#55333=CARTESIAN_POINT('Ctrl Pts',(-0.0725474987715683,0.857667143220317,
-0.826524915754568));
#55334=CARTESIAN_POINT('Ctrl Pts',(-0.467939238669323,0.722418810006908,
-0.816090953152088));
#55335=CARTESIAN_POINT('Ctrl Pts',(-0.753033301188211,0.416889572236419,
-0.805656990549607));
#55336=CARTESIAN_POINT('Ctrl Pts',(-0.86063033579018,0.0130955433541141,
-0.795223027947127));
#55337=CARTESIAN_POINT('Ctrl Pts',(-0.765368709962157,-0.393785228200411,
-0.784789065344645));
#55338=CARTESIAN_POINT('Ctrl Pts',(-0.489702484411022,-0.707847119722667,
-0.774355102742166));
#55339=CARTESIAN_POINT('Ctrl Pts',(-0.0986087798765727,-0.855062791068153,
-0.763921140139684));
#55340=CARTESIAN_POINT('Ctrl Pts',(0.315727941038427,-0.800732124611992,
-0.753487177537205));
#55341=CARTESIAN_POINT('Ctrl Pts',(0.655644618276346,-0.557661369168844,
-0.743053214934723));
#55342=CARTESIAN_POINT('Ctrl Pts',(0.841019695653654,-0.183144586763133,
-0.732619252332244));
#55343=CARTESIAN_POINT('Ctrl Pts',(0.828158524829477,0.23454109637815,-0.722185289729761));
#55344=CARTESIAN_POINT('Ctrl Pts',(0.620092604667449,0.596943238318974,
-0.711751327127283));
#55345=CARTESIAN_POINT('Ctrl Pts',(0.265865028456182,0.818640247472597,
-0.7013173645248));
#55346=CARTESIAN_POINT('Ctrl Pts',(-0.151029434204362,0.84737605473716,
-0.690883401922322));
#55347=CARTESIAN_POINT('Ctrl Pts',(-0.532324839483263,0.676377360211827,
-0.680449439319839));
#55348=CARTESIAN_POINT('Ctrl Pts',(-0.788146276020443,0.345950163655275,
-0.670015476717359));
#55349=CARTESIAN_POINT('Ctrl Pts',(-0.858194226395883,-0.0660207385506573,
-0.659581514114879));
#55350=CARTESIAN_POINT('Ctrl Pts',(-0.725957730226144,-0.46242993205772,
-0.649147551512397));
#55351=CARTESIAN_POINT('Ctrl Pts',(-0.42260617273665,-0.749840043544545,
-0.638713588909918));
#55352=CARTESIAN_POINT('Ctrl Pts',(-0.0196423676588402,-0.860505807958759,
-0.628279626307437));
#55353=CARTESIAN_POINT('Ctrl Pts',(0.387951328122605,-0.768342264323595,
-0.617845663704956));
#55354=CARTESIAN_POINT('Ctrl Pts',(0.704101248961261,-0.495073226249609,
-0.607411701102476));
#55355=CARTESIAN_POINT('Ctrl Pts',(0.854287886574333,-0.105110774853773,
-0.596977738499995));
#55356=CARTESIAN_POINT('Ctrl Pts',(0.803110838659391,0.309627274260221,
-0.586543775897515));
#55357=CARTESIAN_POINT('Ctrl Pts',(0.562633016495577,0.65138326420556,-0.576109813295034));
#55358=CARTESIAN_POINT('Ctrl Pts',(0.189537303358733,0.839602095503282,
-0.565675850692553));
#55359=CARTESIAN_POINT('Ctrl Pts',(-0.228234133909469,0.829918820280995,
-0.555241888090073));
#55360=CARTESIAN_POINT('Ctrl Pts',(-0.592208640319157,0.624615877535415,
-0.544807925487591));
#55361=CARTESIAN_POINT('Ctrl Pts',(-0.816594003197397,0.272085100804974,
-0.534373962885112));
#55362=CARTESIAN_POINT('Ctrl Pts',(-0.848500483197789,-0.144578691898632,
-0.523940000282631));
#55363=CARTESIAN_POINT('Ctrl Pts',(-0.680407423050025,-0.527163927821724,
-0.51350603768015));
#55364=CARTESIAN_POINT('Ctrl Pts',(-0.351935937175801,-0.785491670396442,
-0.50307207507767));
#55365=CARTESIAN_POINT('Ctrl Pts',(0.0594901574353561,-0.858671642309399,
-0.492638112475189));
#55366=CARTESIAN_POINT('Ctrl Pts',(0.456893862706708,-0.729454636258447,
-0.482204149872708));
#55367=CARTESIAN_POINT('Ctrl Pts',(0.746603389545214,-0.428298315263561,
-0.471770187270228));
#55368=CARTESIAN_POINT('Ctrl Pts',(0.860331479084652,-0.0261880551782322,
-0.461336224667747));
#55369=CARTESIAN_POINT('Ctrl Pts',(0.771271351529099,0.382094975691208,
-0.450902262065267));
#55370=CARTESIAN_POINT('Ctrl Pts',(0.500415316145748,0.700314628938169,
-0.440468299462786));
#55371=CARTESIAN_POINT('Ctrl Pts',(0.111606686634148,0.853463540894647,
-0.430034336860305));
#55372=CARTESIAN_POINT('Ctrl Pts',(-0.303508688066508,0.805443073349301,
-0.419600374257825));
#55373=CARTESIAN_POINT('Ctrl Pts',(-0.64708421188166,0.567572101914111,
-0.409166411655344));
#55374=CARTESIAN_POINT('Ctrl Pts',(-0.838135904094767,0.195919050644432,
-0.398732449052864));
#55375=CARTESIAN_POINT('Ctrl Pts',(-0.831631084885775,-0.221913962585196,
-0.388298486450383));
#55376=CARTESIAN_POINT('Ctrl Pts',(-0.629103001289925,-0.587439768745239,
-0.377864523847903));
#55377=CARTESIAN_POINT('Ctrl Pts',(-0.278289426459866,-0.814500499241933,
-0.367430561245421));
#55378=CARTESIAN_POINT('Ctrl Pts',(0.138119582224307,-0.849575805405707,
-0.356996598642941));
#55379=CARTESIAN_POINT('Ctrl Pts',(0.521972506994872,-0.684398107902206,
-0.346562636040461));
#55380=CARTESIAN_POINT('Ctrl Pts',(0.78279160511073,-0.35790134267213,-0.336128673437979));
#55381=CARTESIAN_POINT('Ctrl Pts',(0.859099363328004,0.0529561333172702,
-0.3256947108355));
#55382=CARTESIAN_POINT('Ctrl Pts',(0.732909325729115,0.451331351130274,
-0.315260748233019));
#55383=CARTESIAN_POINT('Ctrl Pts',(0.433965670377806,0.743323526275441,
-0.304826785630538));
#55384=CARTESIAN_POINT('Ctrl Pts',(0.032732227108719,0.86010735971567,-0.294392823028057));
#55385=CARTESIAN_POINT('Ctrl Pts',(-0.376216509881933,0.774155801158885,
-0.283958860425577));
#55386=CARTESIAN_POINT('Ctrl Pts',(-0.696487478713739,0.505728446701731,
-0.273524897823096));
#55387=CARTESIAN_POINT('Ctrl Pts',(-0.85258980190849,0.118096135791892,
-0.263090935220616));
#55388=CARTESIAN_POINT('Ctrl Pts',(-0.807728693369422,-0.297372529726142,
-0.252656972618135));
#55389=CARTESIAN_POINT('Ctrl Pts',(-0.57247834023972,-0.642747723547633,
-0.242223010015654));
#55390=CARTESIAN_POINT('Ctrl Pts',(-0.202289457983834,-0.836621179874879,
-0.231789047413174));
#55391=CARTESIAN_POINT('Ctrl Pts',(0.215580945628928,-0.833295271439718,
-0.221355084810693));
#55392=CARTESIAN_POINT('Ctrl Pts',(0.582636904604284,-0.633553614274387,
-0.210921122208213));
#55393=CARTESIAN_POINT('Ctrl Pts',(0.812359846915988,-0.2844778467197,-0.200487159605732));
#55394=CARTESIAN_POINT('Ctrl Pts',(0.850601978482956,0.131652872725018,
-0.190053197003252));
#55395=CARTESIAN_POINT('Ctrl Pts',(0.688349145776723,0.516750103768243,
-0.179619234400771));
#55396=CARTESIAN_POINT('Ctrl Pts',(0.363846109644695,0.780047756745801,
-0.16918527179829));
#55397=CARTESIAN_POINT('Ctrl Pts',(-0.0464191912805547,0.85947437704138,
-0.15875130919581));
#55398=CARTESIAN_POINT('Ctrl Pts',(-0.445742429839068,0.736327471811283,
-0.148317346593329));
#55399=CARTESIAN_POINT('Ctrl Pts',(-0.740001219981211,0.439596343345489,
-0.137883383990848));
#55400=CARTESIAN_POINT('Ctrl Pts',(-0.859832243554816,0.0392975248057425,
-0.127449421388368));
#55401=CARTESIAN_POINT('Ctrl Pts',(-0.776998800479074,-0.370364750731842,
-0.117015458785887));
#55402=CARTESIAN_POINT('Ctrl Pts',(-0.599661587021621,-0.58511176084468,
-0.110059483717567));
#55403=CARTESIAN_POINT('Ctrl Pts',(-0.490897892427236,-0.665357183556695,
-0.106581496183407));
#55404=CARTESIAN_POINT('Ctrl Pts',(0.825266255435535,-1.18168310543808E-14,
-1.13578682154469));
#55405=CARTESIAN_POINT('Ctrl Pts',(0.825266255435537,0.13490237313339,-1.13230883401053));
#55406=CARTESIAN_POINT('Ctrl Pts',(0.757875373501364,0.404582484316022,
-1.12535285894221));
#55407=CARTESIAN_POINT('Ctrl Pts',(0.477939823171883,0.7138581043365,-1.11491889633972));
#55408=CARTESIAN_POINT('Ctrl Pts',(0.0854337254619297,0.854817337751033,
-1.10448493373724));
#55409=CARTESIAN_POINT('Ctrl Pts',(-0.327250953856651,0.794314572438201,
-1.09405097113476));
#55410=CARTESIAN_POINT('Ctrl Pts',(-0.662778785930788,0.54657097627622,
-1.08361700853228));
#55411=CARTESIAN_POINT('Ctrl Pts',(-0.842093957705063,0.170002286889046,
-1.0731830459298));
#55412=CARTESIAN_POINT('Ctrl Pts',(-0.822914310253027,-0.246641011830828,
-1.06274908332732));
#55413=CARTESIAN_POINT('Ctrl Pts',(-0.609768750387392,-0.605146938555674,
-1.05231512072484));
#55414=CARTESIAN_POINT('Ctrl Pts',(-0.252893576591479,-0.821014942444095,
-1.04188115812236));
#55415=CARTESIAN_POINT('Ctrl Pts',(0.163590284471105,-0.843361548903805,
-1.03144719551988));
#55416=CARTESIAN_POINT('Ctrl Pts',(0.541514736972462,-0.666920143216012,
-1.0210132329174));
#55417=CARTESIAN_POINT('Ctrl Pts',(0.791798892653782,-0.333279271931917,
-1.01057927031492));
#55418=CARTESIAN_POINT('Ctrl Pts',(0.855448699150102,0.0789185963993196,
-1.00014530771244));
#55419=CARTESIAN_POINT('Ctrl Pts',(0.717461158327158,0.472514640384086,
-0.989711345109958));
#55420=CARTESIAN_POINT('Ctrl Pts',(0.410361302151426,0.754734526176116,
-0.979277382507477));
#55421=CARTESIAN_POINT('Ctrl Pts',(0.00653541722715152,0.859056397277897,
-0.968843419904996));
#55422=CARTESIAN_POINT('Ctrl Pts',(-0.398830920732009,0.760890596007683,
-0.958409457302515));
#55423=CARTESIAN_POINT('Ctrl Pts',(-0.710189064673792,0.483375730628087,
-0.947975494700036));
#55424=CARTESIAN_POINT('Ctrl Pts',(-0.854148968382191,0.0919246605583529,
-0.937541532097554));
#55425=CARTESIAN_POINT('Ctrl Pts',(-0.796777931708914,-0.321193915601999,
-0.927107569495075));
#55426=CARTESIAN_POINT('Ctrl Pts',(-0.551598846068358,-0.658604066769501,
-0.916673606892592));
#55427=CARTESIAN_POINT('Ctrl Pts',(-0.176402727363301,-0.840775048108436,
-0.906239644290114));
#55428=CARTESIAN_POINT('Ctrl Pts',(0.240373172548911,-0.824767447042349,
-0.895805681687632));
#55429=CARTESIAN_POINT('Ctrl Pts',(0.600490856028094,-0.61435440551462,
-0.885371719085151));
#55430=CARTESIAN_POINT('Ctrl Pts',(0.819067199905029,-0.259132255437641,
-0.874937756482671));
#55431=CARTESIAN_POINT('Ctrl Pts',(0.844581705176757,0.157169803206534,
-0.86450379388019));
#55432=CARTESIAN_POINT('Ctrl Pts',(0.671020363125302,0.53642546176851,-0.854069831277709));
#55433=CARTESIAN_POINT('Ctrl Pts',(0.339293213610226,0.789240596370972,
-0.84363586867523));
#55434=CARTESIAN_POINT('Ctrl Pts',(-0.0724085358486207,0.856024303216785,
-0.833201906072748));
#55435=CARTESIAN_POINT('Ctrl Pts',(-0.467042912738468,0.721035034809539,
-0.822767943470269));
#55436=CARTESIAN_POINT('Ctrl Pts',(-0.751590884697192,0.416091030667303,
-0.812333980867787));
#55437=CARTESIAN_POINT('Ctrl Pts',(-0.858981819865244,0.013070459167713,
-0.801900018265307));
#55438=CARTESIAN_POINT('Ctrl Pts',(-0.763902665303551,-0.393030942425558,
-0.791466055662826));
#55439=CARTESIAN_POINT('Ctrl Pts',(-0.488764471526209,-0.706491256234298,
-0.781032093060345));
#55440=CARTESIAN_POINT('Ctrl Pts',(-0.0984198972202164,-0.853424939636153,
-0.770598130457865));
#55441=CARTESIAN_POINT('Ctrl Pts',(0.315123172048648,-0.799198342215375,
-0.760164167855384));
#55442=CARTESIAN_POINT('Ctrl Pts',(0.654388747376403,-0.556593182736684,
-0.749730205252904));
#55443=CARTESIAN_POINT('Ctrl Pts',(0.839408743420374,-0.182793777878889,
-0.739296242650423));
#55444=CARTESIAN_POINT('Ctrl Pts',(0.826572207847868,0.234091838762711,
-0.728862280047942));
#55445=CARTESIAN_POINT('Ctrl Pts',(0.618904832762115,0.595799808447021,
-0.718428317445462));
#55446=CARTESIAN_POINT('Ctrl Pts',(0.265355770630764,0.817072162513667,
-0.70799435484298));
#55447=CARTESIAN_POINT('Ctrl Pts',(-0.150740141093178,0.845752927056724,
-0.697560392240501));
#55448=CARTESIAN_POINT('Ctrl Pts',(-0.531305184541259,0.675081776262244,
-0.687126429638019));
#55449=CARTESIAN_POINT('Ctrl Pts',(-0.786636601502631,0.345287504752488,
-0.67669246703554));
#55450=CARTESIAN_POINT('Ctrl Pts',(-0.856550376777681,-0.0658942774739896,
-0.666258504433059));
#55451=CARTESIAN_POINT('Ctrl Pts',(-0.724567176315435,-0.461544159066156,
-0.655824541830578));
#55452=CARTESIAN_POINT('Ctrl Pts',(-0.421796681161974,-0.74840374365883,
-0.645390579228098));
#55453=CARTESIAN_POINT('Ctrl Pts',(-0.0196047431939077,-0.858857530563777,
-0.634956616625617));
#55454=CARTESIAN_POINT('Ctrl Pts',(0.387208217037725,-0.766870523895835,
-0.624522654023137));
#55455=CARTESIAN_POINT('Ctrl Pts',(0.702752560594827,-0.49412492584287,
-0.614088691420656));
#55456=CARTESIAN_POINT('Ctrl Pts',(0.85265151945255,-0.104909437788342,
-0.603654728818175));
#55457=CARTESIAN_POINT('Ctrl Pts',(0.801572499895392,0.309034190945369,
-0.593220766215695));
#55458=CARTESIAN_POINT('Ctrl Pts',(0.561555306997066,0.650135555822967,
-0.582786803613214));
#55459=CARTESIAN_POINT('Ctrl Pts',(0.189174249385427,0.837993858647704,
-0.572352841010733));
#55460=CARTESIAN_POINT('Ctrl Pts',(-0.227796957123204,0.828329131497389,
-0.561918878408252));
#55461=CARTESIAN_POINT('Ctrl Pts',(-0.591074279451486,0.623419441413815,
-0.551484915805773));
#55462=CARTESIAN_POINT('Ctrl Pts',(-0.815029837768297,0.271563928586238,
-0.541050953203291));
#55463=CARTESIAN_POINT('Ctrl Pts',(-0.846875201702706,-0.144301755023309,
-0.530616990600811));
#55464=CARTESIAN_POINT('Ctrl Pts',(-0.679104119615673,-0.52615415847718,
-0.52018302799833));
#55465=CARTESIAN_POINT('Ctrl Pts',(-0.351261812673254,-0.783987080709438,
-0.50974906539585));
#55466=CARTESIAN_POINT('Ctrl Pts',(0.0593762055237972,-0.857026878212933,
-0.499315102793369));
#55467=CARTESIAN_POINT('Ctrl Pts',(0.456018693917792,-0.728057384111524,
-0.488881140190888));
#55468=CARTESIAN_POINT('Ctrl Pts',(0.745173289389441,-0.427477920531964,
-0.478447177588408));
#55469=CARTESIAN_POINT('Ctrl Pts',(0.858683535612276,-0.0261378926122512,
-0.468013214985927));
#55470=CARTESIAN_POINT('Ctrl Pts',(0.769794000507914,0.381363082303222,
-0.457579252383447));
#55471=CARTESIAN_POINT('Ctrl Pts',(0.499456783099164,0.698973193747868,
-0.447145289780966));
#55472=CARTESIAN_POINT('Ctrl Pts',(0.111392906811854,0.851828752786435,
-0.436711327178485));
#55473=CARTESIAN_POINT('Ctrl Pts',(-0.302927324750776,0.803900267247972,
-0.426277364576005));
#55474=CARTESIAN_POINT('Ctrl Pts',(-0.645844738226482,0.566484931720774,
-0.415843401973524));
#55475=CARTESIAN_POINT('Ctrl Pts',(-0.836530475692227,0.195543772593499,
-0.405409439371044));
#55476=CARTESIAN_POINT('Ctrl Pts',(-0.830038116302071,-0.221488891929327,
-0.394975476768563));
#55477=CARTESIAN_POINT('Ctrl Pts',(-0.627897970194759,-0.586314542532045,
-0.384541514166082));
#55478=CARTESIAN_POINT('Ctrl Pts',(-0.277756370010257,-0.812940343867364,
-0.374107551563602));
#55479=CARTESIAN_POINT('Ctrl Pts',(0.137855017612419,-0.84794846415785,
-0.363673588961121));
#55480=CARTESIAN_POINT('Ctrl Pts',(0.52097268168716,-0.683087160410494,
-0.353239626358641));
#55481=CARTESIAN_POINT('Ctrl Pts',(0.781292187331718,-0.357215791584545,
-0.34280566375616));
#55482=CARTESIAN_POINT('Ctrl Pts',(0.85745377994194,0.0528546971663574,
-0.33237170115368));
#55483=CARTESIAN_POINT('Ctrl Pts',(0.731505456212053,0.450466837192345,
-0.321937738551198));
#55484=CARTESIAN_POINT('Ctrl Pts',(0.433134419966394,0.741899708618021,
-0.311503775948719));
#55485=CARTESIAN_POINT('Ctrl Pts',(0.0326695293497987,0.85845984553416,
-0.301069813346238));
#55486=CARTESIAN_POINT('Ctrl Pts',(-0.375495876558362,0.772672925054669,
-0.290635850743757));
#55487=CARTESIAN_POINT('Ctrl Pts',(-0.695153374314712,0.504759736470019,
-0.280201888141276));
#55488=CARTESIAN_POINT('Ctrl Pts',(-0.850956687463709,0.117869925623513,
-0.269767925538796));
#55489=CARTESIAN_POINT('Ctrl Pts',(-0.806181509144908,-0.296802920130996,
-0.259333962936315));
#55490=CARTESIAN_POINT('Ctrl Pts',(-0.571381772416895,-0.641516556204879,
-0.248900000333835));
#55491=CARTESIAN_POINT('Ctrl Pts',(-0.201901977286717,-0.83501865312994,
-0.238466037731354));
#55492=CARTESIAN_POINT('Ctrl Pts',(0.215168005139208,-0.831699114674313,
-0.228032075128874));
#55493=CARTESIAN_POINT('Ctrl Pts',(0.581520879277018,-0.632340059072367,
-0.217598112526393));
#55494=CARTESIAN_POINT('Ctrl Pts',(0.810803789707571,-0.283932934675695,
-0.207164149923912));
#55495=CARTESIAN_POINT('Ctrl Pts',(0.84897267594911,0.131400691338038,-0.196730187321431));
#55496=CARTESIAN_POINT('Ctrl Pts',(0.687030621675953,0.515760288909202,
-0.186296224718951));
#55497=CARTESIAN_POINT('Ctrl Pts',(0.363149188196698,0.778553580855524,
-0.175862262116471));
#55498=CARTESIAN_POINT('Ctrl Pts',(-0.0463303092822942,0.857828102611029,
-0.16542829951399));
#55499=CARTESIAN_POINT('Ctrl Pts',(-0.444888556851283,0.734917001280111,
-0.154994336911509));
#55500=CARTESIAN_POINT('Ctrl Pts',(-0.738583893176423,0.438754413204503,
-0.144560374309029));
#55501=CARTESIAN_POINT('Ctrl Pts',(-0.858185002917794,0.0392220405825323,
-0.134126411706548));
#55502=CARTESIAN_POINT('Ctrl Pts',(-0.77551101875214,-0.369654877107249,
-0.123692449104067));
#55503=CARTESIAN_POINT('Ctrl Pts',(-0.598512098358559,-0.583991704355505,
-0.116736474035747));
#55504=CARTESIAN_POINT('Ctrl Pts',(-0.489957628934657,-0.664082761566146,
-0.113258486501587));
#55505=CARTESIAN_POINT('Ctrl Pts',(0.82035433218061,-1.17464981565151E-14,
-1.14076763757253));
#55506=CARTESIAN_POINT('Ctrl Pts',(0.820354332180612,0.134101768298544,
-1.13728965003837));
#55507=CARTESIAN_POINT('Ctrl Pts',(0.753364766519594,0.402173049067142,
-1.13033367497005));
#55508=CARTESIAN_POINT('Ctrl Pts',(0.475095200548904,0.709610076749487,
-1.11989971236757));
#55509=CARTESIAN_POINT('Ctrl Pts',(0.0849252644561764,0.849729327752102,
-1.10946574976509));
#55510=CARTESIAN_POINT('Ctrl Pts',(-0.325303245075429,0.789587177339037,
-1.09903178716261));
#55511=CARTESIAN_POINT('Ctrl Pts',(-0.658834080958521,0.543317828833928,
-1.08859782456013));
#55512=CARTESIAN_POINT('Ctrl Pts',(-0.837082019765518,0.168990519247415,
-1.07816386195765));
#55513=CARTESIAN_POINT('Ctrl Pts',(-0.818016521001053,-0.245173086817304,
-1.06772989935517));
#55514=CARTESIAN_POINT('Ctrl Pts',(-0.606139554222435,-0.601545237955094,
-1.05729593675269));
#55515=CARTESIAN_POINT('Ctrl Pts',(-0.251388414543869,-0.816128465044896,
-1.04686197415021));
#55516=CARTESIAN_POINT('Ctrl Pts',(0.162616634294616,-0.838342060921673,
-1.03642801154773));
#55517=CARTESIAN_POINT('Ctrl Pts',(0.538291771678315,-0.662950796574508,
-1.02599404894525));
#55518=CARTESIAN_POINT('Ctrl Pts',(0.787086296167862,-0.331295673135843,
-1.01556008634276));
#55519=CARTESIAN_POINT('Ctrl Pts',(0.850357274403785,0.0784488915092764,
-1.00512612374029));
#55520=CARTESIAN_POINT('Ctrl Pts',(0.713191002178242,0.469702347171158,
-0.994692161137803));
#55521=CARTESIAN_POINT('Ctrl Pts',(0.407918930452038,0.750242527821308,
-0.984258198535323));
#55522=CARTESIAN_POINT('Ctrl Pts',(0.00649651999369233,0.853943500409919,
-0.973824235932843));
#55523=CARTESIAN_POINT('Ctrl Pts',(-0.396457175080158,0.756361958283298,
-0.963390273330362));
#55524=CARTESIAN_POINT('Ctrl Pts',(-0.705962190288657,0.480498794630974,
-0.952956310727882));
#55525=CARTESIAN_POINT('Ctrl Pts',(-0.849065279296998,0.0913775470960521,
-0.9425223481254));
#55526=CARTESIAN_POINT('Ctrl Pts',(-0.792035701226651,-0.319282246717183,
-0.932088385522921));
#55527=CARTESIAN_POINT('Ctrl Pts',(-0.548315862494261,-0.654684213877508,
-0.92165442292044));
#55528=CARTESIAN_POINT('Ctrl Pts',(-0.175352820786375,-0.835770957377393,
-0.911220460317959));
#55529=CARTESIAN_POINT('Ctrl Pts',(0.238942529278504,-0.819858629701546,
-0.900786497715479));
#55530=CARTESIAN_POINT('Ctrl Pts',(0.596916878978049,-0.610697915954462,
-0.890352535112997));
#55531=CARTESIAN_POINT('Ctrl Pts',(0.814192309062805,-0.257589962620876,
-0.879918572510518));
#55532=CARTESIAN_POINT('Ctrl Pts',(0.83955495813993,0.156234366365253,-0.869484609908036));
#55533=CARTESIAN_POINT('Ctrl Pts',(0.667026611423942,0.533232786525937,
-0.859050647305557));
#55534=CARTESIAN_POINT('Ctrl Pts',(0.33727382206329,0.784543226294379,-0.848616684703075));
#55535=CARTESIAN_POINT('Ctrl Pts',(-0.0719775776704039,0.850929452590404,
-0.838182722100595));
#55536=CARTESIAN_POINT('Ctrl Pts',(-0.464263185728888,0.716743607819756,
-0.827748759498115));
#55537=CARTESIAN_POINT('Ctrl Pts',(-0.747117596643002,0.413614556996802,
-0.817314796895633));
#55538=CARTESIAN_POINT('Ctrl Pts',(-0.853869366811588,0.012992666940522,
-0.806880834293153));
#55539=CARTESIAN_POINT('Ctrl Pts',(-0.759356100494369,-0.390691716850214,
-0.796446871690672));
#55540=CARTESIAN_POINT('Ctrl Pts',(-0.485855463026629,-0.70228639031422,
-0.786012909088192));
#55541=CARTESIAN_POINT('Ctrl Pts',(-0.0978341256794837,-0.848345559796202,
-0.775578946485711));
#55542=CARTESIAN_POINT('Ctrl Pts',(0.313247634771886,-0.794441706032112,
-0.765144983883231));
#55543=CARTESIAN_POINT('Ctrl Pts',(0.650493983049112,-0.553280474072871,
-0.754711021280749));
#55544=CARTESIAN_POINT('Ctrl Pts',(0.834412784606905,-0.181705833307428,
-0.74427705867827));
#55545=CARTESIAN_POINT('Ctrl Pts',(0.821652649004654,0.232698580479193,
-0.733843096075788));
#55546=CARTESIAN_POINT('Ctrl Pts',(0.615221260154405,0.592253751383159,
-0.723409133473309));
#55547=CARTESIAN_POINT('Ctrl Pts',(0.263776436949314,0.812209145653827,
-0.712975170870827));
#55548=CARTESIAN_POINT('Ctrl Pts',(-0.149842972053255,0.84071920918916,
-0.702541208268347));
#55549=CARTESIAN_POINT('Ctrl Pts',(-0.528142983956435,0.671063852007384,
-0.692107245665866));
#55550=CARTESIAN_POINT('Ctrl Pts',(-0.781954729776754,0.34323243662737,
-0.681673283063386));
#55551=CARTESIAN_POINT('Ctrl Pts',(-0.851452395088088,-0.0655020905937791,
-0.671239320460906));
#55552=CARTESIAN_POINT('Ctrl Pts',(-0.720254726869515,-0.458797159315003,
-0.660805357858424));
#55553=CARTESIAN_POINT('Ctrl Pts',(-0.419286248832957,-0.743949424701024,
-0.650371395255944));
#55554=CARTESIAN_POINT('Ctrl Pts',(-0.0194880604808514,-0.85374581725013,
-0.639937432653463));
#55555=CARTESIAN_POINT('Ctrl Pts',(0.384903646922486,-0.76230629510661,
-0.629503470050983));
#55556=CARTESIAN_POINT('Ctrl Pts',(0.698569946491375,-0.491184013209342,
-0.619069507448502));
#55557=CARTESIAN_POINT('Ctrl Pts',(0.847576742823385,-0.104285042064039,
-0.608635544846021));
#55558=CARTESIAN_POINT('Ctrl Pts',(0.796801733297026,0.307194893818649,
-0.598201582243541));
#55559=CARTESIAN_POINT('Ctrl Pts',(0.55821306496393,0.646266105468152,-0.58776761964106));
#55560=CARTESIAN_POINT('Ctrl Pts',(0.188048329783199,0.833006320887871,
-0.577333657038579));
#55561=CARTESIAN_POINT('Ctrl Pts',(-0.226441164460163,0.823399115867464,
-0.566899694436099));
#55562=CARTESIAN_POINT('Ctrl Pts',(-0.587556347598874,0.619708998941978,
-0.556465731833618));
#55563=CARTESIAN_POINT('Ctrl Pts',(-0.810178976333799,0.269947645442805,
-0.546031769231138));
#55564=CARTESIAN_POINT('Ctrl Pts',(-0.841834804326554,-0.143442905707695,
-0.535597806628657));
#55565=CARTESIAN_POINT('Ctrl Pts',(-0.675062255341266,-0.52302261555975,
-0.525163844026177));
#55566=CARTESIAN_POINT('Ctrl Pts',(-0.349171186905277,-0.779320978293641,
-0.514729881423696));
#55567=CARTESIAN_POINT('Ctrl Pts',(0.0590228126390766,-0.851926060501479,
-0.504295918821215));
#55568=CARTESIAN_POINT('Ctrl Pts',(0.453304580405343,-0.723724161788819,
-0.493861956218735));
#55569=CARTESIAN_POINT('Ctrl Pts',(0.740738197317948,-0.424933674833566,
-0.483427993616254));
#55570=CARTESIAN_POINT('Ctrl Pts',(0.853572857874703,-0.0259823261662435,
-0.472994031013774));
#55571=CARTESIAN_POINT('Ctrl Pts',(0.765212371889512,0.379093301023127,
-0.462560068411293));
#55572=CARTESIAN_POINT('Ctrl Pts',(0.496484136534507,0.694813073526278,
-0.452126105808813));
#55573=CARTESIAN_POINT('Ctrl Pts',(0.110729923040354,0.846758873066444,
-0.441692143206331));
#55574=CARTESIAN_POINT('Ctrl Pts',(-0.30112437422186,0.799115646338569,
-0.431258180603851));
#55575=CARTESIAN_POINT('Ctrl Pts',(-0.642000825785288,0.56311334974773,
-0.420824218001371));
#55576=CARTESIAN_POINT('Ctrl Pts',(-0.831551647635553,0.194379943122152,
-0.41039025539889));
#55577=CARTESIAN_POINT('Ctrl Pts',(-0.825097929205881,-0.220170643352128,
-0.39995629279641));
#55578=CARTESIAN_POINT('Ctrl Pts',(-0.624160872597549,-0.582824939487973,
-0.389522330193928));
#55579=CARTESIAN_POINT('Ctrl Pts',(-0.276103230945762,-0.808101918597746,
-0.379088367591449));
#55580=CARTESIAN_POINT('Ctrl Pts',(0.137034537726103,-0.842901678981725,
-0.368654404988967));
#55581=CARTESIAN_POINT('Ctrl Pts',(0.517871977672874,-0.679021590036204,
-0.358220442386487));
#55582=CARTESIAN_POINT('Ctrl Pts',(0.776642124272,-0.355089729166497,-0.347786479784006));
#55583=CARTESIAN_POINT('Ctrl Pts',(0.852350421415522,0.0525401187286473,
-0.337352517181526));
#55584=CARTESIAN_POINT('Ctrl Pts',(0.72715171179137,0.447785766997171,-0.326918554579045));
#55585=CARTESIAN_POINT('Ctrl Pts',(0.430556508150087,0.737484100106967,
-0.316484591976564));
#55586=CARTESIAN_POINT('Ctrl Pts',(0.0324750881634825,0.853350499154804,
-0.306050629374084));
#55587=CARTESIAN_POINT('Ctrl Pts',(-0.373261015454179,0.768074161753147,
-0.295616666771603));
#55588=CARTESIAN_POINT('Ctrl Pts',(-0.691015988779464,0.501755528036826,
-0.285182704169123));
#55589=CARTESIAN_POINT('Ctrl Pts',(-0.8458919979872,0.117168392128854,-0.274748741566642));
#55590=CARTESIAN_POINT('Ctrl Pts',(-0.801383310988863,-0.295036420454541,
-0.264314778964161));
#55591=CARTESIAN_POINT('Ctrl Pts',(-0.567981045319887,-0.637698404316488,
-0.253880816361681));
#55592=CARTESIAN_POINT('Ctrl Pts',(-0.200700305913994,-0.830048822576,-0.2434468537592));
#55593=CARTESIAN_POINT('Ctrl Pts',(0.213887378143152,-0.826749042700625,
-0.23301289115672));
#55594=CARTESIAN_POINT('Ctrl Pts',(0.578059804635804,-0.628576521295636,
-0.222578928554239));
#55595=CARTESIAN_POINT('Ctrl Pts',(0.805978085266888,-0.282243037988429,
-0.212144965951759));
#55596=CARTESIAN_POINT('Ctrl Pts',(0.843919785925286,0.130618633522338,
-0.201711003349278));
#55597=CARTESIAN_POINT('Ctrl Pts',(0.68294159842625,0.512690593115567,-0.191277040746797));
#55598=CARTESIAN_POINT('Ctrl Pts',(0.36098777693341,0.773919846182344,-0.180843078144317));
#55599=CARTESIAN_POINT('Ctrl Pts',(-0.0460544942459941,0.852722459491375,
-0.170409115541836));
#55600=CARTESIAN_POINT('Ctrl Pts',(-0.442240821285006,0.730543063661545,
-0.159975152939355));
#55601=CARTESIAN_POINT('Ctrl Pts',(-0.734187755498606,0.436142832866609,
-0.149541190336875));
#55602=CARTESIAN_POINT('Ctrl Pts',(-0.853077819122259,0.0389890385957994,
-0.139107227734394));
#55603=CARTESIAN_POINT('Ctrl Pts',(-0.770894241208358,-0.367455713931453,
-0.128673265131913));
#55604=CARTESIAN_POINT('Ctrl Pts',(-0.594951669076752,-0.580514449476566,
-0.121717290063593));
#55605=CARTESIAN_POINT('Ctrl Pts',(-0.487041437638041,-0.660130190455614,
-0.118239302529433));
#55606=CARTESIAN_POINT('Ctrl Pts',(0.816972063808647,-1.16980680969206E-14,
-1.1425283350431));
#55607=CARTESIAN_POINT('Ctrl Pts',(0.816972063808649,0.133547259366542,
-1.13905034750894));
#55608=CARTESIAN_POINT('Ctrl Pts',(0.750258545288667,0.400515882139589,
-1.13209437244062));
#55609=CARTESIAN_POINT('Ctrl Pts',(0.473136385937643,0.706683841755145,
-1.12166040983814));
#55610=CARTESIAN_POINT('Ctrl Pts',(0.0845750992767583,0.84622608784569,
-1.11122644723566));
#55611=CARTESIAN_POINT('Ctrl Pts',(-0.323961995775528,0.786331547179381,
-1.10079248463318));
#55612=CARTESIAN_POINT('Ctrl Pts',(-0.656117677249225,0.541077762637857,
-1.0903585220307));
#55613=CARTESIAN_POINT('Ctrl Pts',(-0.833630685095572,0.168293731192079,
-1.07992455942822));
#55614=CARTESIAN_POINT('Ctrl Pts',(-0.814643797129344,-0.244162209445375,
-1.06949059682573));
#55615=CARTESIAN_POINT('Ctrl Pts',(-0.603640408739925,-0.599065043663486,
-1.05905663422325));
#55616=CARTESIAN_POINT('Ctrl Pts',(-0.250351927233731,-0.812763520669612,
-1.04862267162077));
#55617=CARTESIAN_POINT('Ctrl Pts',(0.161946157548475,-0.834885534961222,
-1.03818870901829));
#55618=CARTESIAN_POINT('Ctrl Pts',(0.536072366553588,-0.660217414778485,
-1.02775474641581));
#55619=CARTESIAN_POINT('Ctrl Pts',(0.783841098330598,-0.32992972433277,
-1.01732078381333));
#55620=CARTESIAN_POINT('Ctrl Pts',(0.846851206973998,0.0781254429130661,
-1.00688682121085));
#55621=CARTESIAN_POINT('Ctrl Pts',(0.710250478470448,0.467765739743972,
-0.996452858608371));
#55622=CARTESIAN_POINT('Ctrl Pts',(0.406237059412565,0.747149238803466,
-0.98601889600589));
#55623=CARTESIAN_POINT('Ctrl Pts',(0.00646973450489691,0.850422646762807,
-0.97558493340341));
#55624=CARTESIAN_POINT('Ctrl Pts',(-0.394822561461409,0.753243438481209,
-0.965150970800928));
#55625=CARTESIAN_POINT('Ctrl Pts',(-0.703051471340727,0.478517673019027,
-0.954717008198449));
#55626=CARTESIAN_POINT('Ctrl Pts',(-0.845564538846854,0.0910007927061417,
-0.944283045595967));
#55627=CARTESIAN_POINT('Ctrl Pts',(-0.78877009670225,-0.317965829356397,
-0.933849082993488));
#55628=CARTESIAN_POINT('Ctrl Pts',(-0.546055127582371,-0.65198491670129,
-0.923415120391006));
#55629=CARTESIAN_POINT('Ctrl Pts',(-0.174629831956398,-0.83232503011057,
-0.912981157788526));
#55630=CARTESIAN_POINT('Ctrl Pts',(0.237957356762347,-0.816478309791074,
-0.902547195186046));
#55631=CARTESIAN_POINT('Ctrl Pts',(0.59445575953915,-0.608179976581176,
-0.892113232583564));
#55632=CARTESIAN_POINT('Ctrl Pts',(0.810835351688311,-0.256527905763967,
-0.881679269981085));
#55633=CARTESIAN_POINT('Ctrl Pts',(0.836093429239884,0.15559020392044,-0.871245307378603));
#55634=CARTESIAN_POINT('Ctrl Pts',(0.664276425899862,0.531034239923243,
-0.860811344776123));
#55635=CARTESIAN_POINT('Ctrl Pts',(0.335883224496113,0.781308513635209,
-0.850377382173642));
#55636=CARTESIAN_POINT('Ctrl Pts',(-0.0716808103619085,0.847421026056226,
-0.839943419571162));
#55637=CARTESIAN_POINT('Ctrl Pts',(-0.462349004389063,0.713788436525322,
-0.829509456968682));
#55638=CARTESIAN_POINT('Ctrl Pts',(-0.74403719180775,0.411909202596066,
-0.8190754943662));
#55639=CARTESIAN_POINT('Ctrl Pts',(-0.850348818857666,0.0129390974967731,
-0.808641531763721));
#55640=CARTESIAN_POINT('Ctrl Pts',(-0.756225235669137,-0.389080874515505,
-0.798207569161238));
#55641=CARTESIAN_POINT('Ctrl Pts',(-0.483852255600829,-0.699390826881937,
-0.787773606558759));
#55642=CARTESIAN_POINT('Ctrl Pts',(-0.0974307504743618,-0.844847786786835,
-0.777339643956278));
#55643=CARTESIAN_POINT('Ctrl Pts',(0.311956098428587,-0.791166181424496,
-0.766905681353798));
#55644=CARTESIAN_POINT('Ctrl Pts',(0.647811962414489,-0.550999269808317,
-0.756471718751317));
#55645=CARTESIAN_POINT('Ctrl Pts',(0.83097245715665,-0.180956650675365,
-0.746037756148837));
#55646=CARTESIAN_POINT('Ctrl Pts',(0.818264932259306,0.23173915208976,-0.735603793546355));
#55647=CARTESIAN_POINT('Ctrl Pts',(0.612684670796792,0.589811858262646,
-0.725169830943875));
#55648=CARTESIAN_POINT('Ctrl Pts',(0.262688872936025,0.808860364965553,
-0.714735868341394));
#55649=CARTESIAN_POINT('Ctrl Pts',(-0.149225161660734,0.837252880021285,
-0.704301905738914));
#55650=CARTESIAN_POINT('Ctrl Pts',(-0.525965422875295,0.668297020729719,
-0.693867943136433));
#55651=CARTESIAN_POINT('Ctrl Pts',(-0.778730689623804,0.341817271381426,
-0.683433980533953));
#55652=CARTESIAN_POINT('Ctrl Pts',(-0.847941812434699,-0.0652320220563885,
-0.673000017931472));
#55653=CARTESIAN_POINT('Ctrl Pts',(-0.717285079048033,-0.456905514687298,
-0.662566055328991));
#55654=CARTESIAN_POINT('Ctrl Pts',(-0.417557509750832,-0.740882082404003,
-0.652132092726512));
#55655=CARTESIAN_POINT('Ctrl Pts',(-0.0194077101906099,-0.850225778697497,
-0.64169813012403));
#55656=CARTESIAN_POINT('Ctrl Pts',(0.383316669102108,-0.759163266475053,
-0.63126416752155));
#55657=CARTESIAN_POINT('Ctrl Pts',(0.695689706150895,-0.489158835893097,
-0.620830204919069));
#55658=CARTESIAN_POINT('Ctrl Pts',(0.844082139686514,-0.103855069394057,
-0.610396242316588));
#55659=CARTESIAN_POINT('Ctrl Pts',(0.793516478173852,0.305928313242129,
-0.599962279714108));
#55660=CARTESIAN_POINT('Ctrl Pts',(0.555911523369752,0.643601516593405,
-0.589528317111627));
#55661=CARTESIAN_POINT('Ctrl Pts',(0.187272996707218,0.829571792360917,
-0.579094354509147));
#55662=CARTESIAN_POINT('Ctrl Pts',(-0.225507535723487,0.820004198348112,
-0.568660391906665));
#55663=CARTESIAN_POINT('Ctrl Pts',(-0.585133822119271,0.617153906403175,
-0.558226429304186));
#55664=CARTESIAN_POINT('Ctrl Pts',(-0.806838566139565,0.268834637214886,
-0.547792466701704));
#55665=CARTESIAN_POINT('Ctrl Pts',(-0.838363875501718,-0.142851483122669,
-0.537358504099225));
#55666=CARTESIAN_POINT('Ctrl Pts',(-0.67227893843802,-0.520866166024689,
-0.526924541496743));
#55667=CARTESIAN_POINT('Ctrl Pts',(-0.347731535882055,-0.776107797235483,
-0.516490578894264));
#55668=CARTESIAN_POINT('Ctrl Pts',(0.0587794585027789,-0.848413524900877,
-0.506056616291782));
#55669=CARTESIAN_POINT('Ctrl Pts',(0.451435581967084,-0.72074020930613,
-0.495622653689302));
#55670=CARTESIAN_POINT('Ctrl Pts',(0.737684095078986,-0.423181651119361,
-0.485188691086821));
#55671=CARTESIAN_POINT('Ctrl Pts',(0.850053532442601,-0.0258751996797124,
-0.474754728484341));
#55672=CARTESIAN_POINT('Ctrl Pts',(0.762057361351739,0.377530279562073,
-0.46432076588186));
#55673=CARTESIAN_POINT('Ctrl Pts',(0.494437106533235,0.691948322969065,
-0.453886803279379));
#55674=CARTESIAN_POINT('Ctrl Pts',(0.110273377789815,0.843267642049257,
-0.443452840676898));
#55675=CARTESIAN_POINT('Ctrl Pts',(-0.299882822714393,0.795820850831183,
-0.433018878074419));
#55676=CARTESIAN_POINT('Ctrl Pts',(-0.639353822881238,0.560791604023697,
-0.422584915471937));
#55677=CARTESIAN_POINT('Ctrl Pts',(-0.828123116802315,0.193578504473986,
-0.412150952869457));
#55678=CARTESIAN_POINT('Ctrl Pts',(-0.821696007390508,-0.219262868301158,
-0.401716990266976));
#55679=CARTESIAN_POINT('Ctrl Pts',(-0.621587424751335,-0.580421921850922,
-0.391283027664496));
#55680=CARTESIAN_POINT('Ctrl Pts',(-0.274964842917683,-0.804770072220884,
-0.380849065062015));
#55681=CARTESIAN_POINT('Ctrl Pts',(0.136469537176779,-0.839426351377121,
-0.370415102459535));
#55682=CARTESIAN_POINT('Ctrl Pts',(0.51573676448633,-0.676221948589207,
-0.359981139857054));
#55683=CARTESIAN_POINT('Ctrl Pts',(0.773439988269244,-0.353625675685112,
-0.349547177254573));
#55684=CARTESIAN_POINT('Ctrl Pts',(0.848836136151767,0.0523234930784053,
-0.339113214652093));
#55685=CARTESIAN_POINT('Ctrl Pts',(0.724153627343059,0.445939522912994,
-0.328679252049612));
#55686=CARTESIAN_POINT('Ctrl Pts',(0.428781301197015,0.734443414683686,
-0.318245289447131));
#55687=CARTESIAN_POINT('Ctrl Pts',(0.0323411916877275,0.849832090513251,
-0.307811326844651));
#55688=CARTESIAN_POINT('Ctrl Pts',(-0.371722040825158,0.764907351918338,
-0.29737736424217));
#55689=CARTESIAN_POINT('Ctrl Pts',(-0.688166893772684,0.499686763789953,
-0.28694340163969));
#55690=CARTESIAN_POINT('Ctrl Pts',(-0.84240434119643,0.116685300780245,
-0.276509439037209));
#55691=CARTESIAN_POINT('Ctrl Pts',(-0.798079165673271,-0.293819969988393,
-0.266075476434728));
#55692=CARTESIAN_POINT('Ctrl Pts',(-0.565639230046271,-0.635069140343272,
-0.255641513832248));
#55693=CARTESIAN_POINT('Ctrl Pts',(-0.199872807661195,-0.826626488317455,
-0.245207551229767));
#55694=CARTESIAN_POINT('Ctrl Pts',(0.213005508499063,-0.823340312573242,
-0.234773588627287));
#55695=CARTESIAN_POINT('Ctrl Pts',(0.575676435516455,-0.625984868845304,
-0.224339626024806));
#55696=CARTESIAN_POINT('Ctrl Pts',(0.802654992386151,-0.281079332570885,
-0.213905663422325));
#55697=CARTESIAN_POINT('Ctrl Pts',(0.840440266860436,0.130080080884035,
-0.203471700819845));
#55698=CARTESIAN_POINT('Ctrl Pts',(0.680125782303049,0.510576753259713,
-0.193037738217364));
#55699=CARTESIAN_POINT('Ctrl Pts',(0.359499429618295,0.770728914207573,
-0.182603775614884));
#55700=CARTESIAN_POINT('Ctrl Pts',(-0.0458646565737162,0.849206679729665,
-0.172169813012403));
#55701=CARTESIAN_POINT('Ctrl Pts',(-0.440417346097015,0.72753091896719,
-0.161735850409923));
#55702=CARTESIAN_POINT('Ctrl Pts',(-0.731160844709429,0.434344745947377,
-0.151301887807442));
#55703=CARTESIAN_POINT('Ctrl Pts',(-0.849560168473915,0.0388279800983555,
-0.140867925204961));
#55704=CARTESIAN_POINT('Ctrl Pts',(-0.767716584589533,-0.365940025647511,
-0.13043396260248));
#55705=CARTESIAN_POINT('Ctrl Pts',(-0.5924974211277,-0.578121984952227,
-0.12347798753416));
#55706=CARTESIAN_POINT('Ctrl Pts',(-0.485033396983243,-0.657408515958423,
-0.12));
#55707=CARTESIAN_POINT('',(-0.814921455736579,-0.139942643537184,-0.12));
#55708=CARTESIAN_POINT('',(-0.485033396983246,-0.657408515958421,-0.12));
#55709=CARTESIAN_POINT('Ctrl Pts',(-0.814921455736576,-0.139942643537195,
-0.12));
#55710=CARTESIAN_POINT('Ctrl Pts',(-0.797805299826955,-0.239614354303296,
-0.12));
#55711=CARTESIAN_POINT('Ctrl Pts',(-0.76198915728887,-0.33528609840046,
-0.12));
#55712=CARTESIAN_POINT('Ctrl Pts',(-0.676216606680933,-0.475719941382479,
-0.12));
#55713=CARTESIAN_POINT('Ctrl Pts',(-0.636663795100031,-0.52585283471045,
-0.12));
#55714=CARTESIAN_POINT('Ctrl Pts',(-0.553238444854244,-0.608184477072079,
-0.12));
#55715=CARTESIAN_POINT('Ctrl Pts',(-0.51637010940319,-0.636623334743938,
-0.12));
#55716=CARTESIAN_POINT('Ctrl Pts',(-0.485033396983242,-0.657408515958424,
-0.12));
#55717=CARTESIAN_POINT('',(0.826819918308061,8.40320865522751E-9,-1.12624999033503));
#55718=CARTESIAN_POINT('Ctrl Pts',(0.82685,-1.18395083925468E-14,-1.12625));
#55719=CARTESIAN_POINT('Ctrl Pts',(0.826850000000002,0.135161967341259,
-1.12277201246584));
#55720=CARTESIAN_POINT('Ctrl Pts',(0.793089927145682,0.2702602256041,-1.11929402493168));
#55721=CARTESIAN_POINT('Ctrl Pts',(0.729464420950729,0.389454322909817,
-1.11581603739752));
#55722=CARTESIAN_POINT('Ctrl Pts',(0.665838914755776,0.508648420215534,
-1.11233804986336));
#55723=CARTESIAN_POINT('Ctrl Pts',(0.572347975220189,0.611938356564128,
-1.1088600623292));
#55724=CARTESIAN_POINT('Ctrl Pts',(0.460059281045234,0.687121564557396,
-1.10538207479504));
#55725=CARTESIAN_POINT('Ctrl Pts',(0.347770586870279,0.762304772550664,
-1.10190408726088));
#55726=CARTESIAN_POINT('Ctrl Pts',(0.216684138055956,0.809381252188606,
-1.09842609972672));
#55727=CARTESIAN_POINT('Ctrl Pts',(0.082228133557474,0.822816371973693,
-1.09494811219256));
#55728=CARTESIAN_POINT('Ctrl Pts',(-0.0522278709410078,0.836251491758779,
-1.0914701246584));
#55729=CARTESIAN_POINT('Ctrl Pts',(-0.190053431123648,0.816045251691008,
-1.08799213712424));
#55730=CARTESIAN_POINT('Ctrl Pts',(-0.314994835569263,0.764572277302744,
-1.08451414959008));
#55731=CARTESIAN_POINT('Ctrl Pts',(-0.439936240014878,0.713099302914481,
-1.08103616205592));
#55732=CARTESIAN_POINT('Ctrl Pts',(-0.551993488723467,0.630359594205724,
-1.07755817452176));
#55733=CARTESIAN_POINT('Ctrl Pts',(-0.63796533003704,0.526107851543772,
-1.0740801869876));
#55734=CARTESIAN_POINT('Ctrl Pts',(-0.723937171350614,0.421856108881819,
-1.07060219945344));
#55735=CARTESIAN_POINT('Ctrl Pts',(-0.783823605269172,0.296092332266671,
-1.06712421191928));
#55736=CARTESIAN_POINT('Ctrl Pts',(-0.810564079439897,0.163636625868307,
-1.06364622438512));
#55737=CARTESIAN_POINT('Ctrl Pts',(-0.837304553610622,0.0311809194699431,
-1.06016823685096));
#55738=CARTESIAN_POINT('Ctrl Pts',(-0.830899068033516,-0.107966716711637,
-1.0566902493168));
#55739=CARTESIAN_POINT('Ctrl Pts',(-0.792103889995619,-0.237406190245854,
-1.05321226178264));
#55740=CARTESIAN_POINT('Ctrl Pts',(-0.753308711957722,-0.36684566378007,
-1.04973427424848));
#55741=CARTESIAN_POINT('Ctrl Pts',(-0.682123841459035,-0.486576974666924,
-1.04625628671432));
#55742=CARTESIAN_POINT('Ctrl Pts',(-0.586938062717305,-0.582489677808403,
-1.04277829918016));
#55743=CARTESIAN_POINT('Ctrl Pts',(-0.491752283975575,-0.678402380949881,
-1.039300311646));
#55744=CARTESIAN_POINT('Ctrl Pts',(-0.372565596990802,-0.750496476345984,
-1.03582232411183));
#55745=CARTESIAN_POINT('Ctrl Pts',(-0.243425062820339,-0.790275105642176,
-1.03234433657767));
#55746=CARTESIAN_POINT('Ctrl Pts',(-0.114284528649877,-0.830053734938369,
-1.02886634904351));
#55747=CARTESIAN_POINT('Ctrl Pts',(0.0248098527062749,-0.837516898134649,
-1.02538836150935));
#55748=CARTESIAN_POINT('Ctrl Pts',(0.157465332643295,-0.81178514359785,
-1.02191037397519));
#55749=CARTESIAN_POINT('Ctrl Pts',(0.290120812580316,-0.78605338906105,
-1.01843238644103));
#55750=CARTESIAN_POINT('Ctrl Pts',(0.416337391098204,-0.727126716791171,
-1.01495439890687));
#55751=CARTESIAN_POINT('Ctrl Pts',(0.521239760584476,-0.641949852425356,
-1.01147641137271));
#55752=CARTESIAN_POINT('Ctrl Pts',(0.626142130070747,-0.55677298805954,
-1.00799842383855));
#55753=CARTESIAN_POINT('Ctrl Pts',(0.709730290525401,-0.445345931597789,
-1.00452043630439));
#55754=CARTESIAN_POINT('Ctrl Pts',(0.762153030458445,-0.320800915734339,
-1.00104244877023));
#55755=CARTESIAN_POINT('Ctrl Pts',(0.814575770391489,-0.19625589987089,
-0.997564461236073));
#55756=CARTESIAN_POINT('Ctrl Pts',(0.835833089802922,-0.0585929246057423,
-0.994086473701913));
#55757=CARTESIAN_POINT('Ctrl Pts',(0.823419690225199,0.0759637968315813,
-0.990608486167753));
#55758=CARTESIAN_POINT('Ctrl Pts',(0.811006290647475,0.210520518268905,
-0.987130498633592));
#55759=CARTESIAN_POINT('Ctrl Pts',(0.764922172080595,0.341970985878405,
-0.983652511099432));
#55760=CARTESIAN_POINT('Ctrl Pts',(0.690598576442017,0.45482313634507,-0.980174523565272));
#55761=CARTESIAN_POINT('Ctrl Pts',(0.616274980803439,0.567675286811736,
-0.976696536031112));
#55762=CARTESIAN_POINT('Ctrl Pts',(0.513711908093162,0.661929120135569,
-0.973218548496952));
#55763=CARTESIAN_POINT('Ctrl Pts',(0.394996892421951,0.726476383047983,
-0.969740560962791));
#55764=CARTESIAN_POINT('Ctrl Pts',(0.276281876750738,0.791023645960397,
-0.966262573428631));
#55765=CARTESIAN_POINT('Ctrl Pts',(0.14141491811859,0.825864338461392,-0.962784585894471));
#55766=CARTESIAN_POINT('Ctrl Pts',(0.00629072459521057,0.826892319144936,
-0.95930659836031));
#55767=CARTESIAN_POINT('Ctrl Pts',(-0.128833468928168,0.82792029982848,
-0.95582861082615));
#55768=CARTESIAN_POINT('Ctrl Pts',(-0.264214897342778,0.795135568694573,
-0.95235062329199));
#55769=CARTESIAN_POINT('Ctrl Pts',(-0.383898224562574,0.73240196143868,
-0.94887263575783));
#55770=CARTESIAN_POINT('Ctrl Pts',(-0.50358155178237,0.669668354182788,
-0.94539464822367));
#55771=CARTESIAN_POINT('Ctrl Pts',(-0.607566777807351,0.576985870804911,
-0.94191666068951));
#55772=CARTESIAN_POINT('Ctrl Pts',(-0.683598754197438,0.465277577070776,
-0.93843867315535));
#55773=CARTESIAN_POINT('Ctrl Pts',(-0.759630730587524,0.353569283336641,
-0.934960685621189));
#55774=CARTESIAN_POINT('Ctrl Pts',(-0.807709457342714,0.222835179246249,
-0.931482698087029));
#55775=CARTESIAN_POINT('Ctrl Pts',(-0.822168630942392,0.088482893712577,
-0.928004710552869));
#55776=CARTESIAN_POINT('Ctrl Pts',(-0.83662780454207,-0.0458693918210959,
-0.924526723018708));
#55777=CARTESIAN_POINT('Ctrl Pts',(-0.817467424986234,-0.183839858798048,
-0.921048735484548));
#55778=CARTESIAN_POINT('Ctrl Pts',(-0.76694563285593,-0.309168039331654,
-0.917570747950388));
#55779=CARTESIAN_POINT('Ctrl Pts',(-0.716423840725626,-0.43449621986526,
-0.914092760416228));
#55780=CARTESIAN_POINT('Ctrl Pts',(-0.634540636020853,-0.54718211395552,
-0.910614772882068));
#55781=CARTESIAN_POINT('Ctrl Pts',(-0.530946339389749,-0.63394515926719,
-0.907136785347908));
#55782=CARTESIAN_POINT('Ctrl Pts',(-0.427352042758645,-0.720708204578859,
-0.903658797813747));
#55783=CARTESIAN_POINT('Ctrl Pts',(-0.30204665420121,-0.781548401111939,
-0.900180810279587));
#55784=CARTESIAN_POINT('Ctrl Pts',(-0.169798002666685,-0.809295445778766,
-0.896702822745427));
#55785=CARTESIAN_POINT('Ctrl Pts',(-0.0375493511321594,-0.837042490445593,
-0.893224835211267));
#55786=CARTESIAN_POINT('Ctrl Pts',(0.101642563379456,-0.831696383246166,
-0.889746847677107));
#55787=CARTESIAN_POINT('Ctrl Pts',(0.231373319484608,-0.793887188023756,
-0.886268860142946));
#55788=CARTESIAN_POINT('Ctrl Pts',(0.36110407558976,-0.756077992801346,
-0.882790872608786));
#55789=CARTESIAN_POINT('Ctrl Pts',(0.481373673288448,-0.685805709555952,
-0.879312885074626));
#55790=CARTESIAN_POINT('Ctrl Pts',(0.578007775213603,-0.591352257171592,
-0.875834897540466));
#55791=CARTESIAN_POINT('Ctrl Pts',(0.674641877138758,-0.496898804787232,
-0.872356910006305));
#55792=CARTESIAN_POINT('Ctrl Pts',(0.747640483290378,-0.378264183263906,
-0.868878922472145));
#55793=CARTESIAN_POINT('Ctrl Pts',(0.788400364817745,-0.249430040350937,
-0.865400934937985));
#55794=CARTESIAN_POINT('Ctrl Pts',(0.829160246345111,-0.120595897437968,
-0.861922947403825));
#55795=CARTESIAN_POINT('Ctrl Pts',(0.837681403248224,0.0184377668646435,
-0.858444959869665));
#55796=CARTESIAN_POINT('Ctrl Pts',(0.81295957713844,0.151285181729246,-0.854966972335505));
#55797=CARTESIAN_POINT('Ctrl Pts',(0.788237751028655,0.284132596593849,
-0.851488984801344));
#55798=CARTESIAN_POINT('Ctrl Pts',(0.730272941905971,0.410793762020445,
-0.848010997267184));
#55799=CARTESIAN_POINT('Ctrl Pts',(0.645896574970356,0.51634106433082,-0.844533009733024));
#55800=CARTESIAN_POINT('Ctrl Pts',(0.561520208034741,0.621888366641196,
-0.841055022198864));
#55801=CARTESIAN_POINT('Ctrl Pts',(0.450732283286197,0.706321805835353,
-0.837577034664704));
#55802=CARTESIAN_POINT('Ctrl Pts',(0.326589678383619,0.759690504248875,
-0.834099047130543));
#55803=CARTESIAN_POINT('Ctrl Pts',(0.202447073481041,0.813059202662397,
-0.830621059596383));
#55804=CARTESIAN_POINT('Ctrl Pts',(0.0649497884244317,0.835363160295282,
-0.827143072062223));
#55805=CARTESIAN_POINT('Ctrl Pts',(-0.0696974754768497,0.823973750907557,
-0.823665084528063));
#55806=CARTESIAN_POINT('Ctrl Pts',(-0.204344739378132,0.812584341519832,
-0.820187096993903));
#55807=CARTESIAN_POINT('Ctrl Pts',(-0.336141982124086,0.767501565111495,
-0.816709109459743));
#55808=CARTESIAN_POINT('Ctrl Pts',(-0.449556279182332,0.694038638780562,
-0.813231121925582));
#55809=CARTESIAN_POINT('Ctrl Pts',(-0.562970576240578,0.620575712449629,
-0.809753134391422));
#55810=CARTESIAN_POINT('Ctrl Pts',(-0.658001927611118,0.518732636196097,
-0.806275146857262));
#55811=CARTESIAN_POINT('Ctrl Pts',(-0.723450441867886,0.400512095240227,
-0.802797159323102));
#55812=CARTESIAN_POINT('Ctrl Pts',(-0.788898956124654,0.282291554284355,
-0.799319171788942));
#55813=CARTESIAN_POINT('Ctrl Pts',(-0.824764633267649,0.147693548626145,
-0.795841184254781));
#55814=CARTESIAN_POINT('Ctrl Pts',(-0.826820534669346,0.0125810858710678,
-0.792363196720621));
#55815=CARTESIAN_POINT('Ctrl Pts',(-0.828876436071043,-0.122531376884008,
-0.788885209186461));
#55816=CARTESIAN_POINT('Ctrl Pts',(-0.79712256173144,-0.258158296735951,
-0.7854072216523));
#55817=CARTESIAN_POINT('Ctrl Pts',(-0.735301254991326,-0.378315403705377,
-0.78192923411814));
#55818=CARTESIAN_POINT('Ctrl Pts',(-0.67347994825121,-0.498472510674805,
-0.77845124658398));
#55819=CARTESIAN_POINT('Ctrl Pts',(-0.581591209110583,-0.603159804761717,
-0.77497325904982));
#55820=CARTESIAN_POINT('Ctrl Pts',(-0.470464557373384,-0.68003939630587,
-0.77149527151566));
#55821=CARTESIAN_POINT('Ctrl Pts',(-0.359337905636187,-0.756918987850021,
-0.768017283981499));
#55822=CARTESIAN_POINT('Ctrl Pts',(-0.228973341302421,-0.805990876851411,
-0.76453929644734));
#55823=CARTESIAN_POINT('Ctrl Pts',(-0.0947349410194663,-0.82147171054311,
-0.761061308913179));
#55824=CARTESIAN_POINT('Ctrl Pts',(0.0395034592634891,-0.83695254423481,
-0.757583321379019));
#55825=CARTESIAN_POINT('Ctrl Pts',(0.177615695495633,-0.818842322616818,
-0.754105333844859));
#55826=CARTESIAN_POINT('Ctrl Pts',(0.303324591480697,-0.769275420428635,
-0.750627346310698));
#55827=CARTESIAN_POINT('Ctrl Pts',(0.42903348746576,-0.719708518240453,
-0.747149358776538));
#55828=CARTESIAN_POINT('Ctrl Pts',(0.542339043203747,-0.638684935482078,
-0.743671371242378));
#55829=CARTESIAN_POINT('Ctrl Pts',(0.629887666391188,-0.535753682209324,
-0.740193383708218));
#55830=CARTESIAN_POINT('Ctrl Pts',(0.71743628957863,-0.432822428936568,
-0.736715396174058));
#55831=CARTESIAN_POINT('Ctrl Pts',(0.779227980215528,-0.307983505149434,
-0.733237408639898));
#55832=CARTESIAN_POINT('Ctrl Pts',(0.807980297126493,-0.175949764785207,
-0.729759421105738));
#55833=CARTESIAN_POINT('Ctrl Pts',(0.836732614037458,-0.0439160244209799,
-0.726281433571577));
#55834=CARTESIAN_POINT('Ctrl Pts',(0.83244555722249,0.0953125325203378,
-0.722803446037417));
#55835=CARTESIAN_POINT('Ctrl Pts',(0.795624376477293,0.22532716619996,-0.719325458503256));
#55836=CARTESIAN_POINT('Ctrl Pts',(0.758803195732096,0.355341799879582,
-0.715847470969096));
#55837=CARTESIAN_POINT('Ctrl Pts',(0.689447891056671,0.476142510297508,
-0.712369483434936));
#55838=CARTESIAN_POINT('Ctrl Pts',(0.595732311091411,0.573492365942453,
-0.708891495900776));
#55839=CARTESIAN_POINT('Ctrl Pts',(0.502016731126152,0.670842221587398,
-0.705413508366616));
#55840=CARTESIAN_POINT('Ctrl Pts',(0.383940875871059,0.744741222459363,
-0.701935520832456));
#55841=CARTESIAN_POINT('Ctrl Pts',(0.255420539849088,0.786480023964872,
-0.698457533298296));
#55842=CARTESIAN_POINT('Ctrl Pts',(0.126900203827117,0.828218825470381,
-0.694979545764135));
#55843=CARTESIAN_POINT('Ctrl Pts',(-0.0120646129617348,0.837797427609435,
-0.691501558229975));
#55844=CARTESIAN_POINT('Ctrl Pts',(-0.145096253695276,0.814086947098516,
-0.688023570695815));
#55845=CARTESIAN_POINT('Ctrl Pts',(-0.278127894428818,0.790376466587597,
-0.684545583161654));
#55846=CARTESIAN_POINT('Ctrl Pts',(-0.405226359107049,0.733376903426708,
-0.681067595627494));
#55847=CARTESIAN_POINT('Ctrl Pts',(-0.511412496278356,0.649805924044191,
-0.677589608093334));
#55848=CARTESIAN_POINT('Ctrl Pts',(-0.617598633449664,0.566234944661674,
-0.674111620559174));
#55849=CARTESIAN_POINT('Ctrl Pts',(-0.702872443114044,0.456092549057531,
-0.670633633025015));
#55850=CARTESIAN_POINT('Ctrl Pts',(-0.757184005997862,0.332359536245938,
-0.667155645490854));
#55851=CARTESIAN_POINT('Ctrl Pts',(-0.811495568881679,0.208626523434346,
-0.663677657956694));
#55852=CARTESIAN_POINT('Ctrl Pts',(-0.834844884984934,0.0713028934153015,
-0.660199670422533));
#55853=CARTESIAN_POINT('Ctrl Pts',(-0.824480127658203,-0.0634271185637466,
-0.656721682888373));
#55854=CARTESIAN_POINT('Ctrl Pts',(-0.814115370331471,-0.198157130542796,
-0.653243695354212));
#55855=CARTESIAN_POINT('Ctrl Pts',(-0.770036539574752,-0.330293524481851,
-0.649765707820053));
#55856=CARTESIAN_POINT('Ctrl Pts',(-0.697438532772424,-0.444263405286587,
-0.646287720285893));
#55857=CARTESIAN_POINT('Ctrl Pts',(-0.624840525970095,-0.558233286091323,
-0.642809732751732));
#55858=CARTESIAN_POINT('Ctrl Pts',(-0.523723343122159,-0.654036653761738,
-0.639331745217572));
#55859=CARTESIAN_POINT('Ctrl Pts',(-0.406004119499086,-0.720382631122071,
-0.635853757683411));
#55860=CARTESIAN_POINT('Ctrl Pts',(-0.288284895876013,-0.786728608482404,
-0.632375770149251));
#55861=CARTESIAN_POINT('Ctrl Pts',(-0.153963631477803,-0.823617195532651,
-0.628897782615092));
#55862=CARTESIAN_POINT('Ctrl Pts',(-0.018870718651746,-0.82670089890489,
-0.625419795080931));
#55863=CARTESIAN_POINT('Ctrl Pts',(0.116222194174311,-0.829784602277128,
-0.621941807546771));
#55864=CARTESIAN_POINT('Ctrl Pts',(0.252086755428218,-0.799063421971358,
-0.618463820012611));
#55865=CARTESIAN_POINT('Ctrl Pts',(0.372710687974431,-0.738157993482569,
-0.614985832478451));
#55866=CARTESIAN_POINT('Ctrl Pts',(0.493334620520646,-0.677252564993779,
-0.61150784494429));
#55867=CARTESIAN_POINT('Ctrl Pts',(0.598717924359164,-0.586162888321972,
-0.608029857410131));
#55868=CARTESIAN_POINT('Ctrl Pts',(0.676440681809117,-0.475624310003393,
-0.604551869875971));
#55869=CARTESIAN_POINT('Ctrl Pts',(0.754163439259069,-0.365085731684814,
-0.60107388234181));
#55870=CARTESIAN_POINT('Ctrl Pts',(0.804225650320453,-0.235098251719462,
-0.59759589480765));
#55871=CARTESIAN_POINT('Ctrl Pts',(0.820727248116851,-0.100981505589522,
-0.594117907273489));
#55872=CARTESIAN_POINT('Ctrl Pts',(0.837228845913249,0.0331352405404182,
-0.590639919739329));
#55873=CARTESIAN_POINT('Ctrl Pts',(0.820169830444662,0.171381252834949,
-0.587161932205169));
#55874=CARTESIAN_POINT('Ctrl Pts',(0.771560686864993,0.29746358896007,-0.583683944671009));
#55875=CARTESIAN_POINT('Ctrl Pts',(0.722951543285324,0.42354592508519,-0.580205957136849));
#55876=CARTESIAN_POINT('Ctrl Pts',(0.642792271594575,0.537464585040901,
-0.576727969602689));
#55877=CARTESIAN_POINT('Ctrl Pts',(0.540530018726793,0.625793719309964,
-0.573249982068529));
#55878=CARTESIAN_POINT('Ctrl Pts',(0.43826776585901,0.714122853579028,-0.569771994534368));
#55879=CARTESIAN_POINT('Ctrl Pts',(0.313902531814194,0.776862462161444,
-0.566294007000208));
#55880=CARTESIAN_POINT('Ctrl Pts',(0.182091343967062,0.80661838729653,-0.562816019466048));
#55881=CARTESIAN_POINT('Ctrl Pts',(0.0502801561199283,0.836374312431616,
-0.559338031931887));
#55882=CARTESIAN_POINT('Ctrl Pts',(-0.0889769855295217,0.833146554119371,
-0.555860044397727));
#55883=CARTESIAN_POINT('Ctrl Pts',(-0.219267972300293,0.79731551884803,
-0.552382056863567));
#55884=CARTESIAN_POINT('Ctrl Pts',(-0.34955895907106,0.76148448357669,-0.548904069329407));
#55885=CARTESIAN_POINT('Ctrl Pts',(-0.470883790963148,0.693050171346257,
-0.545426081795247));
#55886=CARTESIAN_POINT('Ctrl Pts',(-0.568943766286064,0.600077887508625,
-0.541948094261086));
#55887=CARTESIAN_POINT('Ctrl Pts',(-0.667003741608982,0.507105603670991,
-0.538470106726926));
#55888=CARTESIAN_POINT('Ctrl Pts',(-0.741798860362727,0.389595348226158,
-0.534992119192766));
#55889=CARTESIAN_POINT('Ctrl Pts',(-0.784514166249514,0.261396257101007,
-0.531514131658606));
#55890=CARTESIAN_POINT('Ctrl Pts',(-0.827229472136301,0.133197165975855,
-0.528036144124446));
#55891=CARTESIAN_POINT('Ctrl Pts',(-0.83786496515613,-0.00569076082960968,
-0.524558156590286));
#55892=CARTESIAN_POINT('Ctrl Pts',(-0.815167202467579,-0.138898928339155,
-0.521080169056126));
#55893=CARTESIAN_POINT('Ctrl Pts',(-0.79246943977903,-0.272107095848698,
-0.517602181521965));
#55894=CARTESIAN_POINT('Ctrl Pts',(-0.736438421382098,-0.399635504062321,
-0.514124193987804));
#55895=CARTESIAN_POINT('Ctrl Pts',(-0.653677666152339,-0.506454330661924,
-0.510646206453644));
#55896=CARTESIAN_POINT('Ctrl Pts',(-0.570916910922578,-0.613273157261528,
-0.507168218919484));
#55897=CARTESIAN_POINT('Ctrl Pts',(-0.461426418859987,-0.699382402247118,
-0.503690231385324));
#55898=CARTESIAN_POINT('Ctrl Pts',(-0.338110159082288,-0.754633686365733,
-0.500212243851164));
#55899=CARTESIAN_POINT('Ctrl Pts',(-0.214793899304592,-0.809884970484346,
-0.496734256317004));
#55900=CARTESIAN_POINT('Ctrl Pts',(-0.0776518718117877,-0.834278293735986,
-0.493256268782844));
#55901=CARTESIAN_POINT('Ctrl Pts',(0.0571530908599681,-0.824938788321739,
-0.489778281248683));
#55902=CARTESIAN_POINT('Ctrl Pts',(0.191958053531728,-0.815599282907491,
-0.486300293714523));
#55903=CARTESIAN_POINT('Ctrl Pts',(0.324425951382439,-0.772526948827354,
-0.482822306180363));
#55904=CARTESIAN_POINT('Ctrl Pts',(0.438944820023649,-0.700798063101627,
-0.479344318646203));
#55905=CARTESIAN_POINT('Ctrl Pts',(0.553463688664858,-0.6290691773759,-0.475866331112043));
#55906=CARTESIAN_POINT('Ctrl Pts',(0.650033528096565,-0.528683740004585,
-0.472388343577882));
#55907=CARTESIAN_POINT('Ctrl Pts',(0.717273128843362,-0.411472646614376,
-0.468910356043722));
#55908=CARTESIAN_POINT('Ctrl Pts',(0.784512729590159,-0.294261553224167,
-0.465432368509562));
#55909=CARTESIAN_POINT('Ctrl Pts',(0.822422091652046,-0.160224803815064,
-0.461954380975402));
#55910=CARTESIAN_POINT('Ctrl Pts',(0.826533418528119,-0.0251592593056137,
-0.458476393441242));
#55911=CARTESIAN_POINT('Ctrl Pts',(0.830644745404193,0.109906285203834,
-0.454998405907081));
#55912=CARTESIAN_POINT('Ctrl Pts',(0.800958037094454,0.246000624813629,
-0.451520418372921));
#55913=CARTESIAN_POINT('Ctrl Pts',(0.740972011706928,0.367084401928998,
-0.448042430838761));
#55914=CARTESIAN_POINT('Ctrl Pts',(0.680985986319401,0.488168179044368,
-0.444564443304601));
#55915=CARTESIAN_POINT('Ctrl Pts',(0.590700643854085,0.594241393665313,
-0.441086455770441));
#55916=CARTESIAN_POINT('Ctrl Pts',(0.480756536280455,0.672802818882485,
-0.437608468236281));
#55917=CARTESIAN_POINT('Ctrl Pts',(0.370812428706822,0.751364244099658,
-0.43413048070212));
#55918=CARTESIAN_POINT('Ctrl Pts',(0.241209556024874,0.802413879913059,
-0.43065249316796));
#55919=CARTESIAN_POINT('Ctrl Pts',(0.107222225940712,0.819935286798217,
-0.427174505633799));
#55920=CARTESIAN_POINT('Ctrl Pts',(-0.0267651041434491,0.837456693683375,
-0.423696518099639));
#55921=CARTESIAN_POINT('Ctrl Pts',(-0.165136891629824,0.821449871640292,
-0.420218530565479));
#55922=CARTESIAN_POINT('Ctrl Pts',(-0.291585370986894,0.773801299882001,
-0.416740543031319));
#55923=CARTESIAN_POINT('Ctrl Pts',(-0.418033850343963,0.726152728123709,
-0.413262555497159));
#55924=CARTESIAN_POINT('Ctrl Pts',(-0.532559021571728,0.646862406650209,
-0.409784567962999));
#55925=CARTESIAN_POINT('Ctrl Pts',(-0.621663554948791,0.545275072528486,
-0.406306580428838));
#55926=CARTESIAN_POINT('Ctrl Pts',(-0.710768088325855,0.443687738406764,
-0.402828592894678));
#55927=CARTESIAN_POINT('Ctrl Pts',(-0.774451983852219,0.319803391636819,
-0.399350605360518));
#55928=CARTESIAN_POINT('Ctrl Pts',(-0.805209795112539,0.188222384767189,
-0.395872617826358));
#55929=CARTESIAN_POINT('Ctrl Pts',(-0.835967606372859,0.0566413778975608,
-0.392394630292198));
#55930=CARTESIAN_POINT('Ctrl Pts',(-0.833799333367138,-0.0826362890717533,
-0.388916642758038));
#55931=CARTESIAN_POINT('Ctrl Pts',(-0.798960517260375,-0.213196088453224,
-0.385438655223877));
#55932=CARTESIAN_POINT('Ctrl Pts',(-0.764121701153612,-0.343755887834697,
-0.381960667689717));
#55933=CARTESIAN_POINT('Ctrl Pts',(-0.696612341945807,-0.465597819628327,
-0.378482680155557));
#55934=CARTESIAN_POINT('Ctrl Pts',(-0.604388734927783,-0.564362239491937,
-0.375004692621397));
#55935=CARTESIAN_POINT('Ctrl Pts',(-0.512165127909759,-0.663126659355548,
-0.371526705087236));
#55936=CARTESIAN_POINT('Ctrl Pts',(-0.395227273081517,-0.738813567289139,
-0.368048717553076));
#55937=CARTESIAN_POINT('Ctrl Pts',(-0.267356846266639,-0.782502905444178,
-0.364570730018916));
#55938=CARTESIAN_POINT('Ctrl Pts',(-0.139486419451759,-0.826192243599218,
-0.361092742484756));
#55939=CARTESIAN_POINT('Ctrl Pts',(-0.000683420650243682,-0.837884011975705,
-0.357614754950596));
#55940=CARTESIAN_POINT('Ctrl Pts',(0.132693564325656,-0.816200280725184,
-0.354136767416435));
#55941=CARTESIAN_POINT('Ctrl Pts',(0.266070549301554,-0.794516549474664,
-0.350658779882275));
#55942=CARTESIAN_POINT('Ctrl Pts',(0.394021520451837,-0.739457318597138,
-0.347180792348115));
#55943=CARTESIAN_POINT('Ctrl Pts',(0.501466854431083,-0.657511577224757,
-0.343702804813955));
#55944=CARTESIAN_POINT('Ctrl Pts',(0.608912188410329,-0.575565835852376,
-0.340224817279794));
#55945=CARTESIAN_POINT('Ctrl Pts',(0.695851885218537,-0.466733583985141,
-0.336746829745634));
#55946=CARTESIAN_POINT('Ctrl Pts',(0.752039692950413,-0.343841214072567,
-0.333268842211474));
#55947=CARTESIAN_POINT('Ctrl Pts',(0.808227500682287,-0.220948844159995,
-0.329790854677314));
#55948=CARTESIAN_POINT('Ctrl Pts',(0.83366341933783,-0.0839963562020835,
-0.326312867143154));
#55949=CARTESIAN_POINT('Ctrl Pts',(0.825349706352787,0.050875755454292,
-0.322834879608994));
#55950=CARTESIAN_POINT('Ctrl Pts',(0.817035993367744,0.185747867110668,
-0.319356892074833));
#55951=CARTESIAN_POINT('Ctrl Pts',(0.774972648742117,0.318539602465508,
-0.315878904540673));
#55952=CARTESIAN_POINT('Ctrl Pts',(0.704117035339796,0.433600831232204,
-0.312400917006513));
#55953=CARTESIAN_POINT('Ctrl Pts',(0.633261421937474,0.548662059998902,
-0.308922929472353));
#55954=CARTESIAN_POINT('Ctrl Pts',(0.533613539758457,0.645992782177456,
-0.305444941938193));
#55955=CARTESIAN_POINT('Ctrl Pts',(0.416917360096596,0.7141221149324,-0.301966954404032));
#55956=CARTESIAN_POINT('Ctrl Pts',(0.300221180434735,0.782251447687343,
-0.298488966869872));
#55957=CARTESIAN_POINT('Ctrl Pts',(0.16647670329003,0.821179391018677,-0.295010979335712));
#55958=CARTESIAN_POINT('Ctrl Pts',(0.031446343894929,0.826318103348089,
-0.291532991801552));
#55959=CARTESIAN_POINT('Ctrl Pts',(-0.103584015500172,0.8314568156775,-0.288055004267392));
#55960=CARTESIAN_POINT('Ctrl Pts',(-0.239900257145668,0.802806297004991,
-0.284577016733231));
#55961=CARTESIAN_POINT('Ctrl Pts',(-0.361436871197806,0.743743146577004,
-0.281099029199071));
#55962=CARTESIAN_POINT('Ctrl Pts',(-0.482973485249944,0.684679996149017,
-0.277621041664911));
#55963=CARTESIAN_POINT('Ctrl Pts',(-0.589730471708724,0.595204213965552,
-0.274143054130751));
#55964=CARTESIAN_POINT('Ctrl Pts',(-0.669126018040229,0.485860939630313,
-0.270665066596591));
#55965=CARTESIAN_POINT('Ctrl Pts',(-0.748521564371732,0.376517665295076,
-0.267187079062431));
#55966=CARTESIAN_POINT('Ctrl Pts',(-0.800555670575961,0.247306898808065,
-0.26370909152827));
#55967=CARTESIAN_POINT('Ctrl Pts',(-0.819095872468407,0.113456740014407,
-0.26023110399411));
#55968=CARTESIAN_POINT('Ctrl Pts',(-0.837636074360853,-0.0203934187792517,
-0.25675311645995));
#55969=CARTESIAN_POINT('Ctrl Pts',(-0.822682371941515,-0.158882969879557,
-0.25327512892579));
#55970=CARTESIAN_POINT('Ctrl Pts',(-0.775997129713513,-0.285690276024395,
-0.24979714139163));
#55971=CARTESIAN_POINT('Ctrl Pts',(-0.729311887485511,-0.412497582169235,
-0.246319153857469));
#55972=CARTESIAN_POINT('Ctrl Pts',(-0.650895105448843,-0.527622643358608,
-0.242841166323309));
#55973=CARTESIAN_POINT('Ctrl Pts',(-0.549988569180355,-0.617497415744048,
-0.239363178789149));
#55974=CARTESIAN_POINT('Ctrl Pts',(-0.449082032911868,-0.707372188129487,
-0.235885191254989));
#55975=CARTESIAN_POINT('Ctrl Pts',(-0.325685742411561,-0.771996671710993,
-0.232407203720828));
#55976=CARTESIAN_POINT('Ctrl Pts',(-0.194342531999369,-0.803754595401518,
-0.228929216186668));
#55977=CARTESIAN_POINT('Ctrl Pts',(-0.0629993215871771,-0.835512519092042,
-0.225451228652508));
#55978=CARTESIAN_POINT('Ctrl Pts',(0.0762908087369,-0.834403882891584,-0.221973241118348));
#55979=CARTESIAN_POINT('Ctrl Pts',(0.207111865361516,-0.800559289665401,
-0.218495253584188));
#55980=CARTESIAN_POINT('Ctrl Pts',(0.337932921986132,-0.766714696439218,
-0.215017266050027));
#55981=CARTESIAN_POINT('Ctrl Pts',(0.460284904911287,-0.70013414618731,
-0.211539278515867));
#55982=CARTESIAN_POINT('Ctrl Pts',(0.559748052092256,-0.608664578014501,
-0.208061290981707));
#55983=CARTESIAN_POINT('Ctrl Pts',(0.659211199273223,-0.517195009841694,
-0.204583303447547));
#55984=CARTESIAN_POINT('Ctrl Pts',(0.735785510710006,-0.400836423747985,
-0.201105315913387));
#55985=CARTESIAN_POINT('Ctrl Pts',(0.780446355236762,-0.273302013173142,
-0.197627328379227));
#55986=CARTESIAN_POINT('Ctrl Pts',(0.825107199763519,-0.145767602598297,
-0.194149340845066));
#55987=CARTESIAN_POINT('Ctrl Pts',(0.837854577380249,-0.00705736754231678,
-0.190671353310906));
#55988=CARTESIAN_POINT('Ctrl Pts',(0.817186127412103,0.126480620590234,
-0.187193365776746));
#55989=CARTESIAN_POINT('Ctrl Pts',(0.796517677443957,0.260018608722786,
-0.183715378242586));
#55990=CARTESIAN_POINT('Ctrl Pts',(0.742433399890935,0.388384349931908,
-0.180237390708426));
#55991=CARTESIAN_POINT('Ctrl Pts',(0.661307424905576,0.496450160114788,
-0.176759403174265));
#55992=CARTESIAN_POINT('Ctrl Pts',(0.580181449920217,0.604515970297668,
-0.173281415640105));
#55993=CARTESIAN_POINT('Ctrl Pts',(0.472013777502521,0.692281849454306,
-0.169803428105945));
#55994=CARTESIAN_POINT('Ctrl Pts',(0.349552390106812,0.749402561227559,
-0.166325440571785));
#55995=CARTESIAN_POINT('Ctrl Pts',(0.227091002711104,0.806523273000812,
-0.162847453037624));
#55996=CARTESIAN_POINT('Ctrl Pts',(0.0903359003373833,0.83299881739068,
-0.159369465503464));
#55997=CARTESIAN_POINT('Ctrl Pts',(-0.0445955159864435,0.825712101000813,
-0.155891477969304));
#55998=CARTESIAN_POINT('Ctrl Pts',(-0.17952693231027,0.818425384610945,
-0.152413490435144));
#55999=CARTESIAN_POINT('Ctrl Pts',(-0.312634662584204,0.777376407441342,
-0.148935502900984));
#56000=CARTESIAN_POINT('Ctrl Pts',(-0.428231669765087,0.707396742051741,
-0.145457515366823));
#56001=CARTESIAN_POINT('Ctrl Pts',(-0.543828676945968,0.637417076662141,
-0.141979527832663));
#56002=CARTESIAN_POINT('Ctrl Pts',(-0.6419149610338,0.538506723052544,-0.138501540298503));
#56003=CARTESIAN_POINT('Ctrl Pts',(-0.710929916311711,0.422335058963047,
-0.135023552764343));
#56004=CARTESIAN_POINT('Ctrl Pts',(-0.779944871589624,0.306163394873548,
-0.131545565230183));
#56005=CARTESIAN_POINT('Ctrl Pts',(-0.819888498057614,0.172730420304148,
-0.128067577696022));
#56006=CARTESIAN_POINT('Ctrl Pts',(-0.826054786734804,0.0377369297661749,
-0.124589590161862));
#56007=CARTESIAN_POINT('Ctrl Pts',(-0.828767153927045,-0.0216426961432744,
-0.123059726774575));
#56008=CARTESIAN_POINT('Ctrl Pts',(-0.824944083444903,-0.0813242598465086,
-0.121529863387287));
#56009=CARTESIAN_POINT('Ctrl Pts',(-0.814862045042683,-0.139933199781809,
-0.12));
#56010=CARTESIAN_POINT('',(0.589301091561381,0.565833523687246,-1.12625));
#56011=CARTESIAN_POINT('Ctrl Pts',(0.589301091561381,0.565833523687246,
-1.12625));
#56012=CARTESIAN_POINT('Ctrl Pts',(0.616667481029585,0.540044898914149,
-1.12625));
#56013=CARTESIAN_POINT('Ctrl Pts',(0.648190221269366,0.505777024736586,
-1.12625));
#56014=CARTESIAN_POINT('Ctrl Pts',(0.716478059012945,0.410513493212772,
-1.12625));
#56015=CARTESIAN_POINT('Ctrl Pts',(0.746976021141481,0.354408470381541,
-1.12625));
#56016=CARTESIAN_POINT('Ctrl Pts',(0.807743006623444,0.201482947924183,
-1.12625));
#56017=CARTESIAN_POINT('Ctrl Pts',(0.826850000000001,0.10113013137271,-1.12625));
#56018=CARTESIAN_POINT('Ctrl Pts',(0.82685,-1.11022302462516E-14,-1.12625));
#56019=CARTESIAN_POINT('Ctrl Pts',(0.589258732516958,0.56579182741905,-1.12625));
#56020=CARTESIAN_POINT('Ctrl Pts',(0.548574338866333,0.608188043340012,
-1.12472013661271));
#56021=CARTESIAN_POINT('Ctrl Pts',(0.400588145741338,0.732737761006612,
-1.11971228569126));
#56022=CARTESIAN_POINT('Ctrl Pts',(0.0845750992767583,0.84622608784569,
-1.11122644723566));
#56023=CARTESIAN_POINT('Ctrl Pts',(-0.323961995775528,0.786331547179381,
-1.10079248463318));
#56024=CARTESIAN_POINT('Ctrl Pts',(-0.656117677249225,0.541077762637857,
-1.0903585220307));
#56025=CARTESIAN_POINT('Ctrl Pts',(-0.833630685095572,0.168293731192079,
-1.07992455942822));
#56026=CARTESIAN_POINT('Ctrl Pts',(-0.814643797129344,-0.244162209445375,
-1.06949059682573));
#56027=CARTESIAN_POINT('Ctrl Pts',(-0.603640408739925,-0.599065043663486,
-1.05905663422325));
#56028=CARTESIAN_POINT('Ctrl Pts',(-0.250351927233731,-0.812763520669612,
-1.04862267162077));
#56029=CARTESIAN_POINT('Ctrl Pts',(0.161946157548475,-0.834885534961222,
-1.03818870901829));
#56030=CARTESIAN_POINT('Ctrl Pts',(0.536072366553588,-0.660217414778485,
-1.02775474641581));
#56031=CARTESIAN_POINT('Ctrl Pts',(0.783841098330598,-0.32992972433277,
-1.01732078381333));
#56032=CARTESIAN_POINT('Ctrl Pts',(0.846851206973998,0.0781254429130661,
-1.00688682121085));
#56033=CARTESIAN_POINT('Ctrl Pts',(0.710250478470448,0.467765739743972,
-0.996452858608371));
#56034=CARTESIAN_POINT('Ctrl Pts',(0.406237059412565,0.747149238803466,
-0.98601889600589));
#56035=CARTESIAN_POINT('Ctrl Pts',(0.00646973450489691,0.850422646762807,
-0.97558493340341));
#56036=CARTESIAN_POINT('Ctrl Pts',(-0.394822561461409,0.753243438481209,
-0.965150970800928));
#56037=CARTESIAN_POINT('Ctrl Pts',(-0.703051471340727,0.478517673019027,
-0.954717008198449));
#56038=CARTESIAN_POINT('Ctrl Pts',(-0.845564538846854,0.0910007927061417,
-0.944283045595967));
#56039=CARTESIAN_POINT('Ctrl Pts',(-0.78877009670225,-0.317965829356397,
-0.933849082993488));
#56040=CARTESIAN_POINT('Ctrl Pts',(-0.546055127582371,-0.65198491670129,
-0.923415120391006));
#56041=CARTESIAN_POINT('Ctrl Pts',(-0.174629831956398,-0.83232503011057,
-0.912981157788526));
#56042=CARTESIAN_POINT('Ctrl Pts',(0.237957356762347,-0.816478309791074,
-0.902547195186046));
#56043=CARTESIAN_POINT('Ctrl Pts',(0.59445575953915,-0.608179976581176,
-0.892113232583564));
#56044=CARTESIAN_POINT('Ctrl Pts',(0.810835351688311,-0.256527905763967,
-0.881679269981085));
#56045=CARTESIAN_POINT('Ctrl Pts',(0.836093429239884,0.15559020392044,-0.871245307378603));
#56046=CARTESIAN_POINT('Ctrl Pts',(0.664276425899862,0.531034239923243,
-0.860811344776123));
#56047=CARTESIAN_POINT('Ctrl Pts',(0.335883224496113,0.781308513635209,
-0.850377382173642));
#56048=CARTESIAN_POINT('Ctrl Pts',(-0.0716808103619085,0.847421026056226,
-0.839943419571162));
#56049=CARTESIAN_POINT('Ctrl Pts',(-0.462349004389063,0.713788436525322,
-0.829509456968682));
#56050=CARTESIAN_POINT('Ctrl Pts',(-0.74403719180775,0.411909202596066,
-0.8190754943662));
#56051=CARTESIAN_POINT('Ctrl Pts',(-0.850348818857666,0.0129390974967731,
-0.808641531763721));
#56052=CARTESIAN_POINT('Ctrl Pts',(-0.756225235669137,-0.389080874515505,
-0.798207569161238));
#56053=CARTESIAN_POINT('Ctrl Pts',(-0.483852255600829,-0.699390826881937,
-0.787773606558759));
#56054=CARTESIAN_POINT('Ctrl Pts',(-0.0974307504743618,-0.844847786786835,
-0.777339643956278));
#56055=CARTESIAN_POINT('Ctrl Pts',(0.311956098428587,-0.791166181424496,
-0.766905681353798));
#56056=CARTESIAN_POINT('Ctrl Pts',(0.647811962414489,-0.550999269808317,
-0.756471718751317));
#56057=CARTESIAN_POINT('Ctrl Pts',(0.83097245715665,-0.180956650675365,
-0.746037756148837));
#56058=CARTESIAN_POINT('Ctrl Pts',(0.818264932259306,0.23173915208976,-0.735603793546355));
#56059=CARTESIAN_POINT('Ctrl Pts',(0.612684670796792,0.589811858262646,
-0.725169830943875));
#56060=CARTESIAN_POINT('Ctrl Pts',(0.262688872936025,0.808860364965553,
-0.714735868341394));
#56061=CARTESIAN_POINT('Ctrl Pts',(-0.149225161660734,0.837252880021285,
-0.704301905738914));
#56062=CARTESIAN_POINT('Ctrl Pts',(-0.525965422875295,0.668297020729719,
-0.693867943136433));
#56063=CARTESIAN_POINT('Ctrl Pts',(-0.778730689623804,0.341817271381426,
-0.683433980533953));
#56064=CARTESIAN_POINT('Ctrl Pts',(-0.847941812434699,-0.0652320220563885,
-0.673000017931472));
#56065=CARTESIAN_POINT('Ctrl Pts',(-0.717285079048033,-0.456905514687298,
-0.662566055328991));
#56066=CARTESIAN_POINT('Ctrl Pts',(-0.417557509750832,-0.740882082404003,
-0.652132092726512));
#56067=CARTESIAN_POINT('Ctrl Pts',(-0.0194077101906099,-0.850225778697497,
-0.64169813012403));
#56068=CARTESIAN_POINT('Ctrl Pts',(0.383316669102108,-0.759163266475053,
-0.63126416752155));
#56069=CARTESIAN_POINT('Ctrl Pts',(0.695689706150895,-0.489158835893097,
-0.620830204919069));
#56070=CARTESIAN_POINT('Ctrl Pts',(0.844082139686514,-0.103855069394057,
-0.610396242316588));
#56071=CARTESIAN_POINT('Ctrl Pts',(0.793516478173852,0.305928313242129,
-0.599962279714108));
#56072=CARTESIAN_POINT('Ctrl Pts',(0.555911523369752,0.643601516593405,
-0.589528317111627));
#56073=CARTESIAN_POINT('Ctrl Pts',(0.187272996707218,0.829571792360917,
-0.579094354509147));
#56074=CARTESIAN_POINT('Ctrl Pts',(-0.225507535723487,0.820004198348112,
-0.568660391906665));
#56075=CARTESIAN_POINT('Ctrl Pts',(-0.585133822119271,0.617153906403175,
-0.558226429304186));
#56076=CARTESIAN_POINT('Ctrl Pts',(-0.806838566139565,0.268834637214886,
-0.547792466701704));
#56077=CARTESIAN_POINT('Ctrl Pts',(-0.838363875501718,-0.142851483122669,
-0.537358504099225));
#56078=CARTESIAN_POINT('Ctrl Pts',(-0.67227893843802,-0.520866166024689,
-0.526924541496743));
#56079=CARTESIAN_POINT('Ctrl Pts',(-0.347731535882055,-0.776107797235483,
-0.516490578894264));
#56080=CARTESIAN_POINT('Ctrl Pts',(0.0587794585027789,-0.848413524900877,
-0.506056616291782));
#56081=CARTESIAN_POINT('Ctrl Pts',(0.451435581967084,-0.72074020930613,
-0.495622653689302));
#56082=CARTESIAN_POINT('Ctrl Pts',(0.737684095078986,-0.423181651119361,
-0.485188691086821));
#56083=CARTESIAN_POINT('Ctrl Pts',(0.850053532442601,-0.0258751996797124,
-0.474754728484341));
#56084=CARTESIAN_POINT('Ctrl Pts',(0.762057361351739,0.377530279562073,
-0.46432076588186));
#56085=CARTESIAN_POINT('Ctrl Pts',(0.494437106533235,0.691948322969065,
-0.453886803279379));
#56086=CARTESIAN_POINT('Ctrl Pts',(0.110273377789815,0.843267642049257,
-0.443452840676898));
#56087=CARTESIAN_POINT('Ctrl Pts',(-0.299882822714393,0.795820850831183,
-0.433018878074419));
#56088=CARTESIAN_POINT('Ctrl Pts',(-0.639353822881238,0.560791604023697,
-0.422584915471937));
#56089=CARTESIAN_POINT('Ctrl Pts',(-0.828123116802315,0.193578504473986,
-0.412150952869457));
#56090=CARTESIAN_POINT('Ctrl Pts',(-0.821696007390508,-0.219262868301158,
-0.401716990266976));
#56091=CARTESIAN_POINT('Ctrl Pts',(-0.621587424751335,-0.580421921850922,
-0.391283027664496));
#56092=CARTESIAN_POINT('Ctrl Pts',(-0.274964842917683,-0.804770072220884,
-0.380849065062015));
#56093=CARTESIAN_POINT('Ctrl Pts',(0.136469537176779,-0.839426351377121,
-0.370415102459535));
#56094=CARTESIAN_POINT('Ctrl Pts',(0.51573676448633,-0.676221948589207,
-0.359981139857054));
#56095=CARTESIAN_POINT('Ctrl Pts',(0.773439988269244,-0.353625675685112,
-0.349547177254573));
#56096=CARTESIAN_POINT('Ctrl Pts',(0.848836136151767,0.0523234930784053,
-0.339113214652093));
#56097=CARTESIAN_POINT('Ctrl Pts',(0.724153627343059,0.445939522912994,
-0.328679252049612));
#56098=CARTESIAN_POINT('Ctrl Pts',(0.428781301197015,0.734443414683686,
-0.318245289447131));
#56099=CARTESIAN_POINT('Ctrl Pts',(0.0323411916877275,0.849832090513251,
-0.307811326844651));
#56100=CARTESIAN_POINT('Ctrl Pts',(-0.371722040825158,0.764907351918338,
-0.29737736424217));
#56101=CARTESIAN_POINT('Ctrl Pts',(-0.688166893772684,0.499686763789953,
-0.28694340163969));
#56102=CARTESIAN_POINT('Ctrl Pts',(-0.84240434119643,0.116685300780245,
-0.276509439037209));
#56103=CARTESIAN_POINT('Ctrl Pts',(-0.798079165673271,-0.293819969988393,
-0.266075476434728));
#56104=CARTESIAN_POINT('Ctrl Pts',(-0.565639230046271,-0.635069140343272,
-0.255641513832248));
#56105=CARTESIAN_POINT('Ctrl Pts',(-0.199872807661195,-0.826626488317455,
-0.245207551229767));
#56106=CARTESIAN_POINT('Ctrl Pts',(0.213005508499063,-0.823340312573242,
-0.234773588627287));
#56107=CARTESIAN_POINT('Ctrl Pts',(0.575676435516455,-0.625984868845304,
-0.224339626024806));
#56108=CARTESIAN_POINT('Ctrl Pts',(0.802654992386151,-0.281079332570885,
-0.213905663422325));
#56109=CARTESIAN_POINT('Ctrl Pts',(0.840440266860436,0.130080080884035,
-0.203471700819845));
#56110=CARTESIAN_POINT('Ctrl Pts',(0.680125782303049,0.510576753259713,
-0.193037738217364));
#56111=CARTESIAN_POINT('Ctrl Pts',(0.359499429618295,0.770728914207573,
-0.182603775614884));
#56112=CARTESIAN_POINT('Ctrl Pts',(-0.0458646565737162,0.849206679729665,
-0.172169813012403));
#56113=CARTESIAN_POINT('Ctrl Pts',(-0.440417346097015,0.72753091896719,
-0.161735850409923));
#56114=CARTESIAN_POINT('Ctrl Pts',(-0.731160844709429,0.434344745947377,
-0.151301887807442));
#56115=CARTESIAN_POINT('Ctrl Pts',(-0.849560168473915,0.0388279800983555,
-0.140867925204961));
#56116=CARTESIAN_POINT('Ctrl Pts',(-0.767716584589533,-0.365940025647511,
-0.13043396260248));
#56117=CARTESIAN_POINT('Ctrl Pts',(-0.5924974211277,-0.578121984952227,
-0.12347798753416));
#56118=CARTESIAN_POINT('Ctrl Pts',(-0.485033396983243,-0.657408515958423,
-0.12));
#56119=CARTESIAN_POINT('Ctrl Pts',(0.546314451000137,0.52455872774923,-1.15727273924394));
#56120=CARTESIAN_POINT('Ctrl Pts',(0.459330425190867,0.615150357993711,
-1.15374460067508));
#56121=CARTESIAN_POINT('Ctrl Pts',(0.239517155169437,0.752140157504834,
-1.14668832353737));
#56122=CARTESIAN_POINT('Ctrl Pts',(-0.148496413265629,0.775239352992087,
-1.1361039078308));
#56123=CARTESIAN_POINT('Ctrl Pts',(-0.500415877733314,0.610427930590285,
-1.12551949212423));
#56124=CARTESIAN_POINT('Ctrl Pts',(-0.731074678445063,0.297631408040504,
-1.11493507641766));
#56125=CARTESIAN_POINT('Ctrl Pts',(-0.78448657507111,-0.0873109114175063,
-1.10435066071109));
#56126=CARTESIAN_POINT('Ctrl Pts',(-0.647739858405566,-0.451090008407739,
-1.09376624500452));
#56127=CARTESIAN_POINT('Ctrl Pts',(-0.35396552579895,-0.705517309450156,
-1.08318182929794));
#56128=CARTESIAN_POINT('Ctrl Pts',(0.0256119661671881,-0.788917676587972,
-1.07259741359137));
#56129=CARTESIAN_POINT('Ctrl Pts',(0.398982356900771,-0.681072808505694,
-1.0620129978848));
#56130=CARTESIAN_POINT('Ctrl Pts',(0.675632891112322,-0.40812628276753,
-1.05142858217823));
#56131=CARTESIAN_POINT('Ctrl Pts',(0.788500750688369,-0.0362440247522399,
-1.04084416647166));
#56132=CARTESIAN_POINT('Ctrl Pts',(0.710224521156417,0.344424265850664,
-1.03025975076509));
#56133=CARTESIAN_POINT('Ctrl Pts',(0.459779801870057,0.641599200064961,
-1.01967533505852));
#56134=CARTESIAN_POINT('Ctrl Pts',(0.097877817393331,0.783241287520996,
-1.00909091935195));
#56135=CARTESIAN_POINT('Ctrl Pts',(-0.287751124101878,0.735014472176637,
-0.998506503645378));
#56136=CARTESIAN_POINT('Ctrl Pts',(-0.603625085401645,0.508609617298406,
-0.987922087938805));
#56137=CARTESIAN_POINT('Ctrl Pts',(-0.773171671953705,0.158910506780707,
-0.977337672232237));
#56138=CARTESIAN_POINT('Ctrl Pts',(-0.755290373416537,-0.229310787602246,
-0.966753256525664));
#56139=CARTESIAN_POINT('Ctrl Pts',(-0.554315867123395,-0.561943861908008,
-0.956168840819094));
#56140=CARTESIAN_POINT('Ctrl Pts',(-0.218967255152568,-0.758353694545465,
-0.945584425112524));
#56141=CARTESIAN_POINT('Ctrl Pts',(0.169462156609868,-0.770927728297873,
-0.935000009405952));
#56142=CARTESIAN_POINT('Ctrl Pts',(0.516811513855876,-0.596617837396196,
-0.924415593699383));
#56143=CARTESIAN_POINT('Ctrl Pts',(0.738878357065632,-0.277679236275888,
-0.91383117799281));
#56144=CARTESIAN_POINT('Ctrl Pts',(0.781830502198587,0.108572789396219,
-0.903246762286241));
#56145=CARTESIAN_POINT('Ctrl Pts',(0.635255734092279,0.468505215644772,
-0.892662346579669));
#56146=CARTESIAN_POINT('Ctrl Pts',(0.334685876135465,0.714865266390365,
-0.882077930873099));
#56147=CARTESIAN_POINT('Ctrl Pts',(-0.0470166324849972,0.787931736286691,
-0.871493515166528));
#56148=CARTESIAN_POINT('Ctrl Pts',(-0.417321635893157,0.669992266368472,
-0.860909099459957));
#56149=CARTESIAN_POINT('Ctrl Pts',(-0.686461896723767,0.389637073600391,
-0.850324683753386));
#56150=CARTESIAN_POINT('Ctrl Pts',(-0.78919396038351,0.0148282727314064,
-0.839740268046816));
#56151=CARTESIAN_POINT('Ctrl Pts',(-0.700614103026785,-0.363575113859107,
-0.829155852340244));
#56152=CARTESIAN_POINT('Ctrl Pts',(-0.442195350963465,-0.65384268472174,
-0.818571436633674));
#56153=CARTESIAN_POINT('Ctrl Pts',(-0.0765821114814538,-0.785609422664232,
-0.807987020927103));
#56154=CARTESIAN_POINT('Ctrl Pts',(0.307595728844424,-0.726933182881658,
-0.797402605220531));
#56155=CARTESIAN_POINT('Ctrl Pts',(0.617207958261566,-0.492037926420706,
-0.786818189513963));
#56156=CARTESIAN_POINT('Ctrl Pts',(0.77720013723641,-0.137865628267142,
-0.776233773807389));
#56157=CARTESIAN_POINT('Ctrl Pts',(0.748787869734938,0.249727273071264,
-0.765649358100821));
#56158=CARTESIAN_POINT('Ctrl Pts',(0.538858696398575,0.576782706132406,
-0.755064942394248));
#56159=CARTESIAN_POINT('Ctrl Pts',(0.198302456030381,0.764017748949666,
-0.744480526687679));
#56160=CARTESIAN_POINT('Ctrl Pts',(-0.19032514031589,0.766043945045929,
-0.733896110981107));
#56161=CARTESIAN_POINT('Ctrl Pts',(-0.532815196286458,0.582370115462682,
-0.723311695274537));
#56162=CARTESIAN_POINT('Ctrl Pts',(-0.746143216224097,0.257521427575559,
-0.712727279567965));
#56163=CARTESIAN_POINT('Ctrl Pts',(-0.778595432221923,-0.129754143290109,
-0.702142863861395));
#56164=CARTESIAN_POINT('Ctrl Pts',(-0.622304962251659,-0.485575451124495,
-0.691558448154824));
#56165=CARTESIAN_POINT('Ctrl Pts',(-0.315158855058528,-0.723686313851513,
-0.680974032448254));
#56166=CARTESIAN_POINT('Ctrl Pts',(0.0683862731776896,-0.786365247463709,
-0.670389616741681));
#56167=CARTESIAN_POINT('Ctrl Pts',(0.435353589178266,-0.658417980592417,
-0.659805201035112));
#56168=CARTESIAN_POINT('Ctrl Pts',(0.696784958823668,-0.370860763541915,
-0.64922078532854));
#56169=CARTESIAN_POINT('Ctrl Pts',(0.789305673168617,0.00659841508485966,
-0.63863636962197));
#56170=CARTESIAN_POINT('Ctrl Pts',(0.690487385718296,0.382458043374312,
-0.6280519539154));
#56171=CARTESIAN_POINT('Ctrl Pts',(0.424285064899528,0.665604363327792,
-0.617467538208828));
#56172=CARTESIAN_POINT('Ctrl Pts',(0.0552299665647739,0.787398650983763,
-0.606883122502257));
#56173=CARTESIAN_POINT('Ctrl Pts',(-0.327213666821637,0.718316226339718,
-0.596298706795687));
#56174=CARTESIAN_POINT('Ctrl Pts',(-0.630336020111223,0.475103658718956,
-0.585714291089115));
#56175=CARTESIAN_POINT('Ctrl Pts',(-0.780655892709758,0.116719158475909,
-0.575129875382546));
#56176=CARTESIAN_POINT('Ctrl Pts',(-0.741733594202337,-0.269959737756351,
-0.564545459675974));
#56177=CARTESIAN_POINT('Ctrl Pts',(-0.52300444729998,-0.591196526446356,
-0.553961043969404));
#56178=CARTESIAN_POINT('Ctrl Pts',(-0.177491530455701,-0.76911880837377,
-0.543376628262832));
#56179=CARTESIAN_POINT('Ctrl Pts',(0.211047875895708,-0.760595673704304,
-0.532792212556262));
#56180=CARTESIAN_POINT('Ctrl Pts',(0.548426253918526,-0.567693252373749,
-0.522207796849691));
#56181=CARTESIAN_POINT('Ctrl Pts',(0.752858251913653,-0.237173854594711,
-0.511623381143121));
#56182=CARTESIAN_POINT('Ctrl Pts',(0.7747866251265,0.150839882998094,-0.501038965436549));
#56183=CARTESIAN_POINT('Ctrl Pts',(0.608895621771465,0.502287872206109,
-0.490454549729979));
#56184=CARTESIAN_POINT('Ctrl Pts',(0.295399597411609,0.731974086035053,
-0.479870134023407));
#56185=CARTESIAN_POINT('Ctrl Pts',(-0.0897055208909376,0.784219296051475,
-0.469285718316837));
#56186=CARTESIAN_POINT('Ctrl Pts',(-0.453064735918984,0.646358514947002,
-0.458701302610266));
#56187=CARTESIAN_POINT('Ctrl Pts',(-0.706594568913726,0.351811170884772,
-0.448116886903695));
#56188=CARTESIAN_POINT('Ctrl Pts',(-0.788835756602106,-0.028020240612635,
-0.437532471197125));
#56189=CARTESIAN_POINT('Ctrl Pts',(-0.679851857001812,-0.401059144402238,
-0.426948055490553));
#56190=CARTESIAN_POINT('Ctrl Pts',(-0.40606212854653,-0.676875566510097,
-0.416363639783983));
#56191=CARTESIAN_POINT('Ctrl Pts',(-0.033837123384323,-0.788607655212059,
-0.405779224077412));
#56192=CARTESIAN_POINT('Ctrl Pts',(0.346590485190783,-0.709169951669662,
-0.395194808370841));
#56193=CARTESIAN_POINT('Ctrl Pts',(0.642999595336517,-0.457819293150201,
-0.38461039266427));
#56194=CARTESIAN_POINT('Ctrl Pts',(0.78353639273709,-0.0954866798140887,
-0.3740259769577));
#56195=CARTESIAN_POINT('Ctrl Pts',(0.734132744595481,0.28999327252796,-0.363441561251129));
#56196=CARTESIAN_POINT('Ctrl Pts',(0.506764802819437,0.605174701533939,
-0.352857145544558));
#56197=CARTESIAN_POINT('Ctrl Pts',(0.156549813679528,0.773653113881338,
-0.342272729837987));
#56198=CARTESIAN_POINT('Ctrl Pts',(-0.231615093084919,0.754586929064552,
-0.331688314131416));
#56199=CARTESIAN_POINT('Ctrl Pts',(-0.563633182964234,0.552598063281491,
-0.321103898424845));
#56200=CARTESIAN_POINT('Ctrl Pts',(-0.759018516340423,0.216651511277527,
-0.310519482718275));
#56201=CARTESIAN_POINT('Ctrl Pts',(-0.770406886705707,-0.171814470849831,
-0.299935067011704));
#56202=CARTESIAN_POINT('Ctrl Pts',(-0.595037595541395,-0.518630163437193,
-0.289350651305133));
#56203=CARTESIAN_POINT('Ctrl Pts',(-0.275422660164443,-0.739722476337535,
-0.278766235598562));
#56204=CARTESIAN_POINT('Ctrl Pts',(0.11095865910622,-0.78149546229302,-0.268181819891991));
#56205=CARTESIAN_POINT('Ctrl Pts',(0.470442038027593,-0.63382275802318,
-0.257597404185421));
#56206=CARTESIAN_POINT('Ctrl Pts',(0.715883472822082,-0.332502328862262,
-0.24701298847885));
#56207=CARTESIAN_POINT('Ctrl Pts',(0.787784607225333,0.0494214101901834,
-0.236428572772279));
#56208=CARTESIAN_POINT('Ctrl Pts',(0.668715255345623,0.419364726111387,
-0.225844157065708));
#56209=CARTESIAN_POINT('Ctrl Pts',(0.387540164029785,0.687647957073743,
-0.215259741359137));
#56210=CARTESIAN_POINT('Ctrl Pts',(0.0124189653016963,0.789235606485636,
-0.204675325652567));
#56211=CARTESIAN_POINT('Ctrl Pts',(-0.365711157649466,0.699500976810326,
-0.194090909945995));
#56212=CARTESIAN_POINT('Ctrl Pts',(-0.655190820886885,0.440197805626207,
-0.183506494239425));
#56213=CARTESIAN_POINT('Ctrl Pts',(-0.785836630350135,0.0741833682121523,
-0.172922078532854));
#56214=CARTESIAN_POINT('Ctrl Pts',(-0.72599658874823,-0.309812190918401,
-0.162337662826283));
#56215=CARTESIAN_POINT('Ctrl Pts',(-0.490140575868292,-0.618708756217204,
-0.151753247119713));
#56216=CARTESIAN_POINT('Ctrl Pts',(-0.135514917188131,-0.777613622822956,
-0.141168831413141));
#56217=CARTESIAN_POINT('Ctrl Pts',(0.252058240770739,-0.748030699511335,
-0.130584415706571));
#56218=CARTESIAN_POINT('Ctrl Pts',(0.469550542503088,-0.607385125337185,
-0.123528138568857));
#56219=CARTESIAN_POINT('Ctrl Pts',(0.555007866453742,-0.515351924808608,
-0.12));
#56220=CARTESIAN_POINT('Ctrl Pts',(0.560643331187219,0.538316993061902,
-1.14693182616263));
#56221=CARTESIAN_POINT('Ctrl Pts',(0.471377865299383,0.631284684590043,
-1.14340368759377));
#56222=CARTESIAN_POINT('Ctrl Pts',(0.245799274584164,0.771867488863265,
-1.13634741045606));
#56223=CARTESIAN_POINT('Ctrl Pts',(-0.152391216542384,0.795572536170746,
-1.12576299474949));
#56224=CARTESIAN_POINT('Ctrl Pts',(-0.513540917978225,0.626438396109299,
-1.11517857904291));
#56225=CARTESIAN_POINT('Ctrl Pts',(-0.750249498836636,0.305437763479057,
-1.10459416333635));
#56226=CARTESIAN_POINT('Ctrl Pts',(-0.805062296840851,-0.089600925138424,
-1.09400974762977));
#56227=CARTESIAN_POINT('Ctrl Pts',(-0.664728951054495,-0.462921316681264,
-1.0834253319232));
#56228=CARTESIAN_POINT('Ctrl Pts',(-0.363249427405883,-0.724021804395359,
-1.07284091621663));
#56229=CARTESIAN_POINT('Ctrl Pts',(0.02628372360266,-0.809609618462481,
-1.06225650051006));
#56230=CARTESIAN_POINT('Ctrl Pts',(0.409446971882717,-0.698936166602649,
-1.05167208480349));
#56231=CARTESIAN_POINT('Ctrl Pts',(0.693353569614376,-0.418830727060134,
-1.04108766909692));
#56232=CARTESIAN_POINT('Ctrl Pts',(0.809181757319903,-0.0371946426376386,
-1.03050325339035));
#56233=CARTESIAN_POINT('Ctrl Pts',(0.728852478097603,0.353457916763361,
-1.01991883768378));
#56234=CARTESIAN_POINT('Ctrl Pts',(0.471839028349194,0.658427233899738,
-1.00933442197721));
#56235=CARTESIAN_POINT('Ctrl Pts',(0.100444982724277,0.803784347558887,
-0.998750006270635));
#56236=CARTESIAN_POINT('Ctrl Pts',(-0.295298336835141,0.754292626522196,
-0.988165590564065));
#56237=CARTESIAN_POINT('Ctrl Pts',(-0.619457124094383,0.521949565115867,
-0.977581174857493));
#56238=CARTESIAN_POINT('Ctrl Pts',(-0.793450623446181,0.163078453661776,
-0.966996759150924));
#56239=CARTESIAN_POINT('Ctrl Pts',(-0.775100329472666,-0.235325211703864,
-0.956412343444351));
#56240=CARTESIAN_POINT('Ctrl Pts',(-0.568854610572829,-0.576682674425973,
-0.945827927737782));
#56241=CARTESIAN_POINT('Ctrl Pts',(-0.224710386344195,-0.778243996199904,
-0.935243512031209));
#56242=CARTESIAN_POINT('Ctrl Pts',(0.173906854958707,-0.791147825041528,
-0.92465909632464));
#56243=CARTESIAN_POINT('Ctrl Pts',(0.530366583189641,-0.612266088131419,
-0.914074680618068));
#56244=CARTESIAN_POINT('Ctrl Pts',(0.75825785440794,-0.284962280866332,
-0.903490264911497));
#56245=CARTESIAN_POINT('Ctrl Pts',(0.802336559785202,0.111420465286886,
-0.892905849204928));
#56246=CARTESIAN_POINT('Ctrl Pts',(0.651917389820589,0.480793294588512,
-0.882321433498355));
#56247=CARTESIAN_POINT('Ctrl Pts',(0.343464105982166,0.733614942027284,
-0.871737017791786));
#56248=CARTESIAN_POINT('Ctrl Pts',(-0.0482497971806113,0.808597818657716,
-0.861152602085215));
#56249=CARTESIAN_POINT('Ctrl Pts',(-0.428267258344188,0.687565001070053,
-0.850568186378643));
#56250=CARTESIAN_POINT('Ctrl Pts',(-0.704466601254544,0.399856578015558,
-0.839983770672074));
#56251=CARTESIAN_POINT('Ctrl Pts',(-0.809893148702622,0.0152171925979065,
-0.829399354965502));
#56252=CARTESIAN_POINT('Ctrl Pts',(-0.718989995374629,-0.373111058288097,
-0.818814939258931));
#56253=CARTESIAN_POINT('Ctrl Pts',(-0.453793367804573,-0.670991843916459,
-0.80823052355236));
#56254=CARTESIAN_POINT('Ctrl Pts',(-0.0785907273946572,-0.806214594778186,
-0.79764610784579));
#56255=CARTESIAN_POINT('Ctrl Pts',(0.315663431129437,-0.745999379030152,
-0.787061692139218));
#56256=CARTESIAN_POINT('Ctrl Pts',(0.633396252142961,-0.504943227538543,
-0.776477276432649));
#56257=CARTESIAN_POINT('Ctrl Pts',(0.797584748383812,-0.141481604497939,
-0.765892860726076));
#56258=CARTESIAN_POINT('Ctrl Pts',(0.768427276401429,0.256277186163868,
-0.755308445019508));
#56259=CARTESIAN_POINT('Ctrl Pts',(0.552992025078288,0.591910715788788,
-0.744724029312934));
#56260=CARTESIAN_POINT('Ctrl Pts',(0.203503585394728,0.78405660892392,-0.734139613606365));
#56261=CARTESIAN_POINT('Ctrl Pts',(-0.19531703852979,0.786135948628312,
-0.723555197899793));
#56262=CARTESIAN_POINT('Ctrl Pts',(-0.546790014443781,0.59764467317157,
-0.712970782193224));
#56263=CARTESIAN_POINT('Ctrl Pts',(-0.765713258217505,0.264275767817853,
-0.702386366486652));
#56264=CARTESIAN_POINT('Ctrl Pts',(-0.79901663953594,-0.133157369343488,
-0.691801950780082));
#56265=CARTESIAN_POINT('Ctrl Pts',(-0.638626941704345,-0.498311252727788,
-0.68121753507351));
#56266=CARTESIAN_POINT('Ctrl Pts',(-0.323424925022017,-0.742667350258706,
-0.67063311936694));
#56267=CARTESIAN_POINT('Ctrl Pts',(0.0701799264720704,-0.806990243550786,
-0.660048703660369));
#56268=CARTESIAN_POINT('Ctrl Pts',(0.446772158478292,-0.675687141859628,
-0.649464287953798));
#56269=CARTESIAN_POINT('Ctrl Pts',(0.71506041936268,-0.380587797921389,
-0.638879872247228));
#56270=CARTESIAN_POINT('Ctrl Pts',(0.810007791520257,0.00677148006419926,
-0.628295456540657));
#56271=CARTESIAN_POINT('Ctrl Pts',(0.708597671841125,0.392489254282357,
-0.617711040834086));
#56272=CARTESIAN_POINT('Ctrl Pts',(0.435413326011757,0.683062010945685,
-0.607126625127516));
#56273=CARTESIAN_POINT('Ctrl Pts',(0.0566785527630608,0.808050751452203,
-0.596542209420943));
#56274=CARTESIAN_POINT('Ctrl Pts',(-0.335795913582415,0.737156414668648,
-0.585957793714374));
#56275=CARTESIAN_POINT('Ctrl Pts',(-0.646868640277576,0.48756480337615,
-0.575373378007802));
#56276=CARTESIAN_POINT('Ctrl Pts',(-0.801131142327445,0.11978049949348,
-0.564788962301232));
#56277=CARTESIAN_POINT('Ctrl Pts',(-0.761187979460866,-0.277040313294056,
-0.554204546594661));
#56278=CARTESIAN_POINT('Ctrl Pts',(-0.536721946533164,-0.606702585601409,
-0.54362013088809));
#56279=CARTESIAN_POINT('Ctrl Pts',(-0.18214682534945,-0.789291460286313,
-0.533035715181519));
#56280=CARTESIAN_POINT('Ctrl Pts',(0.216583295509653,-0.780544778582218,
-0.522451299474949));
#56281=CARTESIAN_POINT('Ctrl Pts',(0.56281052303215,-0.582582861428363,
-0.511866883768378));
#56282=CARTESIAN_POINT('Ctrl Pts',(0.772604417642525,-0.24339451330102,
-0.501282468061807));
#56283=CARTESIAN_POINT('Ctrl Pts',(0.795107934038734,0.154796151419981,
-0.490698052355236));
#56284=CARTESIAN_POINT('Ctrl Pts',(0.624865897488736,0.515462011618108,
-0.480113636648666));
#56285=CARTESIAN_POINT('Ctrl Pts',(0.303147416329586,0.751172496327227,
-0.469529220942094));
#56286=CARTESIAN_POINT('Ctrl Pts',(-0.0920583410636652,0.804788007556264,
-0.458944805235524));
#56287=CARTESIAN_POINT('Ctrl Pts',(-0.464947837868951,0.663311377353662,
-0.448360389528953));
#56288=CARTESIAN_POINT('Ctrl Pts',(-0.725127318505599,0.361038567500139,
-0.437775973822382));
#56289=CARTESIAN_POINT('Ctrl Pts',(-0.809525549857519,-0.0287551629084234,
-0.427191558115811));
#56290=CARTESIAN_POINT('Ctrl Pts',(-0.697683191659187,-0.411578229917095,
-0.416607142409241));
#56291=CARTESIAN_POINT('Ctrl Pts',(-0.416712433655251,-0.694628838231777,
-0.40602272670267));
#56292=CARTESIAN_POINT('Ctrl Pts',(-0.034724612422847,-0.80929146576377,
-0.395438310996099));
#56293=CARTESIAN_POINT('Ctrl Pts',(0.355680952278354,-0.727770249082901,
-0.384853895289528));
#56294=CARTESIAN_POINT('Ctrl Pts',(0.659864359109563,-0.469827098887125,
-0.374269479582957));
#56295=CARTESIAN_POINT('Ctrl Pts',(0.804087192872789,-0.0979911297549861,
-0.363685063876387));
#56296=CARTESIAN_POINT('Ctrl Pts',(0.753387772756394,0.297599292924283,
-0.353100648169815));
#56297=CARTESIAN_POINT('Ctrl Pts',(0.520056364353892,0.621047383969223,
-0.342516232463245));
#56298=CARTESIAN_POINT('Ctrl Pts',(0.160655843676387,0.793944692760268,
-0.331931816756674));
#56299=CARTESIAN_POINT('Ctrl Pts',(-0.237689955121348,0.774378434995814,
-0.321347401050103));
#56300=CARTESIAN_POINT('Ctrl Pts',(-0.578416303442509,0.567091751716565,
-0.310762985343532));
#56301=CARTESIAN_POINT('Ctrl Pts',(-0.778926255117071,0.222333904525157,
-0.300178569636961));
#56302=CARTESIAN_POINT('Ctrl Pts',(-0.790613322678065,-0.176320866319888,
-0.289594153930391));
#56303=CARTESIAN_POINT('Ctrl Pts',(-0.610644399274507,-0.532232932794095,
-0.27900973822382));
#56304=CARTESIAN_POINT('Ctrl Pts',(-0.282646518678672,-0.759124113463787,
-0.268425322517249));
#56305=CARTESIAN_POINT('Ctrl Pts',(0.113868912219864,-0.801992732364211,
-0.257840906810678));
#56306=CARTESIAN_POINT('Ctrl Pts',(0.482780916462025,-0.65044682927543,
-0.247256491104107));
#56307=CARTESIAN_POINT('Ctrl Pts',(0.734659854247102,-0.34122328805247,
-0.236672075397537));
#56308=CARTESIAN_POINT('Ctrl Pts',(0.808446830656353,0.0507176480326844,
-0.226087659690966));
#56309=CARTESIAN_POINT('Ctrl Pts',(0.686254496263704,0.430363935274053,
-0.215503243984395));
#56310=CARTESIAN_POINT('Ctrl Pts',(0.39770467014508,0.705683769909671,-0.204918828277824));
#56311=CARTESIAN_POINT('Ctrl Pts',(0.0127446932144949,0.809935887109748,
-0.194334412571253));
#56312=CARTESIAN_POINT('Ctrl Pts',(-0.375303126801014,0.717847673788803,
-0.183749996864682));
#56313=CARTESIAN_POINT('Ctrl Pts',(-0.672375339354181,0.451743430318885,
-0.173165581158112));
#56314=CARTESIAN_POINT('Ctrl Pts',(-0.806447761727482,0.0761290692512524,
-0.162581165451541));
#56315=CARTESIAN_POINT('Ctrl Pts',(-0.745038219657606,-0.317938027158024,
-0.15199674974497));
#56316=CARTESIAN_POINT('Ctrl Pts',(-0.502996112773066,-0.634936413425072,
-0.141412334038399));
#56317=CARTESIAN_POINT('Ctrl Pts',(-0.139069238345838,-0.798009078979888,
-0.130827918331828));
#56318=CARTESIAN_POINT('Ctrl Pts',(0.258669291101841,-0.76765024691656,
-0.120243502625258));
#56319=CARTESIAN_POINT('Ctrl Pts',(0.481866038556668,-0.623315783353716,
-0.113187225487544));
#56320=CARTESIAN_POINT('Ctrl Pts',(0.569564759844983,-0.52886871165407,
-0.109659086918687));
#56321=CARTESIAN_POINT('Ctrl Pts',(0.574972211374301,0.552075258374573,
-1.13659091308131));
#56322=CARTESIAN_POINT('Ctrl Pts',(0.4834253054079,0.647419011186374,-1.13306277451246));
#56323=CARTESIAN_POINT('Ctrl Pts',(0.25208139399889,0.791594820221696,-1.12600649737474));
#56324=CARTESIAN_POINT('Ctrl Pts',(-0.15628601981914,0.815905719349405,
-1.11542208166817));
#56325=CARTESIAN_POINT('Ctrl Pts',(-0.526665958223137,0.642448861628311,
-1.1048376659616));
#56326=CARTESIAN_POINT('Ctrl Pts',(-0.769424319228209,0.31324411891761,
-1.09425325025503));
#56327=CARTESIAN_POINT('Ctrl Pts',(-0.825638018610592,-0.0918909388593417,
-1.08366883454846));
#56328=CARTESIAN_POINT('Ctrl Pts',(-0.681718043703425,-0.474752624954789,
-1.07308441884189));
#56329=CARTESIAN_POINT('Ctrl Pts',(-0.372533329012816,-0.742526299340561,
-1.06250000313532));
#56330=CARTESIAN_POINT('Ctrl Pts',(0.0269554810381316,-0.830301560336992,
-1.05191558742875));
#56331=CARTESIAN_POINT('Ctrl Pts',(0.419911586864664,-0.716799524699605,
-1.04133117172218));
#56332=CARTESIAN_POINT('Ctrl Pts',(0.711074248116431,-0.429535171352737,
-1.0307467560156));
#56333=CARTESIAN_POINT('Ctrl Pts',(0.829862763951438,-0.0381452605230374,
-1.02016234030904));
#56334=CARTESIAN_POINT('Ctrl Pts',(0.747480435038788,0.362491567676058,
-1.00957792460246));
#56335=CARTESIAN_POINT('Ctrl Pts',(0.483898254828331,0.675255267734517,
-0.998993508895893));
#56336=CARTESIAN_POINT('Ctrl Pts',(0.103012148055223,0.824327407596778,
-0.988409093189322));
#56337=CARTESIAN_POINT('Ctrl Pts',(-0.302845549568404,0.773570780867756,
-0.977824677482752));
#56338=CARTESIAN_POINT('Ctrl Pts',(-0.635289162787122,0.535289512933327,
-0.96724026177618));
#56339=CARTESIAN_POINT('Ctrl Pts',(-0.813729574938656,0.167246400542847,
-0.95665584606961));
#56340=CARTESIAN_POINT('Ctrl Pts',(-0.794910285528796,-0.241339635805483,
-0.946071430363038));
#56341=CARTESIAN_POINT('Ctrl Pts',(-0.583393354022263,-0.591421486943936,
-0.935487014656468));
#56342=CARTESIAN_POINT('Ctrl Pts',(-0.230453517535823,-0.798134297854346,
-0.924902598949897));
#56343=CARTESIAN_POINT('Ctrl Pts',(0.178351553307546,-0.811367921785181,
-0.914318183243326));
#56344=CARTESIAN_POINT('Ctrl Pts',(0.543921652523406,-0.627914338866642,
-0.903733767536756));
#56345=CARTESIAN_POINT('Ctrl Pts',(0.777637351750247,-0.292245325456775,
-0.893149351830184));
#56346=CARTESIAN_POINT('Ctrl Pts',(0.822842617371817,0.114268141177551,
-0.882564936123615));
#56347=CARTESIAN_POINT('Ctrl Pts',(0.6685790455489,0.493081373532255,-0.871980520417042));
#56348=CARTESIAN_POINT('Ctrl Pts',(0.352242335828867,0.7523646176642,-0.861396104710473));
#56349=CARTESIAN_POINT('Ctrl Pts',(-0.0494829618762249,0.829263901028745,
-0.850811689003901));
#56350=CARTESIAN_POINT('Ctrl Pts',(-0.439212880795219,0.705137735771633,
-0.840227273297331));
#56351=CARTESIAN_POINT('Ctrl Pts',(-0.72247130578532,0.410076082430725,
-0.829642857590759));
#56352=CARTESIAN_POINT('Ctrl Pts',(-0.830592337021733,0.0156061124644064,
-0.81905844188419));
#56353=CARTESIAN_POINT('Ctrl Pts',(-0.737365887722473,-0.382647002717086,
-0.808474026177617));
#56354=CARTESIAN_POINT('Ctrl Pts',(-0.465391384645681,-0.688141003111179,
-0.797889610471048));
#56355=CARTESIAN_POINT('Ctrl Pts',(-0.0805993433078604,-0.826819766892139,
-0.787305194764476));
#56356=CARTESIAN_POINT('Ctrl Pts',(0.32373113341445,-0.765065575178645,
-0.776720779057906));
#56357=CARTESIAN_POINT('Ctrl Pts',(0.649584546024354,-0.51784852865638,
-0.766136363351335));
#56358=CARTESIAN_POINT('Ctrl Pts',(0.817969359531213,-0.145097580728735,
-0.755551947644763));
#56359=CARTESIAN_POINT('Ctrl Pts',(0.788066683067918,0.262827099256472,
-0.744967531938194));
#56360=CARTESIAN_POINT('Ctrl Pts',(0.567125353758002,0.607038725445171,
-0.734383116231622));
#56361=CARTESIAN_POINT('Ctrl Pts',(0.208704714759074,0.804095468898175,
-0.723798700525051));
#56362=CARTESIAN_POINT('Ctrl Pts',(-0.20030893674369,0.806227952210694,
-0.713214284818481));
#56363=CARTESIAN_POINT('Ctrl Pts',(-0.560764832601105,0.612919230880461,
-0.702629869111909));
#56364=CARTESIAN_POINT('Ctrl Pts',(-0.785283300210914,0.271030108060145,
-0.69204545340534));
#56365=CARTESIAN_POINT('Ctrl Pts',(-0.819437846849956,-0.136560595396867,
-0.681461037698767));
#56366=CARTESIAN_POINT('Ctrl Pts',(-0.654948921157034,-0.511047054331084,
-0.670876621992198));
#56367=CARTESIAN_POINT('Ctrl Pts',(-0.331690994985504,-0.761648386665898,
-0.660292206285627));
#56368=CARTESIAN_POINT('Ctrl Pts',(0.0719735797664497,-0.827615239637865,
-0.649707790579055));
#56369=CARTESIAN_POINT('Ctrl Pts',(0.458190727778319,-0.692956303126838,
-0.639123374872485));
#56370=CARTESIAN_POINT('Ctrl Pts',(0.733335879901691,-0.390314832300863,
-0.628538959165914));
#56371=CARTESIAN_POINT('Ctrl Pts',(0.830709909871899,0.00694454504353916,
-0.617954543459344));
#56372=CARTESIAN_POINT('Ctrl Pts',(0.726707957963954,0.402520465190403,
-0.607370127752772));
#56373=CARTESIAN_POINT('Ctrl Pts',(0.446541587123986,0.700519658563577,
-0.596785712046202));
#56374=CARTESIAN_POINT('Ctrl Pts',(0.0581271389613474,0.828702851920643,
-0.586201296339631));
#56375=CARTESIAN_POINT('Ctrl Pts',(-0.344378160343194,0.755996602997577,
-0.575616880633061));
#56376=CARTESIAN_POINT('Ctrl Pts',(-0.66340126044393,0.500025948033344,
-0.565032464926489));
#56377=CARTESIAN_POINT('Ctrl Pts',(-0.821606391945131,0.122841840511051,
-0.554448049219919));
#56378=CARTESIAN_POINT('Ctrl Pts',(-0.780642364719396,-0.284120888831762,
-0.543863633513348));
#56379=CARTESIAN_POINT('Ctrl Pts',(-0.55043944576635,-0.622208644756461,
-0.533279217806777));
#56380=CARTESIAN_POINT('Ctrl Pts',(-0.186802120243198,-0.809464112198859,
-0.522694802100206));
#56381=CARTESIAN_POINT('Ctrl Pts',(0.222118715123597,-0.800493883460131,
-0.512110386393635));
#56382=CARTESIAN_POINT('Ctrl Pts',(0.577194792145775,-0.597472470482978,
-0.501525970687065));
#56383=CARTESIAN_POINT('Ctrl Pts',(0.792350583371397,-0.249615172007328,
-0.490941554980493));
#56384=CARTESIAN_POINT('Ctrl Pts',(0.815429242950966,0.158752419841869,
-0.480357139273923));
#56385=CARTESIAN_POINT('Ctrl Pts',(0.640836173206008,0.528636151030106,
-0.469772723567352));
#56386=CARTESIAN_POINT('Ctrl Pts',(0.310895235247563,0.770370906619402,
-0.459188307860781));
#56387=CARTESIAN_POINT('Ctrl Pts',(-0.0944111612363924,0.825356719061053,
-0.44860389215421));
#56388=CARTESIAN_POINT('Ctrl Pts',(-0.476830939818917,0.680264239760323,
-0.43801947644764));
#56389=CARTESIAN_POINT('Ctrl Pts',(-0.743660068097472,0.370265964115506,
-0.427435060741068));
#56390=CARTESIAN_POINT('Ctrl Pts',(-0.830215343112932,-0.0294900852042113,
-0.416850645034498));
#56391=CARTESIAN_POINT('Ctrl Pts',(-0.715514526316563,-0.422097315431953,
-0.406266229327927));
#56392=CARTESIAN_POINT('Ctrl Pts',(-0.427362738763972,-0.712382109953456,
-0.395681813621356));
#56393=CARTESIAN_POINT('Ctrl Pts',(-0.0356121014613704,-0.829975276315482,
-0.385097397914786));
#56394=CARTESIAN_POINT('Ctrl Pts',(0.364771419365924,-0.746370546496139,
-0.374512982208215));
#56395=CARTESIAN_POINT('Ctrl Pts',(0.676729122882608,-0.481834904624049,
-0.363928566501644));
#56396=CARTESIAN_POINT('Ctrl Pts',(0.824637993008488,-0.100495579695883,
-0.353344150795073));
#56397=CARTESIAN_POINT('Ctrl Pts',(0.772642800917309,0.305205313320604,
-0.342759735088502));
#56398=CARTESIAN_POINT('Ctrl Pts',(0.533347925888346,0.63692006640451,-0.332175319381932));
#56399=CARTESIAN_POINT('Ctrl Pts',(0.164761873673246,0.814236271639195,
-0.321590903675361));
#56400=CARTESIAN_POINT('Ctrl Pts',(-0.243764817157777,0.794169940927079,
-0.311006487968789));
#56401=CARTESIAN_POINT('Ctrl Pts',(-0.593199423920784,0.581585440151637,
-0.300422072262219));
#56402=CARTESIAN_POINT('Ctrl Pts',(-0.798833993893717,0.228016297772788,
-0.289837656555648));
#56403=CARTESIAN_POINT('Ctrl Pts',(-0.810819758650425,-0.180827261789946,
-0.279253240849078));
#56404=CARTESIAN_POINT('Ctrl Pts',(-0.626251203007618,-0.545835702150998,
-0.268668825142506));
#56405=CARTESIAN_POINT('Ctrl Pts',(-0.289870377192901,-0.778525750590038,
-0.258084409435936));
#56406=CARTESIAN_POINT('Ctrl Pts',(0.116779165333508,-0.822490002435403,
-0.247499993729365));
#56407=CARTESIAN_POINT('Ctrl Pts',(0.495119794896455,-0.667070900527678,
-0.236915578022794));
#56408=CARTESIAN_POINT('Ctrl Pts',(0.753436235672123,-0.349944247242678,
-0.226331162316223));
#56409=CARTESIAN_POINT('Ctrl Pts',(0.829109054087371,0.0520138858751856,
-0.215746746609652));
#56410=CARTESIAN_POINT('Ctrl Pts',(0.703793737181786,0.44136314443672,-0.205162330903082));
#56411=CARTESIAN_POINT('Ctrl Pts',(0.407869176260375,0.723719582745598,
-0.194577915196511));
#56412=CARTESIAN_POINT('Ctrl Pts',(0.0130704211272931,0.830636167733862,
-0.18399349948994));
#56413=CARTESIAN_POINT('Ctrl Pts',(-0.384895095952561,0.736194370767277,
-0.173409083783369));
#56414=CARTESIAN_POINT('Ctrl Pts',(-0.689559857821479,0.463289055011564,
-0.162824668076798));
#56415=CARTESIAN_POINT('Ctrl Pts',(-0.827058893104828,0.0780747702903524,
-0.152240252370228));
#56416=CARTESIAN_POINT('Ctrl Pts',(-0.764079850566983,-0.326063863397647,
-0.141655836663657));
#56417=CARTESIAN_POINT('Ctrl Pts',(-0.515851649677841,-0.651164070632938,
-0.131071420957086));
#56418=CARTESIAN_POINT('Ctrl Pts',(-0.142623559503546,-0.818404535136822,
-0.120487005250515));
#56419=CARTESIAN_POINT('Ctrl Pts',(0.265280341432943,-0.787269794321785,
-0.109902589543944));
#56420=CARTESIAN_POINT('Ctrl Pts',(0.494181534610247,-0.639246441370247,
-0.10284631240623));
#56421=CARTESIAN_POINT('Ctrl Pts',(0.584121653236224,-0.542385498499533,
-0.0993181738373734));
#56422=CARTESIAN_POINT('Ctrl Pts',(0.589301091561382,0.565833523687245,
-1.12625));
#56423=CARTESIAN_POINT('Ctrl Pts',(0.495472745516417,0.663553337782706,
-1.12272186143114));
#56424=CARTESIAN_POINT('Ctrl Pts',(0.258363513413617,0.811322151580129,
-1.11566558429343));
#56425=CARTESIAN_POINT('Ctrl Pts',(-0.160180823095895,0.836238902528063,
-1.10508116858686));
#56426=CARTESIAN_POINT('Ctrl Pts',(-0.539790998468049,0.658459327147326,
-1.09449675288029));
#56427=CARTESIAN_POINT('Ctrl Pts',(-0.788599139619781,0.321050474356163,
-1.08391233717372));
#56428=CARTESIAN_POINT('Ctrl Pts',(-0.846213740380333,-0.0941809525802601,
-1.07332792146715));
#56429=CARTESIAN_POINT('Ctrl Pts',(-0.698707136352355,-0.486583933228312,
-1.06274350576058));
#56430=CARTESIAN_POINT('Ctrl Pts',(-0.381817230619748,-0.761030794285765,
-1.052159090054));
#56431=CARTESIAN_POINT('Ctrl Pts',(0.0276272384736035,-0.8509935022115,
-1.04157467434743));
#56432=CARTESIAN_POINT('Ctrl Pts',(0.430376201846611,-0.734662882796562,
-1.03099025864086));
#56433=CARTESIAN_POINT('Ctrl Pts',(0.728794926618486,-0.44023961564534,
-1.02040584293429));
#56434=CARTESIAN_POINT('Ctrl Pts',(0.850543770582973,-0.0390958784084376,
-1.00982142722772));
#56435=CARTESIAN_POINT('Ctrl Pts',(0.766108391979974,0.371525218588757,
-0.99923701152115));
#56436=CARTESIAN_POINT('Ctrl Pts',(0.495957481307468,0.692083301569292,
-0.988652595814579));
#56437=CARTESIAN_POINT('Ctrl Pts',(0.10557931338617,0.844870467634672,-0.978068180108009));
#56438=CARTESIAN_POINT('Ctrl Pts',(-0.310392762301666,0.792848935213314,
-0.967483764401438));
#56439=CARTESIAN_POINT('Ctrl Pts',(-0.651121201479862,0.548629460750789,
-0.956899348694867));
#56440=CARTESIAN_POINT('Ctrl Pts',(-0.834008526431131,0.171414347423916,
-0.946314932988296));
#56441=CARTESIAN_POINT('Ctrl Pts',(-0.814720241584927,-0.247354059907101,
-0.935730517281725));
#56442=CARTESIAN_POINT('Ctrl Pts',(-0.597932097471697,-0.6061602994619,
-0.925146101575155));
#56443=CARTESIAN_POINT('Ctrl Pts',(-0.23619664872745,-0.818024599508785,
-0.914561685868583));
#56444=CARTESIAN_POINT('Ctrl Pts',(0.182796251656384,-0.831588018528836,
-0.903977270162014));
#56445=CARTESIAN_POINT('Ctrl Pts',(0.557476721857172,-0.643562589601865,
-0.893392854455442));
#56446=CARTESIAN_POINT('Ctrl Pts',(0.797016849092552,-0.299528370047219,
-0.882808438748871));
#56447=CARTESIAN_POINT('Ctrl Pts',(0.843348674958435,0.117115817068216,
-0.872224023042301));
#56448=CARTESIAN_POINT('Ctrl Pts',(0.685240701277209,0.505369452475996,
-0.86163960733573));
#56449=CARTESIAN_POINT('Ctrl Pts',(0.361020565675569,0.771114293301118,
-0.851055191629159));
#56450=CARTESIAN_POINT('Ctrl Pts',(-0.0507161265718399,0.849929983399771,
-0.840470775922588));
#56451=CARTESIAN_POINT('Ctrl Pts',(-0.450158503246249,0.722710470473214,
-0.829886360216016));
#56452=CARTESIAN_POINT('Ctrl Pts',(-0.740476010316099,0.420295586845891,
-0.819301944509447));
#56453=CARTESIAN_POINT('Ctrl Pts',(-0.851291525340843,0.0159950323309065,
-0.808717528802875));
#56454=CARTESIAN_POINT('Ctrl Pts',(-0.755741780070319,-0.392182947146076,
-0.798133113096306));
#56455=CARTESIAN_POINT('Ctrl Pts',(-0.476989401486788,-0.705290162305898,
-0.787548697389734));
#56456=CARTESIAN_POINT('Ctrl Pts',(-0.0826079592210633,-0.847424939006094,
-0.776964281683164));
#56457=CARTESIAN_POINT('Ctrl Pts',(0.331798835699463,-0.784131771327138,
-0.766379865976592));
#56458=CARTESIAN_POINT('Ctrl Pts',(0.66577283990575,-0.530753829774217,
-0.755795450270022));
#56459=CARTESIAN_POINT('Ctrl Pts',(0.838353970678613,-0.148713556959531,
-0.74521103456345));
#56460=CARTESIAN_POINT('Ctrl Pts',(0.807706089734409,0.269377012349076,
-0.73462661885688));
#56461=CARTESIAN_POINT('Ctrl Pts',(0.581258682437715,0.622166735101554,
-0.72404220315031));
#56462=CARTESIAN_POINT('Ctrl Pts',(0.213905844123421,0.824134328872429,
-0.713457787443737));
#56463=CARTESIAN_POINT('Ctrl Pts',(-0.205300834957591,0.826319955793078,
-0.702873371737168));
#56464=CARTESIAN_POINT('Ctrl Pts',(-0.574739650758427,0.628193788589349,
-0.692288956030596));
#56465=CARTESIAN_POINT('Ctrl Pts',(-0.804853342204323,0.277784448302439,
-0.681704540324026));
#56466=CARTESIAN_POINT('Ctrl Pts',(-0.839859054163972,-0.139963821450246,
-0.671120124617455));
#56467=CARTESIAN_POINT('Ctrl Pts',(-0.67127090060972,-0.523782855934378,
-0.660535708910885));
#56468=CARTESIAN_POINT('Ctrl Pts',(-0.339957064948993,-0.780629423073091,
-0.649951293204313));
#56469=CARTESIAN_POINT('Ctrl Pts',(0.0737672330608303,-0.848240235724942,
-0.639366877497742));
#56470=CARTESIAN_POINT('Ctrl Pts',(0.469609297078345,-0.71022546439405,
-0.628782461791172));
#56471=CARTESIAN_POINT('Ctrl Pts',(0.751611340440703,-0.400041866680337,
-0.6181980460846));
#56472=CARTESIAN_POINT('Ctrl Pts',(0.85141202822354,0.00711761002287854,
-0.60761363037803));
#56473=CARTESIAN_POINT('Ctrl Pts',(0.744818244086783,0.41255167609845,-0.597029214671459));
#56474=CARTESIAN_POINT('Ctrl Pts',(0.457669848236215,0.717977306181469,
-0.586444798964888));
#56475=CARTESIAN_POINT('Ctrl Pts',(0.0595757251596351,0.849354952389083,
-0.575860383258318));
#56476=CARTESIAN_POINT('Ctrl Pts',(-0.352960407103974,0.774836791326507,
-0.565275967551747));
#56477=CARTESIAN_POINT('Ctrl Pts',(-0.679933880610282,0.512487092690538,
-0.554691551845177));
#56478=CARTESIAN_POINT('Ctrl Pts',(-0.842081641562818,0.125903181528622,
-0.544107136138605));
#56479=CARTESIAN_POINT('Ctrl Pts',(-0.800096749977925,-0.291201464369467,
-0.533522720432035));
#56480=CARTESIAN_POINT('Ctrl Pts',(-0.564156944999535,-0.637714703911514,
-0.522938304725464));
#56481=CARTESIAN_POINT('Ctrl Pts',(-0.191457415136946,-0.829636764111403,
-0.512353889018893));
#56482=CARTESIAN_POINT('Ctrl Pts',(0.227654134737541,-0.820442988338044,
-0.501769473312322));
#56483=CARTESIAN_POINT('Ctrl Pts',(0.591579061259401,-0.612362079537592,
-0.491185057605751));
#56484=CARTESIAN_POINT('Ctrl Pts',(0.812096749100268,-0.255835830713636,
-0.48060064189918));
#56485=CARTESIAN_POINT('Ctrl Pts',(0.8357505518632,0.162708688263756,-0.47001622619261));
#56486=CARTESIAN_POINT('Ctrl Pts',(0.656806448923279,0.541810290442105,
-0.459431810486038));
#56487=CARTESIAN_POINT('Ctrl Pts',(0.318643054165541,0.789569316911576,
-0.448847394779468));
#56488=CARTESIAN_POINT('Ctrl Pts',(-0.0967639814091197,0.845925430565842,
-0.438262979072897));
#56489=CARTESIAN_POINT('Ctrl Pts',(-0.488714041768884,0.697217102166983,
-0.427678563366326));
#56490=CARTESIAN_POINT('Ctrl Pts',(-0.762192817689344,0.379493360730874,
-0.417094147659756));
#56491=CARTESIAN_POINT('Ctrl Pts',(-0.850905136368346,-0.0302250075,-0.406509731953184));
#56492=CARTESIAN_POINT('Ctrl Pts',(-0.733345860973939,-0.43261640094681,
-0.395925316246614));
#56493=CARTESIAN_POINT('Ctrl Pts',(-0.438013043872693,-0.730135381675136,
-0.385340900540043));
#56494=CARTESIAN_POINT('Ctrl Pts',(-0.0364995904998943,-0.850659086867193,
-0.374756484833472));
#56495=CARTESIAN_POINT('Ctrl Pts',(0.373861886453494,-0.764970843909378,
-0.364172069126902));
#56496=CARTESIAN_POINT('Ctrl Pts',(0.693593886655655,-0.493842710360973,
-0.35358765342033));
#56497=CARTESIAN_POINT('Ctrl Pts',(0.845188793144186,-0.10300002963678,
-0.34300323771376));
#56498=CARTESIAN_POINT('Ctrl Pts',(0.791897829078223,0.312811333716926,
-0.332418822007189));
#56499=CARTESIAN_POINT('Ctrl Pts',(0.5466394874228,0.652792748839794,-0.321834406300618));
#56500=CARTESIAN_POINT('Ctrl Pts',(0.168867903670105,0.834527850518125,
-0.311249990594047));
#56501=CARTESIAN_POINT('Ctrl Pts',(-0.249839679194206,0.813961446858341,
-0.300665574887477));
#56502=CARTESIAN_POINT('Ctrl Pts',(-0.607982544399059,0.59607912858671,
-0.290081159180906));
#56503=CARTESIAN_POINT('Ctrl Pts',(-0.818741732670364,0.233698691020418,
-0.279496743474335));
#56504=CARTESIAN_POINT('Ctrl Pts',(-0.831026194622783,-0.185333657260002,
-0.268912327767764));
#56505=CARTESIAN_POINT('Ctrl Pts',(-0.64185800674073,-0.559438471507901,
-0.258327912061193));
#56506=CARTESIAN_POINT('Ctrl Pts',(-0.29709423570713,-0.797927387716288,
-0.247743496354622));
#56507=CARTESIAN_POINT('Ctrl Pts',(0.119689418447152,-0.842987272506594,
-0.237159080648052));
#56508=CARTESIAN_POINT('Ctrl Pts',(0.507458673330886,-0.683694971779928,
-0.226574664941481));
#56509=CARTESIAN_POINT('Ctrl Pts',(0.772212617097144,-0.358665206432886,
-0.21599024923491));
#56510=CARTESIAN_POINT('Ctrl Pts',(0.849771277518388,0.0533101237176862,
-0.205405833528339));
#56511=CARTESIAN_POINT('Ctrl Pts',(0.721332978099869,0.452362353599387,
-0.194821417821768));
#56512=CARTESIAN_POINT('Ctrl Pts',(0.41803368237567,0.741755395581526,-0.184237002115198));
#56513=CARTESIAN_POINT('Ctrl Pts',(0.0133961490400916,0.851336448357975,
-0.173652586408627));
#56514=CARTESIAN_POINT('Ctrl Pts',(-0.394487065104108,0.754541067745753,
-0.163068170702056));
#56515=CARTESIAN_POINT('Ctrl Pts',(-0.706744376288777,0.474834679704242,
-0.152483754995485));
#56516=CARTESIAN_POINT('Ctrl Pts',(-0.847670024482175,0.0800204713294527,
-0.141899339288914));
#56517=CARTESIAN_POINT('Ctrl Pts',(-0.783121481476359,-0.334189699637271,
-0.131314923582344));
#56518=CARTESIAN_POINT('Ctrl Pts',(-0.528707186582616,-0.667391727840805,
-0.120730507875773));
#56519=CARTESIAN_POINT('Ctrl Pts',(-0.146177880661253,-0.838799991293755,
-0.110146092169202));
#56520=CARTESIAN_POINT('Ctrl Pts',(0.271891391764045,-0.80688934172701,
-0.0995616764626311));
#56521=CARTESIAN_POINT('Ctrl Pts',(0.506497030663827,-0.655177099386778,
-0.0925053993249171));
#56522=CARTESIAN_POINT('Ctrl Pts',(0.598678546627464,-0.555902285344995,
-0.0889772607560602));
#56523=CARTESIAN_POINT('',(0.555007866453742,-0.515351924808608,-0.12));
#56524=CARTESIAN_POINT('Ctrl Pts',(-0.485074560134029,-0.65745190369334,
-0.12));
#56525=CARTESIAN_POINT('Ctrl Pts',(-0.453585509292985,-0.678311536271589,
-0.12));
#56526=CARTESIAN_POINT('Ctrl Pts',(-0.420738538427663,-0.696888835579881,
-0.12));
#56527=CARTESIAN_POINT('Ctrl Pts',(-0.386803943986794,-0.71311112212273,
-0.12));
#56528=CARTESIAN_POINT('Ctrl Pts',(-0.352869989072943,-0.729333102942445,
-0.12));
#56529=CARTESIAN_POINT('Ctrl Pts',(-0.317847265091438,-0.743200535649333,
-0.12));
#56530=CARTESIAN_POINT('Ctrl Pts',(-0.281986661942266,-0.754592743143696,
-0.12));
#56531=CARTESIAN_POINT('Ctrl Pts',(-0.255949172785094,-0.762864340748367,
-0.12));
#56532=CARTESIAN_POINT('Ctrl Pts',(-0.229469505293985,-0.7698300648233,
-0.12));
#56533=CARTESIAN_POINT('Ctrl Pts',(-0.202642618159761,-0.775426102639775,
-0.12));
#56534=CARTESIAN_POINT('Ctrl Pts',(-0.195274171519276,-0.776963146645012,
-0.12));
#56535=CARTESIAN_POINT('Ctrl Pts',(-0.187880255141526,-0.778396492216609,
-0.12));
#56536=CARTESIAN_POINT('Ctrl Pts',(-0.18047576779481,-0.779722738931636,
-0.12));
#56537=CARTESIAN_POINT('Ctrl Pts',(-0.166033419362242,-0.782309564496876,
-0.12));
#56538=CARTESIAN_POINT('Ctrl Pts',(-0.151538081932198,-0.784491790553693,
-0.12));
#56539=CARTESIAN_POINT('Ctrl Pts',(-0.137004865545485,-0.786263720842401,
-0.12));
#56540=CARTESIAN_POINT('Ctrl Pts',(-0.100095238310147,-0.790763845570678,
-0.12));
#56541=CARTESIAN_POINT('Ctrl Pts',(-0.0629412165342028,-0.792621345331591,
-0.12));
#56542=CARTESIAN_POINT('Ctrl Pts',(-0.0258198641282066,-0.791883010674466,
-0.12));
#56543=CARTESIAN_POINT('Ctrl Pts',(0.00402572525169566,-0.791289389171658,
-0.12));
#56544=CARTESIAN_POINT('Ctrl Pts',(0.0338506107991278,-0.789016694488355,
-0.12));
#56545=CARTESIAN_POINT('Ctrl Pts',(0.0635063571289652,-0.78506522308076,
-0.12));
#56546=CARTESIAN_POINT('Ctrl Pts',(0.0773427424639829,-0.78322159788827,
-0.12));
#56547=CARTESIAN_POINT('Ctrl Pts',(0.0911422070269432,-0.781012233182779,
-0.12));
#56548=CARTESIAN_POINT('Ctrl Pts',(0.104888951407889,-0.778435636705529,
-0.12));
#56549=CARTESIAN_POINT('Ctrl Pts',(0.112442728465956,-0.777019807995953,
-0.12));
#56550=CARTESIAN_POINT('Ctrl Pts',(0.119978617797336,-0.775493331514514,
-0.12));
#56551=CARTESIAN_POINT('Ctrl Pts',(0.127482778712085,-0.773858786233986,
-0.12));
#56552=CARTESIAN_POINT('Ctrl Pts',(0.163232326165741,-0.766071872449056,
-0.12));
#56553=CARTESIAN_POINT('Ctrl Pts',(0.198335071471806,-0.755823166547615,
-0.12));
#56554=CARTESIAN_POINT('Ctrl Pts',(0.232522340410342,-0.743135834971473,
-0.12));
#56555=CARTESIAN_POINT('Ctrl Pts',(0.237813230372167,-0.741172318219104,
-0.12));
#56556=CARTESIAN_POINT('Ctrl Pts',(0.243082158223076,-0.739150297995532,
-0.12));
#56557=CARTESIAN_POINT('Ctrl Pts',(0.248328083260998,-0.73706975670363,
-0.12));
#56558=CARTESIAN_POINT('Ctrl Pts',(0.277906408593185,-0.725338951029883,
-0.12));
#56559=CARTESIAN_POINT('Ctrl Pts',(0.306754972760517,-0.711749564176307,
-0.12));
#56560=CARTESIAN_POINT('Ctrl Pts',(0.334717544680486,-0.696396977944506,
-0.12));
#56561=CARTESIAN_POINT('Ctrl Pts',(0.341939489339631,-0.692431837382394,
-0.12));
#56562=CARTESIAN_POINT('Ctrl Pts',(0.349102230975186,-0.688348968720245,
-0.12));
#56563=CARTESIAN_POINT('Ctrl Pts',(0.356202844476414,-0.684149788320379,
-0.12));
#56564=CARTESIAN_POINT('Ctrl Pts',(0.363162967541051,-0.680033691542456,
-0.12));
#56565=CARTESIAN_POINT('Ctrl Pts',(0.370055970531007,-0.675810190952825,
-0.12));
#56566=CARTESIAN_POINT('Ctrl Pts',(0.376876658708298,-0.671483106796323,
-0.12));
#56567=CARTESIAN_POINT('Ctrl Pts',(0.40745623441888,-0.652083246528505,
-0.12));
#56568=CARTESIAN_POINT('Ctrl Pts',(0.436604118212131,-0.630593159071821,
-0.12));
#56569=CARTESIAN_POINT('Ctrl Pts',(0.46410233189715,-0.60717227783143,-0.12));
#56570=CARTESIAN_POINT('Ctrl Pts',(0.491112633055654,-0.58416696327003,
-0.12));
#56571=CARTESIAN_POINT('Ctrl Pts',(0.516532076721098,-0.559297921856729,
-0.12));
#56572=CARTESIAN_POINT('Ctrl Pts',(0.540116340216444,-0.532683959290642,
-0.12));
#56573=CARTESIAN_POINT('Ctrl Pts',(0.545165350086534,-0.52698633978665,
-0.12));
#56574=CARTESIAN_POINT('Ctrl Pts',(0.550130085791934,-0.521208653511241,
-0.12));
#56575=CARTESIAN_POINT('Ctrl Pts',(0.555007866453742,-0.515351924808608,
-0.12));
#56576=CARTESIAN_POINT('',(-0.459778808448974,0.601851132366397,-1.12625));
#56577=CARTESIAN_POINT('Ctrl Pts',(-0.459817636075317,0.601890711574512,
-1.12625));
#56578=CARTESIAN_POINT('Ctrl Pts',(-0.432503985120066,0.625165263761577,
-1.12625));
#56579=CARTESIAN_POINT('Ctrl Pts',(-0.403593713495987,0.646405611026664,
-1.12625));
#56580=CARTESIAN_POINT('Ctrl Pts',(-0.373360039769222,0.665530294930177,
-1.12625));
#56581=CARTESIAN_POINT('Ctrl Pts',(-0.342830078355013,0.684842399271513,
-1.12625));
#56582=CARTESIAN_POINT('Ctrl Pts',(-0.310949650189556,0.701997871851442,
-1.12625));
#56583=CARTESIAN_POINT('Ctrl Pts',(-0.277963229106153,0.716874587570175,
-1.12625));
#56584=CARTESIAN_POINT('Ctrl Pts',(-0.26649732981671,0.722045652468588,
-1.12625));
#56585=CARTESIAN_POINT('Ctrl Pts',(-0.254897548952348,0.726941007906439,
-1.12625));
#56586=CARTESIAN_POINT('Ctrl Pts',(-0.243173471026141,0.731554211541609,
-1.12625));
#56587=CARTESIAN_POINT('Ctrl Pts',(-0.235772847930162,0.734466217209243,
-1.12625));
#56588=CARTESIAN_POINT('Ctrl Pts',(-0.228323386851445,0.737265362586449,
-1.12625));
#56589=CARTESIAN_POINT('Ctrl Pts',(-0.220840169223985,0.739945834211391,
-1.12625));
#56590=CARTESIAN_POINT('Ctrl Pts',(-0.196274161499892,0.748745322602708,
-1.12625));
#56591=CARTESIAN_POINT('Ctrl Pts',(-0.171310177385804,0.756280719952739,
-1.12625));
#56592=CARTESIAN_POINT('Ctrl Pts',(-0.146041756546086,0.762513765607057,
-1.12625));
#56593=CARTESIAN_POINT('Ctrl Pts',(-0.114363689392244,0.770327900097808,
-1.12625));
#56594=CARTESIAN_POINT('Ctrl Pts',(-0.0822071438969164,0.77609639727171,
-1.12625));
#56595=CARTESIAN_POINT('Ctrl Pts',(-0.0497689197316119,0.779842549380837,
-1.12625));
#56596=CARTESIAN_POINT('Ctrl Pts',(-0.0298100993332151,0.782147508393085,
-1.12625));
#56597=CARTESIAN_POINT('Ctrl Pts',(-0.00974437858899013,0.783686221448935,
-1.12625));
#56598=CARTESIAN_POINT('Ctrl Pts',(0.0103835877245399,0.784457979579496,
-1.12625));
#56599=CARTESIAN_POINT('Ctrl Pts',(0.0199668006274251,0.784825424673526,
-1.12625));
#56600=CARTESIAN_POINT('Ctrl Pts',(0.0295667334923406,0.785018756675102,
-1.12625));
#56601=CARTESIAN_POINT('Ctrl Pts',(0.0391548342268405,0.785038051041722,
-1.12625));
#56602=CARTESIAN_POINT('Ctrl Pts',(0.0764066796303495,0.785113013829703,
-1.12625));
#56603=CARTESIAN_POINT('Ctrl Pts',(0.11355304850067,0.782569361975542,-1.12625));
#56604=CARTESIAN_POINT('Ctrl Pts',(0.150309494084269,0.77745070961784,-1.12625));
#56605=CARTESIAN_POINT('Ctrl Pts',(0.181105692018343,0.773162073198822,
-1.12625));
#56606=CARTESIAN_POINT('Ctrl Pts',(0.211628935934584,0.767064947824248,
-1.12625));
#56607=CARTESIAN_POINT('Ctrl Pts',(0.241714208481684,0.759156929049666,
-1.12625));
#56608=CARTESIAN_POINT('Ctrl Pts',(0.258311234815863,0.754794342815906,
-1.12625));
#56609=CARTESIAN_POINT('Ctrl Pts',(0.274774951161081,0.74988017519975,-1.12625));
#56610=CARTESIAN_POINT('Ctrl Pts',(0.291082790748006,0.744427662964972,
-1.12625));
#56611=CARTESIAN_POINT('Ctrl Pts',(0.302253486659231,0.740692750329715,
-1.12625));
#56612=CARTESIAN_POINT('Ctrl Pts',(0.313351031748266,0.736705191681207,
-1.12625));
#56613=CARTESIAN_POINT('Ctrl Pts',(0.324367932128155,0.73246863871898,-1.12625));
#56614=CARTESIAN_POINT('Ctrl Pts',(0.331410788641081,0.729760305740237,
-1.12625));
#56615=CARTESIAN_POINT('Ctrl Pts',(0.338411390394597,0.72695377103039,-1.12625));
#56616=CARTESIAN_POINT('Ctrl Pts',(0.345367277999311,0.724051012762939,
-1.12625));
#56617=CARTESIAN_POINT('Ctrl Pts',(0.379999812823563,0.709598525532449,
-1.12625));
#56618=CARTESIAN_POINT('Ctrl Pts',(0.413530302276288,0.692762730520224,
-1.12625));
#56619=CARTESIAN_POINT('Ctrl Pts',(0.445738862386879,0.673721922806075,
-1.12625));
#56620=CARTESIAN_POINT('Ctrl Pts',(0.47805582561834,0.654617030172481,-1.12625));
#56621=CARTESIAN_POINT('Ctrl Pts',(0.509043040540198,0.63329174243941,-1.12625));
#56622=CARTESIAN_POINT('Ctrl Pts',(0.538461112130946,0.609877570946476,
-1.12625));
#56623=CARTESIAN_POINT('Ctrl Pts',(0.555983532413065,0.595931281088856,
-1.12625));
#56624=CARTESIAN_POINT('Ctrl Pts',(0.57294884620607,0.581243006920529,-1.12625));
#56625=CARTESIAN_POINT('Ctrl Pts',(0.589301091561381,0.565833523687246,
-1.12625));
#56626=CARTESIAN_POINT('Ctrl Pts',(-0.459817636075315,0.601890711574514,
-1.12625));
#56627=CARTESIAN_POINT('Ctrl Pts',(-0.466706837362038,0.596634000305894,
-1.12600649737474));
#56628=CARTESIAN_POINT('Ctrl Pts',(-0.571995661495492,0.513358547689718,
-1.12223485618063));
#56629=CARTESIAN_POINT('Ctrl Pts',(-0.731074678445063,0.297631408040504,
-1.11493507641766));
#56630=CARTESIAN_POINT('Ctrl Pts',(-0.78448657507111,-0.0873109114175063,
-1.10435066071109));
#56631=CARTESIAN_POINT('Ctrl Pts',(-0.647739858405566,-0.451090008407739,
-1.09376624500452));
#56632=CARTESIAN_POINT('Ctrl Pts',(-0.35396552579895,-0.705517309450156,
-1.08318182929794));
#56633=CARTESIAN_POINT('Ctrl Pts',(0.0256119661671881,-0.788917676587972,
-1.07259741359137));
#56634=CARTESIAN_POINT('Ctrl Pts',(0.398982356900771,-0.681072808505694,
-1.0620129978848));
#56635=CARTESIAN_POINT('Ctrl Pts',(0.675632891112322,-0.40812628276753,
-1.05142858217823));
#56636=CARTESIAN_POINT('Ctrl Pts',(0.788500750688369,-0.0362440247522399,
-1.04084416647166));
#56637=CARTESIAN_POINT('Ctrl Pts',(0.710224521156417,0.344424265850664,
-1.03025975076509));
#56638=CARTESIAN_POINT('Ctrl Pts',(0.459779801870057,0.641599200064961,
-1.01967533505852));
#56639=CARTESIAN_POINT('Ctrl Pts',(0.097877817393331,0.783241287520996,
-1.00909091935195));
#56640=CARTESIAN_POINT('Ctrl Pts',(-0.287751124101878,0.735014472176637,
-0.998506503645378));
#56641=CARTESIAN_POINT('Ctrl Pts',(-0.603625085401645,0.508609617298406,
-0.987922087938805));
#56642=CARTESIAN_POINT('Ctrl Pts',(-0.773171671953705,0.158910506780707,
-0.977337672232237));
#56643=CARTESIAN_POINT('Ctrl Pts',(-0.755290373416537,-0.229310787602246,
-0.966753256525664));
#56644=CARTESIAN_POINT('Ctrl Pts',(-0.554315867123395,-0.561943861908008,
-0.956168840819094));
#56645=CARTESIAN_POINT('Ctrl Pts',(-0.218967255152568,-0.758353694545465,
-0.945584425112524));
#56646=CARTESIAN_POINT('Ctrl Pts',(0.169462156609868,-0.770927728297873,
-0.935000009405952));
#56647=CARTESIAN_POINT('Ctrl Pts',(0.516811513855876,-0.596617837396196,
-0.924415593699383));
#56648=CARTESIAN_POINT('Ctrl Pts',(0.738878357065632,-0.277679236275888,
-0.91383117799281));
#56649=CARTESIAN_POINT('Ctrl Pts',(0.781830502198587,0.108572789396219,
-0.903246762286241));
#56650=CARTESIAN_POINT('Ctrl Pts',(0.635255734092279,0.468505215644772,
-0.892662346579669));
#56651=CARTESIAN_POINT('Ctrl Pts',(0.334685876135465,0.714865266390365,
-0.882077930873099));
#56652=CARTESIAN_POINT('Ctrl Pts',(-0.0470166324849972,0.787931736286691,
-0.871493515166528));
#56653=CARTESIAN_POINT('Ctrl Pts',(-0.417321635893157,0.669992266368472,
-0.860909099459957));
#56654=CARTESIAN_POINT('Ctrl Pts',(-0.686461896723767,0.389637073600391,
-0.850324683753386));
#56655=CARTESIAN_POINT('Ctrl Pts',(-0.78919396038351,0.0148282727314064,
-0.839740268046816));
#56656=CARTESIAN_POINT('Ctrl Pts',(-0.700614103026785,-0.363575113859107,
-0.829155852340244));
#56657=CARTESIAN_POINT('Ctrl Pts',(-0.442195350963465,-0.65384268472174,
-0.818571436633674));
#56658=CARTESIAN_POINT('Ctrl Pts',(-0.0765821114814538,-0.785609422664232,
-0.807987020927103));
#56659=CARTESIAN_POINT('Ctrl Pts',(0.307595728844424,-0.726933182881658,
-0.797402605220531));
#56660=CARTESIAN_POINT('Ctrl Pts',(0.617207958261566,-0.492037926420706,
-0.786818189513963));
#56661=CARTESIAN_POINT('Ctrl Pts',(0.77720013723641,-0.137865628267142,
-0.776233773807389));
#56662=CARTESIAN_POINT('Ctrl Pts',(0.748787869734938,0.249727273071264,
-0.765649358100821));
#56663=CARTESIAN_POINT('Ctrl Pts',(0.538858696398575,0.576782706132406,
-0.755064942394248));
#56664=CARTESIAN_POINT('Ctrl Pts',(0.198302456030381,0.764017748949666,
-0.744480526687679));
#56665=CARTESIAN_POINT('Ctrl Pts',(-0.19032514031589,0.766043945045929,
-0.733896110981107));
#56666=CARTESIAN_POINT('Ctrl Pts',(-0.532815196286458,0.582370115462682,
-0.723311695274537));
#56667=CARTESIAN_POINT('Ctrl Pts',(-0.746143216224097,0.257521427575559,
-0.712727279567965));
#56668=CARTESIAN_POINT('Ctrl Pts',(-0.778595432221923,-0.129754143290109,
-0.702142863861395));
#56669=CARTESIAN_POINT('Ctrl Pts',(-0.622304962251659,-0.485575451124495,
-0.691558448154824));
#56670=CARTESIAN_POINT('Ctrl Pts',(-0.315158855058528,-0.723686313851513,
-0.680974032448254));
#56671=CARTESIAN_POINT('Ctrl Pts',(0.0683862731776896,-0.786365247463709,
-0.670389616741681));
#56672=CARTESIAN_POINT('Ctrl Pts',(0.435353589178266,-0.658417980592417,
-0.659805201035112));
#56673=CARTESIAN_POINT('Ctrl Pts',(0.696784958823668,-0.370860763541915,
-0.64922078532854));
#56674=CARTESIAN_POINT('Ctrl Pts',(0.789305673168617,0.00659841508485966,
-0.63863636962197));
#56675=CARTESIAN_POINT('Ctrl Pts',(0.690487385718296,0.382458043374312,
-0.6280519539154));
#56676=CARTESIAN_POINT('Ctrl Pts',(0.424285064899528,0.665604363327792,
-0.617467538208828));
#56677=CARTESIAN_POINT('Ctrl Pts',(0.0552299665647739,0.787398650983763,
-0.606883122502257));
#56678=CARTESIAN_POINT('Ctrl Pts',(-0.327213666821637,0.718316226339718,
-0.596298706795687));
#56679=CARTESIAN_POINT('Ctrl Pts',(-0.630336020111223,0.475103658718956,
-0.585714291089115));
#56680=CARTESIAN_POINT('Ctrl Pts',(-0.780655892709758,0.116719158475909,
-0.575129875382546));
#56681=CARTESIAN_POINT('Ctrl Pts',(-0.741733594202337,-0.269959737756351,
-0.564545459675974));
#56682=CARTESIAN_POINT('Ctrl Pts',(-0.52300444729998,-0.591196526446356,
-0.553961043969404));
#56683=CARTESIAN_POINT('Ctrl Pts',(-0.177491530455701,-0.76911880837377,
-0.543376628262832));
#56684=CARTESIAN_POINT('Ctrl Pts',(0.211047875895708,-0.760595673704304,
-0.532792212556262));
#56685=CARTESIAN_POINT('Ctrl Pts',(0.548426253918526,-0.567693252373749,
-0.522207796849691));
#56686=CARTESIAN_POINT('Ctrl Pts',(0.752858251913653,-0.237173854594711,
-0.511623381143121));
#56687=CARTESIAN_POINT('Ctrl Pts',(0.7747866251265,0.150839882998094,-0.501038965436549));
#56688=CARTESIAN_POINT('Ctrl Pts',(0.608895621771465,0.502287872206109,
-0.490454549729979));
#56689=CARTESIAN_POINT('Ctrl Pts',(0.295399597411609,0.731974086035053,
-0.479870134023407));
#56690=CARTESIAN_POINT('Ctrl Pts',(-0.0897055208909376,0.784219296051475,
-0.469285718316837));
#56691=CARTESIAN_POINT('Ctrl Pts',(-0.453064735918984,0.646358514947002,
-0.458701302610266));
#56692=CARTESIAN_POINT('Ctrl Pts',(-0.706594568913726,0.351811170884772,
-0.448116886903695));
#56693=CARTESIAN_POINT('Ctrl Pts',(-0.788835756602106,-0.028020240612635,
-0.437532471197125));
#56694=CARTESIAN_POINT('Ctrl Pts',(-0.679851857001812,-0.401059144402238,
-0.426948055490553));
#56695=CARTESIAN_POINT('Ctrl Pts',(-0.40606212854653,-0.676875566510097,
-0.416363639783983));
#56696=CARTESIAN_POINT('Ctrl Pts',(-0.033837123384323,-0.788607655212059,
-0.405779224077412));
#56697=CARTESIAN_POINT('Ctrl Pts',(0.346590485190783,-0.709169951669662,
-0.395194808370841));
#56698=CARTESIAN_POINT('Ctrl Pts',(0.642999595336517,-0.457819293150201,
-0.38461039266427));
#56699=CARTESIAN_POINT('Ctrl Pts',(0.78353639273709,-0.0954866798140887,
-0.3740259769577));
#56700=CARTESIAN_POINT('Ctrl Pts',(0.734132744595481,0.28999327252796,-0.363441561251129));
#56701=CARTESIAN_POINT('Ctrl Pts',(0.506764802819437,0.605174701533939,
-0.352857145544558));
#56702=CARTESIAN_POINT('Ctrl Pts',(0.156549813679528,0.773653113881338,
-0.342272729837987));
#56703=CARTESIAN_POINT('Ctrl Pts',(-0.231615093084919,0.754586929064552,
-0.331688314131416));
#56704=CARTESIAN_POINT('Ctrl Pts',(-0.563633182964234,0.552598063281491,
-0.321103898424845));
#56705=CARTESIAN_POINT('Ctrl Pts',(-0.759018516340423,0.216651511277527,
-0.310519482718275));
#56706=CARTESIAN_POINT('Ctrl Pts',(-0.770406886705707,-0.171814470849831,
-0.299935067011704));
#56707=CARTESIAN_POINT('Ctrl Pts',(-0.595037595541395,-0.518630163437193,
-0.289350651305133));
#56708=CARTESIAN_POINT('Ctrl Pts',(-0.275422660164443,-0.739722476337535,
-0.278766235598562));
#56709=CARTESIAN_POINT('Ctrl Pts',(0.11095865910622,-0.78149546229302,-0.268181819891991));
#56710=CARTESIAN_POINT('Ctrl Pts',(0.470442038027593,-0.63382275802318,
-0.257597404185421));
#56711=CARTESIAN_POINT('Ctrl Pts',(0.715883472822082,-0.332502328862262,
-0.24701298847885));
#56712=CARTESIAN_POINT('Ctrl Pts',(0.787784607225333,0.0494214101901834,
-0.236428572772279));
#56713=CARTESIAN_POINT('Ctrl Pts',(0.668715255345623,0.419364726111387,
-0.225844157065708));
#56714=CARTESIAN_POINT('Ctrl Pts',(0.387540164029785,0.687647957073743,
-0.215259741359137));
#56715=CARTESIAN_POINT('Ctrl Pts',(0.0124189653016963,0.789235606485636,
-0.204675325652567));
#56716=CARTESIAN_POINT('Ctrl Pts',(-0.365711157649466,0.699500976810326,
-0.194090909945995));
#56717=CARTESIAN_POINT('Ctrl Pts',(-0.655190820886885,0.440197805626207,
-0.183506494239425));
#56718=CARTESIAN_POINT('Ctrl Pts',(-0.785836630350135,0.0741833682121523,
-0.172922078532854));
#56719=CARTESIAN_POINT('Ctrl Pts',(-0.72599658874823,-0.309812190918401,
-0.162337662826283));
#56720=CARTESIAN_POINT('Ctrl Pts',(-0.490140575868292,-0.618708756217204,
-0.151753247119713));
#56721=CARTESIAN_POINT('Ctrl Pts',(-0.135514917188131,-0.777613622822956,
-0.141168831413141));
#56722=CARTESIAN_POINT('Ctrl Pts',(0.252058240770739,-0.748030699511335,
-0.130584415706571));
#56723=CARTESIAN_POINT('Ctrl Pts',(0.469550542503088,-0.607385125337185,
-0.123528138568857));
#56724=CARTESIAN_POINT('Ctrl Pts',(0.555007866453742,-0.515351924808608,
-0.12));
#56725=CARTESIAN_POINT('Ctrl Pts',(-0.453782243834438,0.594001620520165,
-1.1425283350431));
#56726=CARTESIAN_POINT('Ctrl Pts',(-0.550881388338772,0.519823594492229,
-1.13905034750894));
#56727=CARTESIAN_POINT('Ctrl Pts',(-0.707932320584141,0.323031319671979,
-1.13209437244062));
#56728=CARTESIAN_POINT('Ctrl Pts',(-0.776614466270609,-0.0485165662670007,
-1.12166040983814));
#56729=CARTESIAN_POINT('Ctrl Pts',(-0.662248238305512,-0.408538693637006,
-1.11122644723566));
#56730=CARTESIAN_POINT('Ctrl Pts',(-0.391780881856498,-0.672308433025162,
-1.10079248463318));
#56731=CARTESIAN_POINT('Ctrl Pts',(-0.0289685614302447,-0.77758653236944,
-1.0903585220307));
#56732=CARTESIAN_POINT('Ctrl Pts',(0.340672665444815,-0.699591456600573,
-1.07992455942822));
#56733=CARTESIAN_POINT('Ctrl Pts',(0.630013764781798,-0.45669036663525,
-1.06949059682573));
#56734=CARTESIAN_POINT('Ctrl Pts',(0.770854889346007,-0.106145976774946,
-1.05905663422326));
#56735=CARTESIAN_POINT('Ctrl Pts',(0.72999817257357,0.269419497799126,-1.04862267162077));
#56736=CARTESIAN_POINT('Ctrl Pts',(0.517074073818034,0.581479511865617,
-1.03818870901829));
#56737=CARTESIAN_POINT('Ctrl Pts',(0.182270729955259,0.756479721113076,
-1.02775474641581));
#56738=CARTESIAN_POINT('Ctrl Pts',(-0.195495525574089,0.753170354596227,
-1.01732078381333));
#56739=CARTESIAN_POINT('Ctrl Pts',(-0.527181654493514,0.572331754114927,
-1.00688682121085));
#56740=CARTESIAN_POINT('Ctrl Pts',(-0.734606108414346,0.256589128857393,
-0.996452858608371));
#56741=CARTESIAN_POINT('Ctrl Pts',(-0.768876998658737,-0.119633940618216,
-0.98601889600589));
#56742=CARTESIAN_POINT('Ctrl Pts',(-0.621916351700691,-0.467658178639452,
-0.97558493340341));
#56743=CARTESIAN_POINT('Ctrl Pts',(-0.328364174807744,-0.705450981188053,
-0.965150970800929));
#56744=CARTESIAN_POINT('Ctrl Pts',(0.0425865250681738,-0.776962359283856,
-0.954717008198449));
#56745=CARTESIAN_POINT('Ctrl Pts',(0.403499180542324,-0.665336403825433,
-0.944283045595967));
#56746=CARTESIAN_POINT('Ctrl Pts',(0.669303286159026,-0.396884404409992,
-0.933849082993487));
#56747=CARTESIAN_POINT('Ctrl Pts',(0.777346315469045,-0.0348830195569247,
-0.923415120391007));
#56748=CARTESIAN_POINT('Ctrl Pts',(0.702161510858138,0.335340620697414,
-0.912981157788526));
#56749=CARTESIAN_POINT('Ctrl Pts',(0.461470637519424,0.626521324425116,
-0.902547195186045));
#56750=CARTESIAN_POINT('Ctrl Pts',(0.112006796904718,0.770025062366403,
-0.892113232583565));
#56751=CARTESIAN_POINT('Ctrl Pts',(-0.26385809865297,0.732026654580473,
-0.881679269981084));
#56752=CARTESIAN_POINT('Ctrl Pts',(-0.577529159980992,0.521482682939164,
-0.871245307378604));
#56753=CARTESIAN_POINT('Ctrl Pts',(-0.75507116928701,0.188020340781937,
-0.860811344776122));
#56754=CARTESIAN_POINT('Ctrl Pts',(-0.754635806007903,-0.189760163171063,
-0.850377382173643));
#56755=CARTESIAN_POINT('Ctrl Pts',(-0.576325689361536,-0.522812412838008,
-0.839943419571161));
#56756=CARTESIAN_POINT('Ctrl Pts',(-0.262170190030731,-0.732632862145289,
-0.829509456968681));
#56757=CARTESIAN_POINT('Ctrl Pts',(0.113781287599417,-0.769764858789943,
-0.8190754943662));
#56758=CARTESIAN_POINT('Ctrl Pts',(0.462913446150841,-0.625456042107333,
-0.808641531763721));
#56759=CARTESIAN_POINT('Ctrl Pts',(0.702932553865032,-0.333721356752229,
-0.798207569161239));
#56760=CARTESIAN_POINT('Ctrl Pts',(0.77726385077405,0.036674589509254,-0.787773606558759));
#56761=CARTESIAN_POINT('Ctrl Pts',(0.668386751451238,0.398425990267,-0.777339643956278));
#56762=CARTESIAN_POINT('Ctrl Pts',(0.401964611697131,0.666264639748313,
-0.766905681353797));
#56763=CARTESIAN_POINT('Ctrl Pts',(0.0407956343310049,0.777058450475451,
-0.756471718751316));
#56764=CARTESIAN_POINT('Ctrl Pts',(-0.329989257542916,0.704692279751986,
-0.746037756148837));
#56765=CARTESIAN_POINT('Ctrl Pts',(-0.622992579377318,0.466223514289631,
-0.735603793546355));
#56766=CARTESIAN_POINT('Ctrl Pts',(-0.769150693862395,0.11786148381372,
-0.725169830943876));
#56767=CARTESIAN_POINT('Ctrl Pts',(-0.734012759466783,-0.258281606344191,
-0.714735868341394));
#56768=CARTESIAN_POINT('Ctrl Pts',(-0.525861117638762,-0.573545293931952,
-0.704301905738914));
#56769=CARTESIAN_POINT('Ctrl Pts',(-0.19375906706945,-0.753618964174968,
-0.693867943136433));
#56770=CARTESIAN_POINT('Ctrl Pts',(0.184013817024176,-0.756057560229359,
-0.683433980533953));
#56771=CARTESIAN_POINT('Ctrl Pts',(0.518412914638575,-0.580286282081279,
-0.673000017931471));
#56772=CARTESIAN_POINT('Ctrl Pts',(0.73061721497504,-0.267736072313561,
-0.662566055328992));
#56773=CARTESIAN_POINT('Ctrl Pts',(0.770608169635336,0.107922046529214,
-0.65213209272651));
#56774=CARTESIAN_POINT('Ctrl Pts',(0.628959534674377,0.458141924492801,
-0.641698130124031));
#56775=CARTESIAN_POINT('Ctrl Pts',(0.339059224908709,0.700373444128261,
-0.631264167521549));
#56776=CARTESIAN_POINT('Ctrl Pts',(-0.0307605314660725,0.777520359180196,
-0.620830204919069));
#56777=CARTESIAN_POINT('Ctrl Pts',(-0.393329741412475,0.671398416557689,
-0.610396242316588));
#56778=CARTESIAN_POINT('Ctrl Pts',(-0.663187433844336,0.407021555727386,
-0.599962279714107));
#56779=CARTESIAN_POINT('Ctrl Pts',(-0.776725613880599,0.0467058880397525,
-0.589528317111628));
#56780=CARTESIAN_POINT('Ctrl Pts',(-0.707182265180475,-0.324618796513678,
-0.579094354509146));
#56781=CARTESIAN_POINT('Ctrl Pts',(-0.470949408769063,-0.619427779176754,
-0.568660391906666));
#56782=CARTESIAN_POINT('Ctrl Pts',(-0.123709349589915,-0.768231811408391,
-0.558226429304186));
#56783=CARTESIAN_POINT('Ctrl Pts',(0.25269016620706,-0.735956383991622,
-0.547792466701704));
#56784=CARTESIAN_POINT('Ctrl Pts',(0.569528234436074,-0.530209118571064,
-0.537358504099225));
#56785=CARTESIAN_POINT('Ctrl Pts',(0.752123144005562,-0.199486579716445,
-0.526924541496743));
#56786=CARTESIAN_POINT('Ctrl Pts',(0.757435558261681,0.178256821234392,
-0.516490578894263));
#56787=CARTESIAN_POINT('Ctrl Pts',(0.58421329122536,0.513983413731815,-0.506056616291782));
#56788=CARTESIAN_POINT('Ctrl Pts',(0.273286459598611,0.728559283954183,
-0.495622653689302));
#56789=CARTESIAN_POINT('Ctrl Pts',(-0.102056559562228,0.771406882187409,
-0.485188691086821));
#56790=CARTESIAN_POINT('Ctrl Pts',(-0.453343888260037,0.632426626742619,
-0.47475472848434));
#56791=CARTESIAN_POINT('Ctrl Pts',(-0.697773800873295,0.344377470300542,
-0.46432076588186));
#56792=CARTESIAN_POINT('Ctrl Pts',(-0.777731869256009,-0.0248446931832663,
-0.453886803279379));
#56793=CARTESIAN_POINT('Ctrl Pts',(-0.674371225051021,-0.388210728933227,
-0.443452840676899));
#56794=CARTESIAN_POINT('Ctrl Pts',(-0.412054943730932,-0.660071846531001,
-0.433018878074418));
#56795=CARTESIAN_POINT('Ctrl Pts',(-0.052613438684712,-0.776347824950466,
-0.422584915471938));
#56796=CARTESIAN_POINT('Ctrl Pts',(0.319229548446942,-0.709631323036312,
-0.412150952869457));
#56797=CARTESIAN_POINT('Ctrl Pts',(0.615827130120364,-0.475648047450975,
-0.401716990266977));
#56798=CARTESIAN_POINT('Ctrl Pts',(0.767268468189366,-0.129550055793595,
-0.391283027664495));
#56799=CARTESIAN_POINT('Ctrl Pts',(0.73785741566876,0.247084101843196,-0.380849065062015));
#56800=CARTESIAN_POINT('Ctrl Pts',(0.53452643409528,0.565478213973466,-0.370415102459534));
#56801=CARTESIAN_POINT('Ctrl Pts',(0.205202547258297,0.750583795355784,
-0.359981139857054));
#56802=CARTESIAN_POINT('Ctrl Pts',(-0.172489509004575,0.758769720339227,
-0.349547177254573));
#56803=CARTESIAN_POINT('Ctrl Pts',(-0.509524166428119,0.588106489551374,
-0.339113214652092));
#56804=CARTESIAN_POINT('Ctrl Pts',(-0.726459188269099,0.278821030603047,
-0.328679252049613));
#56805=CARTESIAN_POINT('Ctrl Pts',(-0.772160950053183,-0.0961851660426531,
-0.318245289447131));
#56806=CARTESIAN_POINT('Ctrl Pts',(-0.635857117988054,-0.448519615362855,
-0.307811326844651));
#56807=CARTESIAN_POINT('Ctrl Pts',(-0.349675784487414,-0.695133774103566,
-0.29737736424217));
#56808=CARTESIAN_POINT('Ctrl Pts',(0.0189274157531999,-0.777898369643473,
-0.28694340163969));
#56809=CARTESIAN_POINT('Ctrl Pts',(0.383069251609923,-0.677305003145055,
-0.276509439037209));
#56810=CARTESIAN_POINT('Ctrl Pts',(0.656918053157327,-0.417064487823471,
-0.266075476434728));
#56811=CARTESIAN_POINT('Ctrl Pts',(0.775925115315039,-0.0585179376441868,
-0.255641513832248));
#56812=CARTESIAN_POINT('Ctrl Pts',(0.712039292365906,0.313821812003498,
-0.245207551229767));
#56813=CARTESIAN_POINT('Ctrl Pts',(0.480319196218488,0.612190866640268,
-0.234773588627287));
#56814=CARTESIAN_POINT('Ctrl Pts',(0.135383189993233,0.766260668703223,
-0.224339626024806));
#56815=CARTESIAN_POINT('Ctrl Pts',(-0.24146359128836,0.739715845333337,
-0.213905663422326));
#56816=CARTESIAN_POINT('Ctrl Pts',(-0.561395755032477,0.538812615893194,
-0.203471700819845));
#56817=CARTESIAN_POINT('Ctrl Pts',(-0.749000440414917,0.210907029399764,
-0.193037738217364));
#56818=CARTESIAN_POINT('Ctrl Pts',(-0.760061084770159,-0.166712982541238,
-0.182603775614884));
#56819=CARTESIAN_POINT('Ctrl Pts',(-0.591963456523637,-0.50503391867701,
-0.172169813012403));
#56820=CARTESIAN_POINT('Ctrl Pts',(-0.284343786563672,-0.724320025643111,
-0.161735850409922));
#56821=CARTESIAN_POINT('Ctrl Pts',(0.0903167314019248,-0.772864465068914,
-0.151301887807442));
#56822=CARTESIAN_POINT('Ctrl Pts',(0.443652359236502,-0.639262442637615,
-0.140867925204961));
#56823=CARTESIAN_POINT('Ctrl Pts',(0.692489824641793,-0.354929918130671,
-0.130433962602481));
#56824=CARTESIAN_POINT('Ctrl Pts',(0.749438361810143,-0.109676867461668,
-0.12347798753416));
#56825=CARTESIAN_POINT('Ctrl Pts',(0.747395528060274,0.0124969850565577,
-0.12));
#56826=CARTESIAN_POINT('Ctrl Pts',(-0.453782243834438,0.594001620520165,
-1.13966850381659));
#56827=CARTESIAN_POINT('Ctrl Pts',(-0.550881059946449,0.519823845364617,
-1.13619051628243));
#56828=CARTESIAN_POINT('Ctrl Pts',(-0.707932492103508,0.323031139564102,
-1.12923454121411));
#56829=CARTESIAN_POINT('Ctrl Pts',(-0.776614348027597,-0.0485164852858499,
-1.11880057861163));
#56830=CARTESIAN_POINT('Ctrl Pts',(-0.662248261705562,-0.408538719445684,
-1.10836661600915));
#56831=CARTESIAN_POINT('Ctrl Pts',(-0.391780845205789,-0.672308389976757,
-1.09793265340667));
#56832=CARTESIAN_POINT('Ctrl Pts',(-0.0289685722792091,-0.777586516102956,
-1.08749869080419));
#56833=CARTESIAN_POINT('Ctrl Pts',(0.340672659850847,-0.699591427563091,
-1.07706472820171));
#56834=CARTESIAN_POINT('Ctrl Pts',(0.630013740257184,-0.456690353715166,
-1.06663076559923));
#56835=CARTESIAN_POINT('Ctrl Pts',(0.770854864632094,-0.106145971815379,
-1.05619680299675));
#56836=CARTESIAN_POINT('Ctrl Pts',(0.729998146909112,0.26941948793622,-1.04576284039427));
#56837=CARTESIAN_POINT('Ctrl Pts',(0.517074056599656,0.581479492398161,
-1.03532887779179));
#56838=CARTESIAN_POINT('Ctrl Pts',(0.182270723540416,0.756479695159438,
-1.02489491518931));
#56839=CARTESIAN_POINT('Ctrl Pts',(-0.195495518808872,0.753170329021128,
-1.01446095258683));
#56840=CARTESIAN_POINT('Ctrl Pts',(-0.527181636582193,0.572331734566928,
-1.00402698998435));
#56841=CARTESIAN_POINT('Ctrl Pts',(-0.73460608335552,0.25658912013712,-0.993593027381866));
#56842=CARTESIAN_POINT('Ctrl Pts',(-0.768876972472472,-0.119633936553384,
-0.983159064779384));
#56843=CARTESIAN_POINT('Ctrl Pts',(-0.621916330501673,-0.467658162697795,
-0.972725102176904));
#56844=CARTESIAN_POINT('Ctrl Pts',(-0.328364163622084,-0.705450957152497,
-0.962291139574423));
#56845=CARTESIAN_POINT('Ctrl Pts',(0.0425865236188016,-0.776962332806938,
-0.951857176971944));
#56846=CARTESIAN_POINT('Ctrl Pts',(0.403499166791982,-0.665336381154549,
-0.941423214369461));
#56847=CARTESIAN_POINT('Ctrl Pts',(0.669303263352646,-0.396884390885562,
-0.930989251766982));
#56848=CARTESIAN_POINT('Ctrl Pts',(0.777346288980351,-0.0348830183684705,
-0.920555289164501));
#56849=CARTESIAN_POINT('Ctrl Pts',(0.702161486931755,0.335340609270619,
-0.910121326562021));
#56850=CARTESIAN_POINT('Ctrl Pts',(0.461470621794524,0.626521303076041,
-0.899687363959539));
#56851=CARTESIAN_POINT('Ctrl Pts',(0.112006793088061,0.770025036127443,
-0.889253401357059));
#56852=CARTESIAN_POINT('Ctrl Pts',(-0.26385808966189,0.73202662963629,-0.878819438754579));
#56853=CARTESIAN_POINT('Ctrl Pts',(-0.577529140301392,0.52148266516939,
-0.868385476152097));
#56854=CARTESIAN_POINT('Ctrl Pts',(-0.755071143557591,0.188020334375048,
-0.857951513549617));
#56855=CARTESIAN_POINT('Ctrl Pts',(-0.754635780293312,-0.189760156704889,
-0.847517550947137));
#56856=CARTESIAN_POINT('Ctrl Pts',(-0.576325669722955,-0.522812395022917,
-0.837083588344655));
#56857=CARTESIAN_POINT('Ctrl Pts',(-0.262170181097151,-0.732632837180461,
-0.826649625742176));
#56858=CARTESIAN_POINT('Ctrl Pts',(0.113781283722264,-0.769764832559824,
-0.816215663139694));
#56859=CARTESIAN_POINT('Ctrl Pts',(0.462913430376835,-0.62545602079461,
-0.805781700537214));
#56860=CARTESIAN_POINT('Ctrl Pts',(0.702932529912258,-0.333721345380508,
-0.795347737934733));
#56861=CARTESIAN_POINT('Ctrl Pts',(0.7772638242884,0.0366745882595488,-0.784913775332253));
#56862=CARTESIAN_POINT('Ctrl Pts',(0.668386728675628,0.398425976690438,
-0.774479812729773));
#56863=CARTESIAN_POINT('Ctrl Pts',(0.401964597999988,0.666264617045015,
-0.764045850127292));
#56864=CARTESIAN_POINT('Ctrl Pts',(0.0407956329408735,0.7770584239968,-0.753611887524811));
#56865=CARTESIAN_POINT('Ctrl Pts',(-0.329989246298369,0.704692255739247,
-0.743177924922331));
#56866=CARTESIAN_POINT('Ctrl Pts',(-0.622992558148537,0.466223498402834,
-0.73274396231985));
#56867=CARTESIAN_POINT('Ctrl Pts',(-0.769150667653205,0.117861479797531,
-0.722309999717369));
#56868=CARTESIAN_POINT('Ctrl Pts',(-0.734012734454935,-0.258281597543118,
-0.711876037114889));
#56869=CARTESIAN_POINT('Ctrl Pts',(-0.525861099719784,-0.573545274388111,
-0.701442074512408));
#56870=CARTESIAN_POINT('Ctrl Pts',(-0.193759060467014,-0.75361893849503,
-0.691008111909928));
#56871=CARTESIAN_POINT('Ctrl Pts',(0.184013810753815,-0.756057534466323,
-0.680574149307446));
#56872=CARTESIAN_POINT('Ctrl Pts',(0.518412896973398,-0.580286262307737,
-0.670140186704967));
#56873=CARTESIAN_POINT('Ctrl Pts',(0.730617190078898,-0.267736063190322,
-0.659706224102485));
#56874=CARTESIAN_POINT('Ctrl Pts',(0.770608143376481,0.107922042851716,
-0.649272261500006));
#56875=CARTESIAN_POINT('Ctrl Pts',(0.62895951324227,0.458141908881389,-0.638838298897524));
#56876=CARTESIAN_POINT('Ctrl Pts',(0.339059213355098,0.700373420262689,
-0.628404336295044));
#56877=CARTESIAN_POINT('Ctrl Pts',(-0.0307605304178917,0.777520332685806,
-0.617970373692564));
#56878=CARTESIAN_POINT('Ctrl Pts',(-0.39332972800957,0.671398393679455,
-0.607536411090082));
#56879=CARTESIAN_POINT('Ctrl Pts',(-0.663187411245896,0.407021541857926,
-0.597102448487602));
#56880=CARTESIAN_POINT('Ctrl Pts',(-0.77672558741329,0.0467058864482261,
-0.586668485885121));
#56881=CARTESIAN_POINT('Ctrl Pts',(-0.70718224108289,-0.324618785452132,
-0.576234523282641));
#56882=CARTESIAN_POINT('Ctrl Pts',(-0.470949392721229,-0.619427758069446,
-0.56580056068016));
#56883=CARTESIAN_POINT('Ctrl Pts',(-0.123709345374458,-0.768231785230511,
-0.55536659807768));
#56884=CARTESIAN_POINT('Ctrl Pts',(0.252690157596518,-0.735956358913544,
-0.544932635475199));
#56885=CARTESIAN_POINT('Ctrl Pts',(0.569528215029118,-0.530209100503925,
-0.534498672872719));
#56886=CARTESIAN_POINT('Ctrl Pts',(0.752123118376594,-0.199486572918841,
-0.524064710270237));
#56887=CARTESIAN_POINT('Ctrl Pts',(0.757435532451691,0.178256815160203,
-0.513630747667758));
#56888=CARTESIAN_POINT('Ctrl Pts',(0.584213271318003,0.513983396217576,
-0.503196785065276));
#56889=CARTESIAN_POINT('Ctrl Pts',(0.27328645028624,0.728559259128164,-0.492762822462796));
#56890=CARTESIAN_POINT('Ctrl Pts',(-0.1020565560846,0.771406855901339,-0.482328859860315));
#56891=CARTESIAN_POINT('Ctrl Pts',(-0.45334387281212,0.632426605192368,
-0.471894897257835));
#56892=CARTESIAN_POINT('Ctrl Pts',(-0.697773777096307,0.344377458565709,
-0.461460934655354));
#56893=CARTESIAN_POINT('Ctrl Pts',(-0.777731842754411,-0.0248446923366709,
-0.451026972052874));
#56894=CARTESIAN_POINT('Ctrl Pts',(-0.674371202071488,-0.388210715704755,
-0.440593009450393));
#56895=CARTESIAN_POINT('Ctrl Pts',(-0.412054929689956,-0.660071824038725,
-0.430159046847913));
#56896=CARTESIAN_POINT('Ctrl Pts',(-0.0526134368918829,-0.776347798496032,
-0.419725084245432));
#56897=CARTESIAN_POINT('Ctrl Pts',(0.319229537569037,-0.70963129885527,
-0.409291121642951));
#56898=CARTESIAN_POINT('Ctrl Pts',(0.61582710913575,-0.475648031243039,
-0.398857159040471));
#56899=CARTESIAN_POINT('Ctrl Pts',(0.767268442044313,-0.129550051379102,
-0.38842319643799));
#56900=CARTESIAN_POINT('Ctrl Pts',(0.737857390525903,0.247084093423662,
-0.37798923383551));
#56901=CARTESIAN_POINT('Ctrl Pts',(0.534526415881029,0.565478194704557,
-0.367555271233028));
#56902=CARTESIAN_POINT('Ctrl Pts',(0.205202540265916,0.750583769779189,
-0.357121308630549));
#56903=CARTESIAN_POINT('Ctrl Pts',(-0.172489503126903,0.758769694483931,
-0.346687346028067));
#56904=CARTESIAN_POINT('Ctrl Pts',(-0.509524149065844,0.588106469511045,
-0.336253383425587));
#56905=CARTESIAN_POINT('Ctrl Pts',(-0.726459163514617,0.278821021102691,
-0.325819420823107));
#56906=CARTESIAN_POINT('Ctrl Pts',(-0.772160923741468,-0.0961851627662938,
-0.315385458220626));
#56907=CARTESIAN_POINT('Ctrl Pts',(-0.635857096320805,-0.44851960007697,
-0.304951495618145));
#56908=CARTESIAN_POINT('Ctrl Pts',(-0.349675772572242,-0.695133750421177,
-0.294517533015665));
#56909=CARTESIAN_POINT('Ctrl Pts',(0.018927415108638,-0.777898343127076,
-0.284083570413184));
#56910=CARTESIAN_POINT('Ctrl Pts',(0.383069238555864,-0.677304980083509,
-0.273649607810704));
#56911=CARTESIAN_POINT('Ctrl Pts',(0.656918030774064,-0.417064473576457,
-0.263215645208223));
#56912=CARTESIAN_POINT('Ctrl Pts',(0.775925088871969,-0.0585179357196898,
-0.252781682605742));
#56913=CARTESIAN_POINT('Ctrl Pts',(0.712039268108792,0.313821801446683,
-0.242347720003261));
#56914=CARTESIAN_POINT('Ctrl Pts',(0.480319179839611,0.612190845510341,
-0.231913757400781));
#56915=CARTESIAN_POINT('Ctrl Pts',(0.135383185403131,0.766260643122266,
-0.2214797947983));
#56916=CARTESIAN_POINT('Ctrl Pts',(-0.241463583105916,0.739715819084738,
-0.21104583219582));
#56917=CARTESIAN_POINT('Ctrl Pts',(-0.561395735813014,0.538812599584084,
-0.200611869593339));
#56918=CARTESIAN_POINT('Ctrl Pts',(-0.749000415068715,0.210907018176785,
-0.190177906990858));
#56919=CARTESIAN_POINT('Ctrl Pts',(-0.760061058523673,-0.166712968918104,
-0.179743944388378));
#56920=CARTESIAN_POINT('Ctrl Pts',(-0.591963437035102,-0.505033917097275,
-0.169309981785897));
#56921=CARTESIAN_POINT('Ctrl Pts',(-0.284343775530124,-0.724319970193128,
-0.158876019183417));
#56922=CARTESIAN_POINT('Ctrl Pts',(0.0903167256721143,-0.772864499431969,
-0.148442056580936));
#56923=CARTESIAN_POINT('Ctrl Pts',(0.443652349415133,-0.639262299658953,
-0.138008093978456));
#56924=CARTESIAN_POINT('Ctrl Pts',(0.692489789754636,-0.354930164383848,
-0.127574131375975));
#56925=CARTESIAN_POINT('Ctrl Pts',(0.749438354901216,-0.109676454265903,
-0.120618156307655));
#56926=CARTESIAN_POINT('Ctrl Pts',(0.747395528060274,0.0124969850565577,
-0.117140168773494));
#56927=CARTESIAN_POINT('Ctrl Pts',(-0.454743647135459,0.595260098846585,
-1.13299148312149));
#56928=CARTESIAN_POINT('Ctrl Pts',(-0.552049078435983,0.520924481859273,
-1.12951349558733));
#56929=CARTESIAN_POINT('Ctrl Pts',(-0.709431880792852,0.323716019874448,
-1.12255752051901));
#56930=CARTESIAN_POINT('Ctrl Pts',(-0.778260040912913,-0.0486194957500408,
-1.11212355791653));
#56931=CARTESIAN_POINT('Ctrl Pts',(-0.663651266471098,-0.409404197277853,
-1.10168959531405));
#56932=CARTESIAN_POINT('Ctrl Pts',(-0.392610989723493,-0.673732890143875,
-1.09125563271157));
#56933=CARTESIAN_POINT('Ctrl Pts',(-0.0290299167445373,-0.779233990024142,
-1.08082167010908));
#56934=CARTESIAN_POINT('Ctrl Pts',(0.341394439427491,-0.701073692506759,
-1.07038770750661));
#56935=CARTESIAN_POINT('Ctrl Pts',(0.631348582478224,-0.457657953570592,
-1.05995374490413));
#56936=CARTESIAN_POINT('Ctrl Pts',(0.772488099658164,-0.106370870957127,
-1.04951978230164));
#56937=CARTESIAN_POINT('Ctrl Pts',(0.731544823668044,0.2699903190294,-1.03908581969916));
#56938=CARTESIAN_POINT('Ctrl Pts',(0.518169599805944,0.582711493978721,
-1.02865185709668));
#56939=CARTESIAN_POINT('Ctrl Pts',(0.182656907952852,0.758082477697758,
-1.0182178944942));
#56940=CARTESIAN_POINT('Ctrl Pts',(-0.195909722819775,0.754766099154425,
-1.00778393189172));
#56941=CARTESIAN_POINT('Ctrl Pts',(-0.528298596051654,0.573544355519819,
-0.997349969289241));
#56942=CARTESIAN_POINT('Ctrl Pts',(-0.736162521039284,0.25713276511868,
-0.98691600668676));
#56943=CARTESIAN_POINT('Ctrl Pts',(-0.77050602107108,-0.119887409454014,
-0.97648204408428));
#56944=CARTESIAN_POINT('Ctrl Pts',(-0.623234008102326,-0.468649007698716,
-0.966048081481799));
#56945=CARTESIAN_POINT('Ctrl Pts',(-0.329059881148497,-0.706945622689529,
-0.955614118879318));
#56946=CARTESIAN_POINT('Ctrl Pts',(0.0426767532874446,-0.778608512204756,
-0.945180156276838));
#56947=CARTESIAN_POINT('Ctrl Pts',(0.404354075695012,-0.666746054432856,
-0.934746193674357));
#56948=CARTESIAN_POINT('Ctrl Pts',(0.670721341414737,-0.397725284812046,
-0.924312231071876));
#56949=CARTESIAN_POINT('Ctrl Pts',(0.778993281877019,-0.0349569263343661,
-0.913878268469396));
#56950=CARTESIAN_POINT('Ctrl Pts',(0.703649182952155,0.336051108064824,
-0.903444305866915));
#56951=CARTESIAN_POINT('Ctrl Pts',(0.462448357003046,0.627848737386998,
-0.893010343264436));
#56952=CARTESIAN_POINT('Ctrl Pts',(0.112244106104245,0.771656517208897,
-0.882576380661953));
#56953=CARTESIAN_POINT('Ctrl Pts',(-0.264417135746447,0.733577602061107,
-0.872142418059474));
#56954=CARTESIAN_POINT('Ctrl Pts',(-0.578752773069474,0.522587550157068,
-0.861708455456993));
#56955=CARTESIAN_POINT('Ctrl Pts',(-0.756670941263008,0.188418700147705,
-0.851274492854512));
#56956=CARTESIAN_POINT('Ctrl Pts',(-0.756234655578183,-0.190162208704721,
-0.840840530252032));
#56957=CARTESIAN_POINT('Ctrl Pts',(-0.577546752652513,-0.523920097359396,
-0.830406567649551));
#56958=CARTESIAN_POINT('Ctrl Pts',(-0.262725650946226,-0.734185094000027,
-0.819972605047071));
#56959=CARTESIAN_POINT('Ctrl Pts',(0.114022356418755,-0.771395762338238,
-0.80953864244459));
#56960=CARTESIAN_POINT('Ctrl Pts',(0.463894222518143,-0.626781198051683,
-0.79910467984211));
#56961=CARTESIAN_POINT('Ctrl Pts',(0.704421859570821,-0.334428413379528,
-0.788670717239629));
#56962=CARTESIAN_POINT('Ctrl Pts',(0.778910642463375,0.0367522920926851,
-0.778236754637147));
#56963=CARTESIAN_POINT('Ctrl Pts',(0.669802864842397,0.399270136831812,
-0.767802792034668));
#56964=CARTESIAN_POINT('Ctrl Pts',(0.402816255551772,0.667676257013847,
-0.757368829432187));
#56965=CARTESIAN_POINT('Ctrl Pts',(0.0408820681867801,0.778704806982432,
-0.746934866829706));
#56966=CARTESIAN_POINT('Ctrl Pts',(-0.330688406958327,0.706185313795279,
-0.736500904227226));
#56967=CARTESIAN_POINT('Ctrl Pts',(-0.624312515974405,0.46721130371009,
-0.726066941624745));
#56968=CARTESIAN_POINT('Ctrl Pts',(-0.770780296177272,0.11811119735931,
-0.715632979022265));
#56969=CARTESIAN_POINT('Ctrl Pts',(-0.735567914914891,-0.258828828503577,
-0.705199016419784));
#56970=CARTESIAN_POINT('Ctrl Pts',(-0.526975261461872,-0.57476046638923,
-0.694765053817304));
#56971=CARTESIAN_POINT('Ctrl Pts',(-0.194169585095039,-0.755215659358831,
-0.684331091214823));
#56972=CARTESIAN_POINT('Ctrl Pts',(0.184403687753781,-0.757659422075368,
-0.673897128612342));
#56973=CARTESIAN_POINT('Ctrl Pts',(0.519511277927458,-0.581515736694161,
-0.663463166009861));
#56974=CARTESIAN_POINT('Ctrl Pts',(0.732165176270938,-0.268303325683674,
-0.653029203407381));
#56975=CARTESIAN_POINT('Ctrl Pts',(0.772240859909324,0.108150701353624,
-0.6425952408049));
#56976=CARTESIAN_POINT('Ctrl Pts',(0.630292113480908,0.459112591420171,
-0.632161278202419));
#56977=CARTESIAN_POINT('Ctrl Pts',(0.339777590896286,0.701857327839134,
-0.621727315599939));
#56978=CARTESIAN_POINT('Ctrl Pts',(-0.0308257039136614,0.779167694334796,
-0.611293352997458));
#56979=CARTESIAN_POINT('Ctrl Pts',(-0.394163090536686,0.672820910774436,
-0.600859390394977));
#56980=CARTESIAN_POINT('Ctrl Pts',(-0.664592531422761,0.407883913747357,
-0.590425427792498));
#56981=CARTESIAN_POINT('Ctrl Pts',(-0.778371265205501,0.0468048439711131,
-0.579991465190016));
#56982=CARTESIAN_POINT('Ctrl Pts',(-0.708680574764765,-0.325306567514176,
-0.569557502587537));
#56983=CARTESIAN_POINT('Ctrl Pts',(-0.471947210958991,-0.620740163018959,
-0.559123539985055));
#56984=CARTESIAN_POINT('Ctrl Pts',(-0.123971453029556,-0.769859466883739,
-0.548689577382575));
#56985=CARTESIAN_POINT('Ctrl Pts',(0.25322554176231,-0.737515657403934,
-0.538255614780094));
#56986=CARTESIAN_POINT('Ctrl Pts',(0.570734895935091,-0.531332474519237,
-0.527821652177614));
#56987=CARTESIAN_POINT('Ctrl Pts',(0.753716669989903,-0.199909232643481,
-0.517387689575133));
#56988=CARTESIAN_POINT('Ctrl Pts',(0.759040339677032,0.17863449459651,-0.506953726972652));
#56989=CARTESIAN_POINT('Ctrl Pts',(0.585451066006504,0.515072392221348,
-0.496519764370172));
#56990=CARTESIAN_POINT('Ctrl Pts',(0.273865472594036,0.730102885104296,
-0.486085801767691));
#56991=CARTESIAN_POINT('Ctrl Pts',(-0.102272787158508,0.773041264696528,
-0.475651839165211));
#56992=CARTESIAN_POINT('Ctrl Pts',(-0.45430438957095,0.633766551289465,
-0.46521787656273));
#56993=CARTESIAN_POINT('Ctrl Pts',(-0.699252176710743,0.345107104073574,
-0.45478391396025));
#56994=CARTESIAN_POINT('Ctrl Pts',(-0.77937965253776,-0.0248973317232137,
-0.444349951357768));
#56995=CARTESIAN_POINT('Ctrl Pts',(-0.675800017767713,-0.389033232387461,
-0.433915988755288));
#56996=CARTESIAN_POINT('Ctrl Pts',(-0.412927966007995,-0.661470343103489,
-0.423482026152807));
#56997=CARTESIAN_POINT('Ctrl Pts',(-0.0527249109646674,-0.777992675852613,
-0.413048063550327));
#56998=CARTESIAN_POINT('Ctrl Pts',(0.319905901228363,-0.711134821448211,
-0.402614100947846));
#56999=CARTESIAN_POINT('Ctrl Pts',(0.617131885254587,-0.476655804663405,
-0.392180138345366));
#57000=CARTESIAN_POINT('Ctrl Pts',(0.768894082626004,-0.129824533958293,
-0.381746175742885));
#57001=CARTESIAN_POINT('Ctrl Pts',(0.739420716803659,0.247607599809944,
-0.371312213140405));
#57002=CARTESIAN_POINT('Ctrl Pts',(0.535658937155231,0.566676294679631,
-0.360878250537924));
#57003=CARTESIAN_POINT('Ctrl Pts',(0.205637310626131,0.752174059916795,
-0.350444287935443));
#57004=CARTESIAN_POINT('Ctrl Pts',(-0.172854963141739,0.760377328448251,
-0.340010325332963));
#57005=CARTESIAN_POINT('Ctrl Pts',(-0.510603697094482,0.589352512866214,
-0.329576362730482));
#57006=CARTESIAN_POINT('Ctrl Pts',(-0.727998339939051,0.279411769712721,
-0.319142400128002));
#57007=CARTESIAN_POINT('Ctrl Pts',(-0.773796930208484,-0.0963889538944966,
-0.308708437525521));
#57008=CARTESIAN_POINT('Ctrl Pts',(-0.6372043107291,-0.449469895473673,
-0.29827447492304));
#57009=CARTESIAN_POINT('Ctrl Pts',(-0.350416643817236,-0.69660655649887,
-0.28784051232056));
#57010=CARTESIAN_POINT('Ctrl Pts',(0.0189675173356873,-0.779546505705978,
-0.277406549718079));
#57011=CARTESIAN_POINT('Ctrl Pts',(0.383880861799198,-0.678740011636774,
-0.266972587115598));
#57012=CARTESIAN_POINT('Ctrl Pts',(0.658309867773886,-0.417948123900588,
-0.256538624513118));
#57013=CARTESIAN_POINT('Ctrl Pts',(0.777569070626036,-0.0586419196868113,
-0.246104661910637));
#57014=CARTESIAN_POINT('Ctrl Pts',(0.71354789254065,0.314486707157718,-0.235670699308157));
#57015=CARTESIAN_POINT('Ctrl Pts',(0.481336850230815,0.613487918075936,
-0.225236736705676));
#57016=CARTESIAN_POINT('Ctrl Pts',(0.135670026800068,0.767884146994866,
-0.214802774103195));
#57017=CARTESIAN_POINT('Ctrl Pts',(-0.24197518098053,0.741283085733479,
-0.204368811500715));
#57018=CARTESIAN_POINT('Ctrl Pts',(-0.562585186373488,0.539954196552602,
-0.193934848898234));
#57019=CARTESIAN_POINT('Ctrl Pts',(-0.750587350010887,0.211353885858101,
-0.183500886295754));
#57020=CARTESIAN_POINT('Ctrl Pts',(-0.761671429498338,-0.167066211673786,
-0.173066923693273));
#57021=CARTESIAN_POINT('Ctrl Pts',(-0.59321765042596,-0.506103908795656,
-0.162632961090792));
#57022=CARTESIAN_POINT('Ctrl Pts',(-0.284946229083329,-0.725854698300198,
-0.152198998488312));
#57023=CARTESIAN_POINT('Ctrl Pts',(0.0905080903716103,-0.774501830736828,
-0.141765035885831));
#57024=CARTESIAN_POINT('Ctrl Pts',(0.444592317906142,-0.640617059956728,
-0.131331073283351));
#57025=CARTESIAN_POINT('Ctrl Pts',(0.693957024835477,-0.35568146239315,
-0.12089711068087));
#57026=CARTESIAN_POINT('Ctrl Pts',(0.751026167303855,-0.109909948718264,
-0.11394113561255));
#57027=CARTESIAN_POINT('Ctrl Pts',(0.748978993560761,0.012523461726479,
-0.110463148078389));
#57028=CARTESIAN_POINT('Ctrl Pts',(-0.457725546467597,0.599163409431307,
-1.12801069747057));
#57029=CARTESIAN_POINT('Ctrl Pts',(-0.555667179198615,0.524341772031445,
-1.12453270993641));
#57030=CARTESIAN_POINT('Ctrl Pts',(-0.714084824405274,0.325837708337138,
-1.11757673486809));
#57031=CARTESIAN_POINT('Ctrl Pts',(-0.783362670351873,-0.0489378503027498,
-1.10714277226561));
#57032=CARTESIAN_POINT('Ctrl Pts',(-0.668003172418794,-0.412088937642732,
-1.09670880966312));
#57033=CARTESIAN_POINT('Ctrl Pts',(-0.395185257636937,-0.67815052788145,
-1.08627484706065));
#57034=CARTESIAN_POINT('Ctrl Pts',(-0.0292203366733351,-0.784343583971593,
-1.07584088445816));
#57035=CARTESIAN_POINT('Ctrl Pts',(0.343633040095591,-0.705670692032951,
-1.06540692185568));
#57036=CARTESIAN_POINT('Ctrl Pts',(0.635488397768254,-0.460658889708482,
-1.0549729592532));
#57037=CARTESIAN_POINT('Ctrl Pts',(0.777553410767087,-0.107068350619836,
-1.04453899665072));
#57038=CARTESIAN_POINT('Ctrl Pts',(0.736341651251885,0.271760675877952,
-1.03410503404824));
#57039=CARTESIAN_POINT('Ctrl Pts',(0.521567305771502,0.586532409010019,
-1.02367107144576));
#57040=CARTESIAN_POINT('Ctrl Pts',(0.183854611276035,0.763053319515687,
-1.01323710884328));
#57041=CARTESIAN_POINT('Ctrl Pts',(-0.197194327096822,0.759715196564629,
-1.0028031462408));
#57042=CARTESIAN_POINT('Ctrl Pts',(-0.531762717152964,0.577305158239887,
-0.99236918363832));
#57043=CARTESIAN_POINT('Ctrl Pts',(-0.740989631772395,0.258818817356293,
-0.981935221035839));
#57044=CARTESIAN_POINT('Ctrl Pts',(-0.775558326712227,-0.12067352644806,
-0.971501258433358));
#57045=CARTESIAN_POINT('Ctrl Pts',(-0.627320632386313,-0.471721998562319,
-0.961067295830878));
#57046=CARTESIAN_POINT('Ctrl Pts',(-0.331217568484237,-0.711581154688746,
-0.950633333228397));
#57047=CARTESIAN_POINT('Ctrl Pts',(0.0429565901738399,-0.783713946820615,
-0.940199370625917));
#57048=CARTESIAN_POINT('Ctrl Pts',(0.407005476575287,-0.671117992759011,
-0.929765408023434));
#57049=CARTESIAN_POINT('Ctrl Pts',(0.675119346199268,-0.400333219873854,
-0.919331445420956));
#57050=CARTESIAN_POINT('Ctrl Pts',(0.784101239483766,-0.035186143328752,
-0.908897482818474));
#57051=CARTESIAN_POINT('Ctrl Pts',(0.70826309976199,0.338254637741563,-0.898463520215994));
#57052=CARTESIAN_POINT('Ctrl Pts',(0.465480689448246,0.631965621074233,
-0.888029557613513));
#57053=CARTESIAN_POINT('Ctrl Pts',(0.112980104923762,0.776716366721998,
-0.877595595011033));
#57054=CARTESIAN_POINT('Ctrl Pts',(-0.266150952393821,0.738387763304697,
-0.867161632408552));
#57055=CARTESIAN_POINT('Ctrl Pts',(-0.582547728300969,0.526014222908736,
-0.856727669806072));
#57056=CARTESIAN_POINT('Ctrl Pts',(-0.761632528456596,0.189654185427614,
-0.846293707203591));
#57057=CARTESIAN_POINT('Ctrl Pts',(-0.761193381991244,-0.191409126391062,
-0.83585974460111));
#57058=CARTESIAN_POINT('Ctrl Pts',(-0.581333799855445,-0.527355507791801,
-0.825425781998629));
#57059=CARTESIAN_POINT('Ctrl Pts',(-0.264448376313448,-0.738999238645272,
-0.81499181939615));
#57060=CARTESIAN_POINT('Ctrl Pts',(0.114770015450621,-0.776453902048481,
-0.804557856793668));
#57061=CARTESIAN_POINT('Ctrl Pts',(0.466936035686987,-0.630891081748588,
-0.794123894191188));
#57062=CARTESIAN_POINT('Ctrl Pts',(0.709040842918429,-0.33662130284112,
-0.783689931588706));
#57063=CARTESIAN_POINT('Ctrl Pts',(0.784018058194349,0.0369932815265828,
-0.773255968986227));
#57064=CARTESIAN_POINT('Ctrl Pts',(0.674194847057106,0.401888201686226,
-0.762822006383745));
#57065=CARTESIAN_POINT('Ctrl Pts',(0.405457572755745,0.672054294791692,
-0.752388043781266));
#57066=CARTESIAN_POINT('Ctrl Pts',(0.0411501370855586,0.783810873024088,
-0.741954081178784));
#57067=CARTESIAN_POINT('Ctrl Pts',(-0.332856772724146,0.710815860335577,
-0.731520118576304));
#57068=CARTESIAN_POINT('Ctrl Pts',(-0.628406212210275,0.470274867400415,
-0.721086155973823));
#57069=CARTESIAN_POINT('Ctrl Pts',(-0.775834400197946,0.118885667439073,
-0.710652193371343));
#57070=CARTESIAN_POINT('Ctrl Pts',(-0.74039112689201,-0.260526001912516,
-0.700218230768863));
#57071=CARTESIAN_POINT('Ctrl Pts',(-0.530430704992227,-0.578529243560247,
-0.689784268166381));
#57072=CARTESIAN_POINT('Ctrl Pts',(-0.195442779655913,-0.760167704084639,
-0.679350305563902));
#57073=CARTESIAN_POINT('Ctrl Pts',(0.185612846088945,-0.762627490862809,
-0.66891634296142));
#57074=CARTESIAN_POINT('Ctrl Pts',(0.52291777917247,-0.585328809028116,
-0.65848238035894));
#57075=CARTESIAN_POINT('Ctrl Pts',(0.736966076059816,-0.27006262457056,
-0.648048417756459));
#57076=CARTESIAN_POINT('Ctrl Pts',(0.777304541031368,0.10885985919959,-0.637614455153979));
#57077=CARTESIAN_POINT('Ctrl Pts',(0.634425018694938,0.462123050828315,
-0.627180492551498));
#57078=CARTESIAN_POINT('Ctrl Pts',(0.342005555592323,0.706459495227383,
-0.616746529949017));
#57079=CARTESIAN_POINT('Ctrl Pts',(-0.0310278319582717,0.784276795587445,
-0.606312567346537));
#57080=CARTESIAN_POINT('Ctrl Pts',(-0.396747667841739,0.677232682698555,
-0.595878604744056));
#57081=CARTESIAN_POINT('Ctrl Pts',(-0.668950348821354,0.410558460227934,
-0.585444642141576));
#57082=CARTESIAN_POINT('Ctrl Pts',(-0.783475144171483,0.0471117492608237,
-0.575010679539095));
#57083=CARTESIAN_POINT('Ctrl Pts',(-0.713327483047262,-0.327439643877154,
-0.564576716936614));
#57084=CARTESIAN_POINT('Ctrl Pts',(-0.475041828592944,-0.624810434884064,
-0.554142754334134));
#57085=CARTESIAN_POINT('Ctrl Pts',(-0.124784349547945,-0.774907532910113,
-0.543708791731654));
#57086=CARTESIAN_POINT('Ctrl Pts',(0.254885973710435,-0.742351640975235,
-0.533274829129173));
#57087=CARTESIAN_POINT('Ctrl Pts',(0.574477276930804,-0.534816488847445,
-0.522840866526692));
#57088=CARTESIAN_POINT('Ctrl Pts',(0.758658885652574,-0.201220062800251,
-0.512406903924211));
#57089=CARTESIAN_POINT('Ctrl Pts',(0.764017463316078,0.179805823601479,
-0.501972941321731));
#57090=CARTESIAN_POINT('Ctrl Pts',(0.589289942793166,0.518449787130605,
-0.49153897871925));
#57091=CARTESIAN_POINT('Ctrl Pts',(0.275661243182654,0.734890262188806,
-0.48110501611677));
#57092=CARTESIAN_POINT('Ctrl Pts',(-0.102943402776664,0.778110194174132,
-0.470671053514289));
#57093=CARTESIAN_POINT('Ctrl Pts',(-0.457283320990613,0.63792223883224,
-0.460237090911809));
#57094=CARTESIAN_POINT('Ctrl Pts',(-0.703837261793103,0.347370015062493,
-0.449803128309327));
#57095=CARTESIAN_POINT('Ctrl Pts',(-0.78449014362719,-0.0250605866805469,
-0.439369165706848));
#57096=CARTESIAN_POINT('Ctrl Pts',(-0.680231324073688,-0.391584172562941,
-0.428935203104366));
#57097=CARTESIAN_POINT('Ctrl Pts',(-0.415635586978069,-0.665807687917846,
-0.418501240501886));
#57098=CARTESIAN_POINT('Ctrl Pts',(-0.0530706348834263,-0.783094072360267,
-0.408067277899405));
#57099=CARTESIAN_POINT('Ctrl Pts',(0.322003564738517,-0.715797822537025,
-0.397633315296925));
#57100=CARTESIAN_POINT('Ctrl Pts',(0.621178497185405,-0.479781297142647,
-0.387199352694444));
#57101=CARTESIAN_POINT('Ctrl Pts',(0.773935818505537,-0.13067580986956,
-0.376765390091964));
#57102=CARTESIAN_POINT('Ctrl Pts',(0.744269192090712,0.249231194201064,
-0.366331427489483));
#57103=CARTESIAN_POINT('Ctrl Pts',(0.539171320646896,0.570392062913125,
-0.355897464887002));
#57104=CARTESIAN_POINT('Ctrl Pts',(0.206985700515669,0.757106160489393,
-0.345463502284522));
#57105=CARTESIAN_POINT('Ctrl Pts',(-0.173988395026948,0.765363218892889,
-0.335029539682041));
#57106=CARTESIAN_POINT('Ctrl Pts',(-0.513951790203912,0.593216971932297,
-0.324595577079561));
#57107=CARTESIAN_POINT('Ctrl Pts',(-0.732771917254223,0.28124390807743,
-0.31416161447708));
#57108=CARTESIAN_POINT('Ctrl Pts',(-0.778870814680851,-0.0970209884795471,
-0.3037276518746));
#57109=CARTESIAN_POINT('Ctrl Pts',(-0.641382540095327,-0.452417126489898,
-0.293293689272119));
#57110=CARTESIAN_POINT('Ctrl Pts',(-0.352714370131851,-0.701174293940722,
-0.282859726669638));
#57111=CARTESIAN_POINT('Ctrl Pts',(0.0190918897513369,-0.784658090821038,
-0.272425764067158));
#57112=CARTESIAN_POINT('Ctrl Pts',(0.386398017223737,-0.68319059595668,
-0.261991801464677));
#57113=CARTESIAN_POINT('Ctrl Pts',(0.662626488959991,-0.420688662481479,
-0.251557838862196));
#57114=CARTESIAN_POINT('Ctrl Pts',(0.782667689483343,-0.0590264425752508,
-0.241123876259716));
#57115=CARTESIAN_POINT('Ctrl Pts',(0.718226716476131,0.316548837101509,
-0.230689913657235));
#57116=CARTESIAN_POINT('Ctrl Pts',(0.484493036851988,0.617510634526491,
-0.220255951054755));
#57117=CARTESIAN_POINT('Ctrl Pts',(0.136559632479484,0.772919263601256,
-0.209821988452274));
#57118=CARTESIAN_POINT('Ctrl Pts',(-0.243561843146326,0.746143766900964,
-0.199388025849794));
#57119=CARTESIAN_POINT('Ctrl Pts',(-0.566274128183453,0.543494756230501,
-0.188954063247313));
#57120=CARTESIAN_POINT('Ctrl Pts',(-0.75550904732574,0.212739737177773,
-0.178520100644832));
#57121=CARTESIAN_POINT('Ctrl Pts',(-0.766665803559575,-0.168161640964736,
-0.168086138042352));
#57122=CARTESIAN_POINT('Ctrl Pts',(-0.597107457561111,-0.509422584813054,
-0.157652175439871));
#57123=CARTESIAN_POINT('Ctrl Pts',(-0.286814649975467,-0.730614045087357,
-0.14721821283739));
#57124=CARTESIAN_POINT('Ctrl Pts',(0.0911015483498812,-0.779580681377717,
-0.13678425023491));
#57125=CARTESIAN_POINT('Ctrl Pts',(0.447507596061856,-0.644816980204467,
-0.126350287632429));
#57126=CARTESIAN_POINT('Ctrl Pts',(0.698507324942254,-0.358015175128548,
-0.115916325029948));
#57127=CARTESIAN_POINT('Ctrl Pts',(0.755950846588164,-0.110628321320808,
-0.108960349961628));
#57128=CARTESIAN_POINT('Ctrl Pts',(0.753890288033488,0.0126055820648136,
-0.105482362427468));
#57129=CARTESIAN_POINT('Ctrl Pts',(-0.459778808448974,0.601851132366397,
-1.12625));
#57130=CARTESIAN_POINT('Ctrl Pts',(-0.558161082255848,0.52669287114394,
-1.12277201246584));
#57131=CARTESIAN_POINT('Ctrl Pts',(-0.717287384517956,0.32730005915496,
-1.11581603739752));
#57132=CARTESIAN_POINT('Ctrl Pts',(-0.786877139371749,-0.0491576947563774,
-1.10538207479504));
#57133=CARTESIAN_POINT('Ctrl Pts',(-0.670999603978847,-0.413937381459674,
-1.09494811219256));
#57134=CARTESIAN_POINT('Ctrl Pts',(-0.396958121390906,-0.681192740453029,
-1.08451414959008));
#57135=CARTESIAN_POINT('Ctrl Pts',(-0.0293513702614997,-0.787862050964758,
-1.0740801869876));
#57136=CARTESIAN_POINT('Ctrl Pts',(0.345174528791172,-0.708836299099991,
-1.06364622438512));
#57137=CARTESIAN_POINT('Ctrl Pts',(0.638339163802785,-0.46272536101763,
-1.05321226178264));
#57138=CARTESIAN_POINT('Ctrl Pts',(0.78104145176708,-0.107548656621837,
-1.04277829918016));
#57139=CARTESIAN_POINT('Ctrl Pts',(0.739644828584922,0.272979776873327,
-1.03234433657767));
#57140=CARTESIAN_POINT('Ctrl Pts',(0.523907016570379,0.589163548674698,
-1.02191037397519));
#57141=CARTESIAN_POINT('Ctrl Pts',(0.184679370276396,0.766476320999639,
-1.01147641137271));
#57142=CARTESIAN_POINT('Ctrl Pts',(-0.198078926680867,0.763123222427558,
-1.00104244877023));
#57143=CARTESIAN_POINT('Ctrl Pts',(-0.53414816518828,0.579894906686743,
-0.990608486167753));
#57144=CARTESIAN_POINT('Ctrl Pts',(-0.74431365659454,0.259979859348694,
-0.980174523565271));
#57145=CARTESIAN_POINT('Ctrl Pts',(-0.779037423985492,-0.121214858921556,
-0.969740560962791));
#57146=CARTESIAN_POINT('Ctrl Pts',(-0.63013474640097,-0.473838108603285,
-0.95930659836031));
#57147=CARTESIAN_POINT('Ctrl Pts',(-0.332703386000087,-0.714773255138959,
-0.94887263575783));
#57148=CARTESIAN_POINT('Ctrl Pts',(0.0431492902551101,-0.78722962966257,
-0.938438673155349));
#57149=CARTESIAN_POINT('Ctrl Pts',(0.40883127306227,-0.674128578464592,
-0.928004710552868));
#57150=CARTESIAN_POINT('Ctrl Pts',(0.678147881681891,-0.40212908510846,
-0.917570747950388));
#57151=CARTESIAN_POINT('Ctrl Pts',(0.787618659686819,-0.0353439857660817,
-0.907136785347908));
#57152=CARTESIAN_POINT('Ctrl Pts',(0.711440315674566,0.339772023043391,
-0.896702822745426));
#57153=CARTESIAN_POINT('Ctrl Pts',(0.467568801414541,0.634800572137749,
-0.886268860142948));
#57154=CARTESIAN_POINT('Ctrl Pts',(0.113486925323209,0.78020065893068,-0.875834897540464));
#57155=CARTESIAN_POINT('Ctrl Pts',(-0.267344885893191,0.741700116231731,
-0.865400934937986));
#57156=CARTESIAN_POINT('Ctrl Pts',(-0.58516099435014,0.528373883831429,
-0.854966972335504));
#57157=CARTESIAN_POINT('Ctrl Pts',(-0.765049155681855,0.190504960084841,
-0.844533009733024));
#57158=CARTESIAN_POINT('Ctrl Pts',(-0.764608039237945,-0.192267773583724,
-0.834099047130543));
#57159=CARTESIAN_POINT('Ctrl Pts',(-0.583941620311303,-0.52972118561936,
-0.823665084528063));
#57160=CARTESIAN_POINT('Ctrl Pts',(-0.265634672182434,-0.742314334605434,
-0.813231121925582));
#57161=CARTESIAN_POINT('Ctrl Pts',(0.11528486525651,-0.77993701686014,-0.802797159323101));
#57162=CARTESIAN_POINT('Ctrl Pts',(0.469030676228696,-0.633721212507912,
-0.792363196720621));
#57163=CARTESIAN_POINT('Ctrl Pts',(0.712221547729785,-0.338131361123721,
-0.781929234118141));
#57164=CARTESIAN_POINT('Ctrl Pts',(0.787535105251362,0.0371592306530882,
-0.77149527151566));
#57165=CARTESIAN_POINT('Ctrl Pts',(0.67721923530673,0.403691042452732,-0.761061308913179));
#57166=CARTESIAN_POINT('Ctrl Pts',(0.407276425457032,0.675069080682076,
-0.750627346310698));
#57167=CARTESIAN_POINT('Ctrl Pts',(0.0413347335588412,0.787326990663742,
-0.740193383708218));
#57168=CARTESIAN_POINT('Ctrl Pts',(-0.334349943602905,0.714004527743863,
-0.729759421105736));
#57169=CARTESIAN_POINT('Ctrl Pts',(-0.631225196028521,0.472384485694395,
-0.719325458503257));
#57170=CARTESIAN_POINT('Ctrl Pts',(-0.779314735970098,0.119418979755566,
-0.708891495900776));
#57171=CARTESIAN_POINT('Ctrl Pts',(-0.743712466759962,-0.261694702299868,
-0.698457533298295));
#57172=CARTESIAN_POINT('Ctrl Pts',(-0.532810177927122,-0.581124482983871,
-0.688023570695815));
#57173=CARTESIAN_POINT('Ctrl Pts',(-0.196319521518959,-0.763577760216057,
-0.677589608093334));
#57174=CARTESIAN_POINT('Ctrl Pts',(0.186445491596607,-0.766048581415893,
-0.667155645490853));
#57175=CARTESIAN_POINT('Ctrl Pts',(0.525263549677469,-0.587954550799829,
-0.656721682888373));
#57176=CARTESIAN_POINT('Ctrl Pts',(0.740272051402902,-0.271274105542238,
-0.646287720285892));
#57177=CARTESIAN_POINT('Ctrl Pts',(0.780791471746631,0.109348196481395,
-0.635853757683412));
#57178=CARTESIAN_POINT('Ctrl Pts',(0.637271002434184,0.464196100675709,
-0.625419795080931));
#57179=CARTESIAN_POINT('Ctrl Pts',(0.34353976723478,0.709628620303801,-0.614985832478451));
#57180=CARTESIAN_POINT('Ctrl Pts',(-0.0311670205189606,0.787795003321278,
-0.604551869875969));
#57181=CARTESIAN_POINT('Ctrl Pts',(-0.39852744855339,0.68027069845432,-0.594117907273489));
#57182=CARTESIAN_POINT('Ctrl Pts',(-0.671951210639548,0.41240019513338,
-0.583683944671008));
#57183=CARTESIAN_POINT('Ctrl Pts',(-0.78698975575632,0.0473230890856614,
-0.573249982068528));
#57184=CARTESIAN_POINT('Ctrl Pts',(-0.716527417409383,-0.328908513916321,
-0.562816019466047));
#57185=CARTESIAN_POINT('Ctrl Pts',(-0.477172831122476,-0.627613288311015,
-0.552382056863567));
#57186=CARTESIAN_POINT('Ctrl Pts',(-0.125344122916367,-0.778383710824121,
-0.541948094261087));
#57187=CARTESIAN_POINT('Ctrl Pts',(0.256029373348164,-0.745681775564449,
-0.531514131658606));
#57188=CARTESIAN_POINT('Ctrl Pts',(0.577054339531638,-0.537215636084532,
-0.521080169056125));
#57189=CARTESIAN_POINT('Ctrl Pts',(0.762062173336032,-0.202122721128445,
-0.510646206453644));
#57190=CARTESIAN_POINT('Ctrl Pts',(0.767444789182846,0.180612419235498,
-0.500212243851164));
#57191=CARTESIAN_POINT('Ctrl Pts',(0.591933453918155,0.520775514553564,
-0.489778281248683));
#57192=CARTESIAN_POINT('Ctrl Pts',(0.276897839143596,0.738186925584304,
-0.479344318646203));
#57193=CARTESIAN_POINT('Ctrl Pts',(-0.103405199272281,0.781600738989842,
-0.468910356043722));
#57194=CARTESIAN_POINT('Ctrl Pts',(-0.459334660167692,0.640783910842519,
-0.458476393441241));
#57195=CARTESIAN_POINT('Ctrl Pts',(-0.706994623724163,0.34892829127361,
-0.448042430838761));
#57196=CARTESIAN_POINT('Ctrl Pts',(-0.78800930842456,-0.0251730066200001,
-0.43760846823628));
#57197=CARTESIAN_POINT('Ctrl Pts',(-0.683282791513013,-0.393340790216438,
-0.4271745056338));
#57198=CARTESIAN_POINT('Ctrl Pts',(-0.417500097498832,-0.668794451991525,
-0.416740543031318));
#57199=CARTESIAN_POINT('Ctrl Pts',(-0.0533087058287059,-0.786606974485122,
-0.406306580428839));
#57200=CARTESIAN_POINT('Ctrl Pts',(0.323448048928484,-0.719008838659507,
-0.395872617826358));
#57201=CARTESIAN_POINT('Ctrl Pts',(0.623965058008301,-0.481933560577747,
-0.385438655223877));
#57202=CARTESIAN_POINT('Ctrl Pts',(0.777407637380551,-0.131262011893549,
-0.375004692621397));
#57203=CARTESIAN_POINT('Ctrl Pts',(0.747607928672496,0.250349226915978,
-0.364570730018916));
#57204=CARTESIAN_POINT('Ctrl Pts',(0.541590003337533,0.57295079954568,-0.354136767416435));
#57205=CARTESIAN_POINT('Ctrl Pts',(0.207914223068492,0.760502482762858,
-0.343702804813955));
#57206=CARTESIAN_POINT('Ctrl Pts',(-0.174768894106414,0.768796581719081,
-0.333268842211474));
#57207=CARTESIAN_POINT('Ctrl Pts',(-0.51625733994508,0.595878099420951,
-0.322834879608994));
#57208=CARTESIAN_POINT('Ctrl Pts',(-0.736059077911031,0.282505547458036,
-0.312400917006513));
#57209=CARTESIAN_POINT('Ctrl Pts',(-0.782364771583724,-0.0974562174576689,
-0.301966954404032));
#57210=CARTESIAN_POINT('Ctrl Pts',(-0.644259734761704,-0.454446636287435,
-0.291532991801552));
#57211=CARTESIAN_POINT('Ctrl Pts',(-0.354296620723973,-0.704319709976542,
-0.281099029199071));
#57212=CARTESIAN_POINT('Ctrl Pts',(0.0191775345559786,-0.788178009053098,
-0.270665066596591));
#57213=CARTESIAN_POINT('Ctrl Pts',(0.388131370170823,-0.686255338400107,
-0.26023110399411));
#57214=CARTESIAN_POINT('Ctrl Pts',(0.665598982404196,-0.422575840864808,
-0.24979714139163));
#57215=CARTESIAN_POINT('Ctrl Pts',(0.786178678898117,-0.0592912305593693,
-0.239363178789148));
#57216=CARTESIAN_POINT('Ctrl Pts',(0.721448628413698,0.317968851246876,
-0.228929216186668));
#57217=CARTESIAN_POINT('Ctrl Pts',(0.486666436849563,0.620280742650438,
-0.218495253584187));
#57218=CARTESIAN_POINT('Ctrl Pts',(0.137172228805453,0.776386520196726,
-0.208061290981707));
#57219=CARTESIAN_POINT('Ctrl Pts',(-0.244654443391746,0.749490916798133,
-0.197627328379226));
#57220=CARTESIAN_POINT('Ctrl Pts',(-0.568814392418841,0.545932825443547,
-0.187193365776746));
#57221=CARTESIAN_POINT('Ctrl Pts',(-0.758898204371725,0.213694087832833,
-0.176759403174265));
#57222=CARTESIAN_POINT('Ctrl Pts',(-0.770105011053623,-0.168916032981121,
-0.166325440571785));
#57223=CARTESIAN_POINT('Ctrl Pts',(-0.599786034786049,-0.511707755229732,
-0.155891477969304));
#57224=CARTESIAN_POINT('Ctrl Pts',(-0.288101284597228,-0.733891647041669,
-0.145457515366823));
#57225=CARTESIAN_POINT('Ctrl Pts',(0.0915102336223925,-0.783077583290337,
-0.135023552764343));
#57226=CARTESIAN_POINT('Ctrl Pts',(0.449515061170523,-0.647710059517752,
-0.124589590161862));
#57227=CARTESIAN_POINT('Ctrl Pts',(0.701640821699951,-0.359620185801168,
-0.114155627559381));
#57228=CARTESIAN_POINT('Ctrl Pts',(0.759341912736313,-0.111126206723813,
-0.107199652491061));
#57229=CARTESIAN_POINT('Ctrl Pts',(0.757272083693561,0.0126621280946486,
-0.103721664956901));
#57230=CARTESIAN_POINT('Ctrl Pts',(0.555007866453738,-0.515351924808612,
-0.12));
#57231=CARTESIAN_POINT('Ctrl Pts',(0.591072083605962,-0.472049785910241,
-0.12));
#57232=CARTESIAN_POINT('Ctrl Pts',(0.641266713589833,-0.405214104043363,
-0.12));
#57233=CARTESIAN_POINT('Ctrl Pts',(0.703252213124767,-0.263984626534931,
-0.12));
#57234=CARTESIAN_POINT('Ctrl Pts',(0.719761895146739,-0.212714660677385,
-0.12));
#57235=CARTESIAN_POINT('Ctrl Pts',(0.742808661707171,-0.103336683918306,
-0.12));
#57236=CARTESIAN_POINT('Ctrl Pts',(0.748364886323481,-0.0454765203713869,
-0.12));
#57237=CARTESIAN_POINT('Ctrl Pts',(0.747395528060274,0.0124969850565566,
-0.12));
#57238=CARTESIAN_POINT('',(-0.738674446606902,0.114170753859872,-1.12625));
#57239=CARTESIAN_POINT('Ctrl Pts',(-0.738728321778976,0.114178441930245,
-1.12625));
#57240=CARTESIAN_POINT('Ctrl Pts',(-0.729872306490505,0.171476380149593,
-1.12625));
#57241=CARTESIAN_POINT('Ctrl Pts',(-0.714604763127107,0.227558322531754,
-1.12625));
#57242=CARTESIAN_POINT('Ctrl Pts',(-0.673382241080463,0.331452140304371,
-1.12625));
#57243=CARTESIAN_POINT('Ctrl Pts',(-0.648435827358875,0.379185799077549,
-1.12625));
#57244=CARTESIAN_POINT('Ctrl Pts',(-0.563441537104104,0.507894222797762,
-1.12625));
#57245=CARTESIAN_POINT('Ctrl Pts',(-0.502653830377742,0.565275533421067,
-1.12625));
#57246=CARTESIAN_POINT('Ctrl Pts',(-0.459778808448976,0.601851132366395,
-1.12625));
#57247=CARTESIAN_POINT('Ctrl Pts',(-0.73867444479349,0.114170753601095,
-1.12625));
#57248=CARTESIAN_POINT('Ctrl Pts',(-0.744523251396961,0.0764015856923683,
-1.12516243468899));
#57249=CARTESIAN_POINT('Ctrl Pts',(-0.747504748693495,0.0381902463136735,
-1.12407486937799));
#57250=CARTESIAN_POINT('Ctrl Pts',(-0.747536615034749,-1.54000427278079E-5,
-1.12298730406698));
#57251=CARTESIAN_POINT('Origin',(-9.99409214431492E-17,0.,-1.12625));
#57252=CARTESIAN_POINT('',(-0.82685,-1.01259920587499E-16,-1.12625));
#57253=CARTESIAN_POINT('Origin',(0.,0.,-1.12625));
#57254=CARTESIAN_POINT('Origin',(0.,0.,-1.12625));
#57255=CARTESIAN_POINT('',(0.589301091561366,-0.565833523687262,-1.12625));
#57256=CARTESIAN_POINT('Ctrl Pts',(0.82685,-1.28508315100362E-14,-1.12625));
#57257=CARTESIAN_POINT('Ctrl Pts',(0.826849999999999,-0.0640849384885683,
-1.12625));
#57258=CARTESIAN_POINT('Ctrl Pts',(0.819177389464159,-0.127972397977417,
-1.12625));
#57259=CARTESIAN_POINT('Ctrl Pts',(0.789918090291951,-0.247778859616496,
-1.12625));
#57260=CARTESIAN_POINT('Ctrl Pts',(0.769494724754838,-0.303642805552855,
-1.12625));
#57261=CARTESIAN_POINT('Ctrl Pts',(0.695180543122699,-0.452454840062382,
-1.12625));
#57262=CARTESIAN_POINT('Ctrl Pts',(0.63618267061235,-0.521654825860835,
-1.12625));
#57263=CARTESIAN_POINT('Ctrl Pts',(0.589301091561366,-0.565833523687262,
-1.12625));
#57264=CARTESIAN_POINT('',(-0.459778808448989,-0.601851132366385,-1.12625));
#57265=CARTESIAN_POINT('Ctrl Pts',(0.589349009255739,-0.565869316348666,
-1.12625));
#57266=CARTESIAN_POINT('Ctrl Pts',(0.561797955794756,-0.591801457111598,
-1.12625));
#57267=CARTESIAN_POINT('Ctrl Pts',(0.53250376759911,-0.61571900169366,-1.12625));
#57268=CARTESIAN_POINT('Ctrl Pts',(0.501718244977289,-0.637497823098473,
-1.12625));
#57269=CARTESIAN_POINT('Ctrl Pts',(0.471023065979674,-0.659212732070133,
-1.12625));
#57270=CARTESIAN_POINT('Ctrl Pts',(0.438844183868204,-0.67880200460138,
-1.12625));
#57271=CARTESIAN_POINT('Ctrl Pts',(0.405405868387118,-0.696097894311475,
-1.12625));
#57272=CARTESIAN_POINT('Ctrl Pts',(0.39491538256918,-0.701524073325039,
-1.12625));
#57273=CARTESIAN_POINT('Ctrl Pts',(0.384300816323107,-0.706724162922387,
-1.12625));
#57274=CARTESIAN_POINT('Ctrl Pts',(0.373568843076448,-0.711691937718432,
-1.12625));
#57275=CARTESIAN_POINT('Ctrl Pts',(0.36393057823419,-0.716153440562365,
-1.12625));
#57276=CARTESIAN_POINT('Ctrl Pts',(0.354194037390873,-0.720428823534973,
-1.12625));
#57277=CARTESIAN_POINT('Ctrl Pts',(0.344389136281756,-0.724503440481216,
-1.12625));
#57278=CARTESIAN_POINT('Ctrl Pts',(0.31940466556717,-0.734886222177191,
-1.12625));
#57279=CARTESIAN_POINT('Ctrl Pts',(0.293946819979983,-0.743981294593248,
-1.12625));
#57280=CARTESIAN_POINT('Ctrl Pts',(0.268101859965993,-0.751732914379289,
-1.12625));
#57281=CARTESIAN_POINT('Ctrl Pts',(0.236780787659364,-0.76112697200912,
-1.12625));
#57282=CARTESIAN_POINT('Ctrl Pts',(0.204890853635392,-0.768548833828937,
-1.12625));
#57283=CARTESIAN_POINT('Ctrl Pts',(0.172622384826076,-0.773986220742675,
-1.12625));
#57284=CARTESIAN_POINT('Ctrl Pts',(0.153540924365838,-0.777201535482726,
-1.12625));
#57285=CARTESIAN_POINT('Ctrl Pts',(0.134327020168851,-0.779722340056188,
-1.12625));
#57286=CARTESIAN_POINT('Ctrl Pts',(0.115020357875884,-0.781541004368767,
-1.12625));
#57287=CARTESIAN_POINT('Ctrl Pts',(0.103888024742991,-0.782589656729145,
-1.12625));
#57288=CARTESIAN_POINT('Ctrl Pts',(0.092719076500179,-0.783404877147977,
-1.12625));
#57289=CARTESIAN_POINT('Ctrl Pts',(0.0815541189292635,-0.783983582560274,
-1.12625));
#57290=CARTESIAN_POINT('Ctrl Pts',(0.0448646731874593,-0.785885280859626,
-1.12625));
#57291=CARTESIAN_POINT('Ctrl Pts',(0.00816270548319765,-0.785244764668238,
-1.12625));
#57292=CARTESIAN_POINT('Ctrl Pts',(-0.0282824614477115,-0.782055278068263,
-1.12625));
#57293=CARTESIAN_POINT('Ctrl Pts',(-0.0590932645529008,-0.779358880934872,
-1.12625));
#57294=CARTESIAN_POINT('Ctrl Pts',(-0.0897210642543918,-0.774839835383059,
-1.12625));
#57295=CARTESIAN_POINT('Ctrl Pts',(-0.119998031533351,-0.768465408942047,
-1.12625));
#57296=CARTESIAN_POINT('Ctrl Pts',(-0.136473000057102,-0.764996816001246,
-1.12625));
#57297=CARTESIAN_POINT('Ctrl Pts',(-0.152843949864888,-0.760978380225147,
-1.12625));
#57298=CARTESIAN_POINT('Ctrl Pts',(-0.169085499191347,-0.756419224292614,
-1.12625));
#57299=CARTESIAN_POINT('Ctrl Pts',(-0.177940972571241,-0.753933409473855,
-1.12625));
#57300=CARTESIAN_POINT('Ctrl Pts',(-0.186757956437418,-0.75128681397849,
-1.12625));
#57301=CARTESIAN_POINT('Ctrl Pts',(-0.195532162352344,-0.748480681726736,
-1.12625));
#57302=CARTESIAN_POINT('Ctrl Pts',(-0.202583374982168,-0.746225590455074,
-1.12625));
#57303=CARTESIAN_POINT('Ctrl Pts',(-0.209606136429063,-0.743867596216528,
-1.12625));
#57304=CARTESIAN_POINT('Ctrl Pts',(-0.216586046830733,-0.741412001954268,
-1.12625));
#57305=CARTESIAN_POINT('Ctrl Pts',(-0.250777745036905,-0.729383059876171,
-1.12625));
#57306=CARTESIAN_POINT('Ctrl Pts',(-0.284021591240393,-0.714991447732211,
-1.12625));
#57307=CARTESIAN_POINT('Ctrl Pts',(-0.316082870424553,-0.698370323834583,
-1.12625));
#57308=CARTESIAN_POINT('Ctrl Pts',(-0.347689999411748,-0.681984639285725,
-1.12625));
#57309=CARTESIAN_POINT('Ctrl Pts',(-0.378148790578374,-0.663431461246423,
-1.12625));
#57310=CARTESIAN_POINT('Ctrl Pts',(-0.40720704752179,-0.64279703590621,
-1.12625));
#57311=CARTESIAN_POINT('Ctrl Pts',(-0.425297299274875,-0.629951050343084,
-1.12625));
#57312=CARTESIAN_POINT('Ctrl Pts',(-0.442844152591749,-0.616297659809349,
-1.12625));
#57313=CARTESIAN_POINT('Ctrl Pts',(-0.459778808448986,-0.601851132366388,
-1.12625));
#57314=CARTESIAN_POINT('Ctrl Pts',(-0.459778808448986,-0.601851132366387,
-1.12625));
#57315=CARTESIAN_POINT('Ctrl Pts',(-0.506938887193883,-0.5616200596157,
-1.12625));
#57316=CARTESIAN_POINT('Ctrl Pts',(-0.580457877279435,-0.492400554929899,
-1.12625));
#57317=CARTESIAN_POINT('Ctrl Pts',(-0.691141067841613,-0.302309651856746,
-1.12625));
#57318=CARTESIAN_POINT('Ctrl Pts',(-0.723888788631576,-0.210189415916568,
-1.12625));
#57319=CARTESIAN_POINT('Ctrl Pts',(-0.738728321778979,-0.114178441930225,
-1.12625));
#57320=CARTESIAN_POINT('Origin',(0.,0.,-1.12625));
#57321=CARTESIAN_POINT('Origin',(0.,0.,-1.33003901172249));
#57322=CARTESIAN_POINT('Ctrl Pts',(-0.748490343485036,-0.115687267834994,
-1.1425283350431));
#57323=CARTESIAN_POINT('Ctrl Pts',(-0.729579393836473,-0.238040085590791,
-1.13905034750894));
#57324=CARTESIAN_POINT('Ctrl Pts',(-0.630653629844322,-0.473183377928875,
-1.13209437244062));
#57325=CARTESIAN_POINT('Ctrl Pts',(-0.333406559150436,-0.714445366112156,
-1.12166040983814));
#57326=CARTESIAN_POINT('Ctrl Pts',(0.0423441932323904,-0.787268438306116,
-1.11122644723566));
#57327=CARTESIAN_POINT('Ctrl Pts',(0.40815462829301,-0.674543622261523,
-1.10079248463318));
#57328=CARTESIAN_POINT('Ctrl Pts',(0.677738701453825,-0.402813068451867,
-1.0903585220307));
#57329=CARTESIAN_POINT('Ctrl Pts',(0.787583785039378,-0.0361404951497466,
-1.07992455942822));
#57330=CARTESIAN_POINT('Ctrl Pts',(0.711782686348956,0.339053175380459,
-1.06949059682573));
#57331=CARTESIAN_POINT('Ctrl Pts',(0.468210400798602,0.634327583870298,
-1.05905663422325));
#57332=CARTESIAN_POINT('Ctrl Pts',(0.114275158775044,0.780085648735315,
-1.04862267162077));
#57333=CARTESIAN_POINT('Ctrl Pts',(-0.266595119432196,0.741969872482332,
-1.03818870901829));
#57334=CARTESIAN_POINT('Ctrl Pts',(-0.584626774041369,0.528964985372609,
-1.02775474641581));
#57335=CARTESIAN_POINT('Ctrl Pts',(-0.764856223313064,0.191277995929144,
-1.01732078381333));
#57336=CARTESIAN_POINT('Ctrl Pts',(-0.764801961726998,-0.191494973175325,
-1.00688682121085));
#57337=CARTESIAN_POINT('Ctrl Pts',(-0.584476642087926,-0.529130798350251,
-0.996452858608371));
#57338=CARTESIAN_POINT('Ctrl Pts',(-0.26638470707097,-0.742045509438615,
-0.98601889600589));
#57339=CARTESIAN_POINT('Ctrl Pts',(0.114496619465382,-0.780053123936527,
-0.975584933403409));
#57340=CARTESIAN_POINT('Ctrl Pts',(0.468390010412389,-0.634194881491945,
-0.965150970800929));
#57341=CARTESIAN_POINT('Ctrl Pts',(0.711879475926061,-0.338850945209242,
-0.954717008198449));
#57342=CARTESIAN_POINT('Ctrl Pts',(0.787572255433586,0.0363633449241294,
-0.944283045595967));
#57343=CARTESIAN_POINT('Ctrl Pts',(0.67762685162374,0.403006452460029,-0.933849082993488));
#57344=CARTESIAN_POINT('Ctrl Pts',(0.40795842850662,0.674657150909492,-0.923415120391005));
#57345=CARTESIAN_POINT('Ctrl Pts',(0.0421303690166799,0.78728481673588,
-0.912981157788527));
#57346=CARTESIAN_POINT('Ctrl Pts',(-0.333628214598002,0.714342050500303,
-0.902547195186044));
#57347=CARTESIAN_POINT('Ctrl Pts',(-0.630747491734475,0.473022147824028,
-0.892113232583565));
#57348=CARTESIAN_POINT('Ctrl Pts',(-0.779193655806612,0.120206478312629,
-0.881679269981084));
#57349=CARTESIAN_POINT('Ctrl Pts',(-0.743976550446063,-0.260942988134431,
-0.871245307378603));
#57350=CARTESIAN_POINT('Ctrl Pts',(-0.53339717846247,-0.58058573930206,
-0.860811344776123));
#57351=CARTESIAN_POINT('Ctrl Pts',(-0.197091077355778,-0.763378973969725,
-0.850377382173642));
#57352=CARTESIAN_POINT('Ctrl Pts',(0.1856712434202,-0.766236608391143,-0.839943419571162));
#57353=CARTESIAN_POINT('Ctrl Pts',(0.524669106735824,-0.588485071271487,
-0.829509456968681));
#57354=CARTESIAN_POINT('Ctrl Pts',(0.739997529484913,-0.272022070847804,
-0.8190754943662));
#57355=CARTESIAN_POINT('Ctrl Pts',(0.780901578249223,0.108559088795519,
-0.80864153176372));
#57356=CARTESIAN_POINT('Ctrl Pts',(0.63773978421953,0.463551850709081,-0.798207569161239));
#57357=CARTESIAN_POINT('Ctrl Pts',(0.34425672802939,0.709281083829745,-0.787773606558759));
#57358=CARTESIAN_POINT('Ctrl Pts',(-0.0303708751141361,0.787826097953732,
-0.777339643956278));
#57359=CARTESIAN_POINT('Ctrl Pts',(-0.397839777494351,0.680673094896104,
-0.766905681353797));
#57360=CARTESIAN_POINT('Ctrl Pts',(-0.671534104459314,0.413079044760477,
-0.756471718751318));
#57361=CARTESIAN_POINT('Ctrl Pts',(-0.786941530302541,0.0481183806594918,
-0.746037756148836));
#57362=CARTESIAN_POINT('Ctrl Pts',(-0.716859439874856,-0.328184238095781,
-0.735603793546357));
#57363=CARTESIAN_POINT('Ctrl Pts',(-0.477806840690935,-0.627130746863161,
-0.725169830943874));
#57364=CARTESIAN_POINT('Ctrl Pts',(-0.126130677572574,-0.778256643304304,
-0.714735868341395));
#57365=CARTESIAN_POINT('Ctrl Pts',(0.255275671930622,-0.745940132981574,
-0.704301905738913));
#57366=CARTESIAN_POINT('Ctrl Pts',(0.576511145861981,-0.537798521166715,
-0.693867943136434));
#57367=CARTESIAN_POINT('Ctrl Pts',(0.761857523268443,-0.202892742382452,
-0.683433980533952));
#57368=CARTESIAN_POINT('Ctrl Pts',(0.767626920662054,0.179836763057757,
-0.673000017931472));
#57369=CARTESIAN_POINT('Ctrl Pts',(0.592459436842396,0.520177052904672,
-0.662566055328991));
#57370=CARTESIAN_POINT('Ctrl Pts',(0.277643694393171,0.7379067215007,-0.652132092726511));
#57371=CARTESIAN_POINT('Ctrl Pts',(-0.102615276791054,0.781704839208057,
-0.64169813012403));
#57372=CARTESIAN_POINT('Ctrl Pts',(-0.458686862609225,0.641247777962548,
-0.63126416752155));
#57373=CARTESIAN_POINT('Ctrl Pts',(-0.706641643062582,0.349642587454695,
-0.620830204919068));
#57374=CARTESIAN_POINT('Ctrl Pts',(-0.788034345519909,-0.0243766477023798,
-0.610396242316589));
#57375=CARTESIAN_POINT('Ctrl Pts',(-0.683679944886671,-0.392650077845349,
-0.599962279714108));
#57376=CARTESIAN_POINT('Ctrl Pts',(-0.418175754367006,-0.668372193565669,
-0.589528317111627));
#57377=CARTESIAN_POINT('Ctrl Pts',(-0.0541036075165322,-0.786552700285172,
-0.579094354509147));
#57378=CARTESIAN_POINT('Ctrl Pts',(0.322721268222067,-0.719335341624016,
-0.568660391906666));
#57379=CARTESIAN_POINT('Ctrl Pts',(0.623477707326197,-0.482563880889843,
-0.558226429304186));
#57380=CARTESIAN_POINT('Ctrl Pts',(0.777274589863052,-0.132047577128183,
-0.547792466701705));
#57381=CARTESIAN_POINT('Ctrl Pts',(0.747860544863849,0.249593581864889,
-0.537358504099224));
#57382=CARTESIAN_POINT('Ctrl Pts',(0.542168739239193,0.572403187328638,
-0.526924541496743));
#57383=CARTESIAN_POINT('Ctrl Pts',(0.208682665163577,0.760291980710321,
-0.516490578894263));
#57384=CARTESIAN_POINT('Ctrl Pts',(-0.173991874795186,0.768972807176858,
-0.506056616291782));
#57385=CARTESIAN_POINT('Ctrl Pts',(-0.515654894268529,0.596399514326687,
-0.495622653689302));
#57386=CARTESIAN_POINT('Ctrl Pts',(-0.735773207791702,0.283249249545539,
-0.485188691086821));
#57387=CARTESIAN_POINT('Ctrl Pts',(-0.782462859663332,-0.0966655260145957,
-0.47475472848434));
#57388=CARTESIAN_POINT('Ctrl Pts',(-0.644718660035084,-0.453795328396793,
-0.46432076588186));
#57389=CARTESIAN_POINT('Ctrl Pts',(-0.355008211612248,-0.703961306010574,
-0.453886803279379));
#57390=CARTESIAN_POINT('Ctrl Pts',(0.018381009512838,-0.788196986267641,
-0.443452840676898));
#57391=CARTESIAN_POINT('Ctrl Pts',(0.387437653906621,-0.686647227481264,
-0.433018878074418));
#57392=CARTESIAN_POINT('Ctrl Pts',(0.665171601199015,-0.423248262406717,
-0.422584915471937));
#57393=CARTESIAN_POINT('Ctrl Pts',(0.786118349198422,-0.0600857031737081,
-0.412150952869458));
#57394=CARTESIAN_POINT('Ctrl Pts',(0.721769612451193,0.317239621129983,
-0.401716990266976));
#57395=CARTESIAN_POINT('Ctrl Pts',(0.487292993114226,0.619788584544707,
-0.391283027664496));
#57396=CARTESIAN_POINT('Ctrl Pts',(0.137956834542056,0.776247552318673,
-0.380849065062015));
#57397=CARTESIAN_POINT('Ctrl Pts',(-0.243897046781887,0.749737674945353,
-0.370415102459534));
#57398=CARTESIAN_POINT('Ctrl Pts',(-0.56826210144847,0.546507579770122,
-0.359981139857054));
#57399=CARTESIAN_POINT('Ctrl Pts',(-0.758682436896786,0.214460510585709,
-0.349547177254573));
#57400=CARTESIAN_POINT('Ctrl Pts',(-0.770274190049176,-0.168136916847529,
-0.339113214652093));
#57401=CARTESIAN_POINT('Ctrl Pts',(-0.600305075684723,-0.511102892647924,
-0.328679252049612));
#57402=CARTESIAN_POINT('Ctrl Pts',(-0.288838411909716,-0.733597111627555,
-0.318245289447132));
#57403=CARTESIAN_POINT('Ctrl Pts',(0.0907101808453047,-0.783175596150041,
-0.307811326844651));
#57404=CARTESIAN_POINT('Ctrl Pts',(0.448877531081795,-0.648152228766215,
-0.29737736424217));
#57405=CARTESIAN_POINT('Ctrl Pts',(0.701240227960024,-0.360353291538606,
-0.28694340163969));
#57406=CARTESIAN_POINT('Ctrl Pts',(0.788314010461381,0.0123843106225132,
-0.276509439037209));
#57407=CARTESIAN_POINT('Ctrl Pts',(0.689574771586226,0.382202801273034,
-0.266075476434728));
#57408=CARTESIAN_POINT('Ctrl Pts',(0.428296274062381,0.661932524534914,
-0.255641513832248));
#57409=CARTESIAN_POINT('Ctrl Pts',(0.0660643238823166,0.785638478676652,
-0.245207551229767));
#57410=CARTESIAN_POINT('Ctrl Pts',(-0.311739618905992,0.72416215772478,
-0.234773588627286));
#57411=CARTESIAN_POINT('Ctrl Pts',(-0.616063582497875,0.491993812660686,
-0.224339626024806));
#57412=CARTESIAN_POINT('Ctrl Pts',(-0.775175608854643,0.14385828691005,
-0.213905663422325));
#57413=CARTESIAN_POINT('Ctrl Pts',(-0.751571377703367,-0.238186748774525,
-0.203471700819845));
#57414=CARTESIAN_POINT('Ctrl Pts',(-0.550814864235516,-0.5640874344097,
-0.193037738217364));
#57415=CARTESIAN_POINT('Ctrl Pts',(-0.220225801435357,-0.757030349608771,
-0.182603775614884));
#57416=CARTESIAN_POINT('Ctrl Pts',(0.162271947040142,-0.771528308468151,
-0.172169813012403));
#57417=CARTESIAN_POINT('Ctrl Pts',(0.506521864189483,-0.604181181458603,
-0.161735850409922));
#57418=CARTESIAN_POINT('Ctrl Pts',(0.73137747471038,-0.294400431622848,
-0.151301887807442));
#57419=CARTESIAN_POINT('Ctrl Pts',(0.78384510265579,0.0847288019872882,
-0.140867925204961));
#57420=CARTESIAN_POINT('Ctrl Pts',(0.651544586453749,0.443977659175339,
-0.13043396260248));
#57421=CARTESIAN_POINT('Ctrl Pts',(0.460967102820788,0.613562143858204,
-0.12347798753416));
#57422=CARTESIAN_POINT('Ctrl Pts',(0.351283760559796,0.670985139773185,
-0.12));
#57423=CARTESIAN_POINT('Ctrl Pts',(-0.745983409600528,-0.115299794123053,
-1.14120781194017));
#57424=CARTESIAN_POINT('Ctrl Pts',(-0.727135791628743,-0.237242859367687,
-1.13772982440601));
#57425=CARTESIAN_POINT('Ctrl Pts',(-0.628541377473358,-0.471598508427924,
-1.13077384933769));
#57426=CARTESIAN_POINT('Ctrl Pts',(-0.332289872157592,-0.71205247591253,
-1.12033988673521));
#57427=CARTESIAN_POINT('Ctrl Pts',(0.0422023676688991,-0.78463162043964,
-1.10990592413273));
#57428=CARTESIAN_POINT('Ctrl Pts',(0.406787590016801,-0.672284365610765,
-1.09947196153025));
#57429=CARTESIAN_POINT('Ctrl Pts',(0.67546873968711,-0.401463918278459,
-1.08903799892777));
#57430=CARTESIAN_POINT('Ctrl Pts',(0.784945917892682,-0.03601945007418,
-1.07860403632529));
#57431=CARTESIAN_POINT('Ctrl Pts',(0.709398700781981,0.33791757944523,-1.06817007372281));
#57432=CARTESIAN_POINT('Ctrl Pts',(0.466642216044099,0.632203019823099,
-1.05773611112033));
#57433=CARTESIAN_POINT('Ctrl Pts',(0.113892415079309,0.777472895144442,
-1.04730214851785));
#57434=CARTESIAN_POINT('Ctrl Pts',(-0.265702207996823,0.73948478051424,
-1.03686818591537));
#57435=CARTESIAN_POINT('Ctrl Pts',(-0.582668673968474,0.527193314268243,
-1.02643422331289));
#57436=CARTESIAN_POINT('Ctrl Pts',(-0.762294477768732,0.190637345373097,
-1.01600026071041));
#57437=CARTESIAN_POINT('Ctrl Pts',(-0.76224039792685,-0.190853595901268,
-1.00556629810793));
#57438=CARTESIAN_POINT('Ctrl Pts',(-0.582519044847132,-0.527358571859842,
-0.995132335505446));
#57439=CARTESIAN_POINT('Ctrl Pts',(-0.265492500386352,-0.739560164195111,
-0.984698372902964));
#57440=CARTESIAN_POINT('Ctrl Pts',(0.114113134052997,-0.777440479167041,
-0.974264410300485));
#57441=CARTESIAN_POINT('Ctrl Pts',(0.46682122403901,-0.632070762133708,
-0.963830447698003));
#57442=CARTESIAN_POINT('Ctrl Pts',(0.709495166277286,-0.337716026160002,
-0.953396485095522));
#57443=CARTESIAN_POINT('Ctrl Pts',(0.784934426712148,0.0362415525744356,
-0.942962522493043));
#57444=CARTESIAN_POINT('Ctrl Pts',(0.67535726485342,0.401656656313793,-0.932528559890562));
#57445=CARTESIAN_POINT('Ctrl Pts',(0.406592046625545,0.672397510606688,
-0.922094597288081));
#57446=CARTESIAN_POINT('Ctrl Pts',(0.0419892610781171,0.784647950737613,
-0.911660634685601));
#57447=CARTESIAN_POINT('Ctrl Pts',(-0.332510788126124,0.711949492909918,
-0.90122667208312));
#57448=CARTESIAN_POINT('Ctrl Pts',(-0.628634918776022,0.471437846956661,
-0.890792709480639));
#57449=CARTESIAN_POINT('Ctrl Pts',(-0.776583889666875,0.119803868775785,
-0.88035874687816));
#57450=CARTESIAN_POINT('Ctrl Pts',(-0.741484737537108,-0.260069007488208,
-0.869924784275677));
#57451=CARTESIAN_POINT('Ctrl Pts',(-0.531610662510999,-0.578641173926874,
-0.859490821673199));
#57452=CARTESIAN_POINT('Ctrl Pts',(-0.196430956965558,-0.760822176204229,
-0.849056859070716));
#57453=CARTESIAN_POINT('Ctrl Pts',(0.185049371667793,-0.763670239503633,
-0.838622896468238));
#57454=CARTESIAN_POINT('Ctrl Pts',(0.522911823858683,-0.586514048533684,
-0.828188933865755));
#57455=CARTESIAN_POINT('Ctrl Pts',(0.737519043576373,-0.271110982847447,
-0.817754971263275));
#57456=CARTESIAN_POINT('Ctrl Pts',(0.778286091736729,0.10819549005214,-0.807321008660795));
#57457=CARTESIAN_POINT('Ctrl Pts',(0.63560379186074,0.461999268863761,-0.796887046058314));
#57458=CARTESIAN_POINT('Ctrl Pts',(0.343103703302491,0.706905477018341,
-0.786453083455834));
#57459=CARTESIAN_POINT('Ctrl Pts',(-0.030269153442102,0.785187419033389,
-0.776019120853353));
#57460=CARTESIAN_POINT('Ctrl Pts',(-0.396507286177708,0.678393305293027,
-0.765585158250872));
#57461=CARTESIAN_POINT('Ctrl Pts',(-0.669284924227368,0.411695512315086,
-0.755151195648393));
#57462=CARTESIAN_POINT('Ctrl Pts',(-0.784305814079196,0.0479572169749462,
-0.74471723304591));
#57463=CARTESIAN_POINT('Ctrl Pts',(-0.714458450750783,-0.327085045224027,
-0.734283270443432));
#57464=CARTESIAN_POINT('Ctrl Pts',(-0.476206514372981,-0.625030287527851,
-0.723849307840949));
#57465=CARTESIAN_POINT('Ctrl Pts',(-0.125708226017612,-0.775650015515965,
-0.71341534523847));
#57466=CARTESIAN_POINT('Ctrl Pts',(0.254420672919864,-0.743441743413307,
-0.702981382635988));
#57467=CARTESIAN_POINT('Ctrl Pts',(0.574580227589687,-0.535997263725662,
-0.692547420033508));
#57468=CARTESIAN_POINT('Ctrl Pts',(0.75930582132283,-0.202213190380042,
-0.682113457431027));
#57469=CARTESIAN_POINT('Ctrl Pts',(0.765055895178765,0.179234432826484,
-0.671679494828547));
#57470=CARTESIAN_POINT('Ctrl Pts',(0.590475102696554,0.518434815337383,
-0.661245532226066));
#57471=CARTESIAN_POINT('Ctrl Pts',(0.276713777796521,0.735435238369764,
-0.650811569623585));
#57472=CARTESIAN_POINT('Ctrl Pts',(-0.10227158575508,0.779086662320408,
-0.640377607021105));
#57473=CARTESIAN_POINT('Ctrl Pts',(-0.457150575148642,0.63910003622256,
-0.629943644418625));
#57474=CARTESIAN_POINT('Ctrl Pts',(-0.704274876573596,0.348471523780152,
-0.619509681816143));
#57475=CARTESIAN_POINT('Ctrl Pts',(-0.785394969112563,-0.0242950025949024,
-0.609075719213664));
#57476=CARTESIAN_POINT('Ctrl Pts',(-0.681390084391417,-0.391334968475181,
-0.598641756611182));
#57477=CARTESIAN_POINT('Ctrl Pts',(-0.416775151428219,-0.666133603573935,
-0.588207794008702));
#57478=CARTESIAN_POINT('Ctrl Pts',(-0.0539223974131361,-0.783918286376605,
-0.577773831406221));
#57479=CARTESIAN_POINT('Ctrl Pts',(0.321640372565251,-0.716926059921453,
-0.567339868803741));
#57480=CARTESIAN_POINT('Ctrl Pts',(0.621389483176351,-0.480947621738832,
-0.55690590620126));
#57481=CARTESIAN_POINT('Ctrl Pts',(0.774671251282473,-0.131605308004127,
-0.54647194359878));
#57482=CARTESIAN_POINT('Ctrl Pts',(0.745355723228447,0.248757613971936,
-0.536037980996299));
#57483=CARTESIAN_POINT('Ctrl Pts',(0.5403528445548,0.570486027909492,-0.525604018393818));
#57484=CARTESIAN_POINT('Ctrl Pts',(0.207983720877473,0.757745522262172,
-0.515170055791338));
#57485=CARTESIAN_POINT('Ctrl Pts',(-0.173409120944399,0.766397273893707,
-0.504736093188857));
#57486=CARTESIAN_POINT('Ctrl Pts',(-0.51392780284161,0.594401983614459,
-0.494302130586377));
#57487=CARTESIAN_POINT('Ctrl Pts',(-0.733308870473358,0.282300558170729,
-0.483868167983896));
#57488=CARTESIAN_POINT('Ctrl Pts',(-0.779842143925293,-0.0963417625768507,
-0.473434205381416));
#57489=CARTESIAN_POINT('Ctrl Pts',(-0.642559293212627,-0.452275424232282,
-0.463000242778934));
#57490=CARTESIAN_POINT('Ctrl Pts',(-0.353819176764376,-0.701603516818604,
-0.452566280176454));
#57491=CARTESIAN_POINT('Ctrl Pts',(0.0183194456950587,-0.785557065124961,
-0.442132317573973));
#57492=CARTESIAN_POINT('Ctrl Pts',(0.386140002593766,-0.684347428617565,
-0.431698354971493));
#57493=CARTESIAN_POINT('Ctrl Pts',(0.662943731003988,-0.42183067003324,
-0.421264392369012));
#57494=CARTESIAN_POINT('Ctrl Pts',(0.783485390069101,-0.0598844571388412,
-0.410830429766532));
#57495=CARTESIAN_POINT('Ctrl Pts',(0.719352177605271,0.316177085244022,
-0.400396467164051));
#57496=CARTESIAN_POINT('Ctrl Pts',(0.485660894669784,0.617712716434528,
-0.389962504561571));
#57497=CARTESIAN_POINT('Ctrl Pts',(0.137494773444854,0.773647653611852,
-0.37952854195909));
#57498=CARTESIAN_POINT('Ctrl Pts',(-0.243080158387669,0.747226566207261,
-0.369094579356609));
#57499=CARTESIAN_POINT('Ctrl Pts',(-0.566358811836447,0.544677152935712,
-0.358660616754129));
#57500=CARTESIAN_POINT('Ctrl Pts',(-0.756141369320216,0.213742214466799,
-0.348226654151648));
#57501=CARTESIAN_POINT('Ctrl Pts',(-0.767694298022974,-0.167573773103771,
-0.337792691549167));
#57502=CARTESIAN_POINT('Ctrl Pts',(-0.598294464011481,-0.509391047315011,
-0.327358728946687));
#57503=CARTESIAN_POINT('Ctrl Pts',(-0.287871000661499,-0.731140062743849,
-0.316924766344206));
#57504=CARTESIAN_POINT('Ctrl Pts',(0.0904063637434109,-0.78055249323209,
-0.306490803741726));
#57505=CARTESIAN_POINT('Ctrl Pts',(0.447374098176345,-0.645981361835208,
-0.296056841139245));
#57506=CARTESIAN_POINT('Ctrl Pts',(0.698891552520453,-0.359146354327071,
-0.285622878536764));
#57507=CARTESIAN_POINT('Ctrl Pts',(0.7856736973659,0.0123428316481057,-0.275188915934284));
#57508=CARTESIAN_POINT('Ctrl Pts',(0.687265167454286,0.380922683136222,
-0.264754953331803));
#57509=CARTESIAN_POINT('Ctrl Pts',(0.42686177429361,0.659715503036756,-0.254320990729322));
#57510=CARTESIAN_POINT('Ctrl Pts',(0.0658430535679579,0.783007126777561,
-0.243887028126842));
#57511=CARTESIAN_POINT('Ctrl Pts',(-0.310695504294158,0.721736709503344,
-0.233453065524361));
#57512=CARTESIAN_POINT('Ctrl Pts',(-0.614000190546963,0.490345969652932,
-0.223019102921881));
#57513=CARTESIAN_POINT('Ctrl Pts',(-0.77257930052689,0.1433764600423,-0.2125851403194));
#57514=CARTESIAN_POINT('Ctrl Pts',(-0.749054127115345,-0.237388986095524,
-0.202151177716919));
#57515=CARTESIAN_POINT('Ctrl Pts',(-0.54897001133411,-0.562198126842408,
-0.191717215114439));
#57516=CARTESIAN_POINT('Ctrl Pts',(-0.219488194761937,-0.754494815860373,
-0.181283252511958));
#57517=CARTESIAN_POINT('Ctrl Pts',(0.16172844541913,-0.768944215087348,
-0.170849289909478));
#57518=CARTESIAN_POINT('Ctrl Pts',(0.504825365157446,-0.602157589282072,
-0.160415327306997));
#57519=CARTESIAN_POINT('Ctrl Pts',(0.728927854200651,-0.293414387856205,
-0.149981364704517));
#57520=CARTESIAN_POINT('Ctrl Pts',(0.781219769114279,0.0844450113192236,
-0.139547402102036));
#57521=CARTESIAN_POINT('Ctrl Pts',(0.649362332362849,0.442490652619726,
-0.129113439499555));
#57522=CARTESIAN_POINT('Ctrl Pts',(0.459423217828204,0.611507106016679,
-0.122157464431235));
#57523=CARTESIAN_POINT('Ctrl Pts',(0.350107198737603,0.668737795639035,
-0.118679476897075));
#57524=CARTESIAN_POINT('Ctrl Pts',(-0.74085300492036,-0.114506834660713,
-1.13671995863906));
#57525=CARTESIAN_POINT('Ctrl Pts',(-0.722134886980708,-0.2356120417266,
-1.1332419711049));
#57526=CARTESIAN_POINT('Ctrl Pts',(-0.624218812318242,-0.468354692822244,
-1.12628599603658));
#57527=CARTESIAN_POINT('Ctrl Pts',(-0.330004563367702,-0.707155702503661,
-1.1158520334341));
#57528=CARTESIAN_POINT('Ctrl Pts',(0.0419121041683188,-0.779235354142127,
-1.10541807083161));
#57529=CARTESIAN_POINT('Ctrl Pts',(0.403990000027003,-0.667660918672009,
-1.09498410822914));
#57530=CARTESIAN_POINT('Ctrl Pts',(0.670823328245093,-0.39870289862725,
-1.08455014562665));
#57531=CARTESIAN_POINT('Ctrl Pts',(0.779547608102048,-0.0357717483197839,
-1.07411618302417));
#57532=CARTESIAN_POINT('Ctrl Pts',(0.704519947383167,0.335593624574007,
-1.06368222042169));
#57533=CARTESIAN_POINT('Ctrl Pts',(0.463432975704649,0.627855162501337,
-1.05324825781921));
#57534=CARTESIAN_POINT('Ctrl Pts',(0.113109141693873,0.77212597832659,-1.04281429521673));
#57535=CARTESIAN_POINT('Ctrl Pts',(-0.263874892464704,0.734399116602391,
-1.03238033261425));
#57536=CARTESIAN_POINT('Ctrl Pts',(-0.578661483474969,0.52356764518171,
-1.02194637001177));
#57537=CARTESIAN_POINT('Ctrl Pts',(-0.757051945540771,0.189326273808817,
-1.01151240740929));
#57538=CARTESIAN_POINT('Ctrl Pts',(-0.756998237707175,-0.189541037243187,
-1.00107844480681));
#57539=CARTESIAN_POINT('Ctrl Pts',(-0.578512883273855,-0.523731765804212,
-0.99064448220433));
#57540=CARTESIAN_POINT('Ctrl Pts',(-0.263666627302361,-0.734473982814123,
-0.980210519601848));
#57541=CARTESIAN_POINT('Ctrl Pts',(0.113328343147262,-0.772093783330432,
-0.969776556999368));
#57542=CARTESIAN_POINT('Ctrl Pts',(0.463610751763093,-0.627723818257466,
-0.959342594396887));
#57543=CARTESIAN_POINT('Ctrl Pts',(0.704615751113339,-0.335393449806217,
-0.948908631794406));
#57544=CARTESIAN_POINT('Ctrl Pts',(0.779536192689488,0.0359923083398992,
-0.938474669191926));
#57545=CARTESIAN_POINT('Ctrl Pts',(0.670712626473466,0.398894340692947,
-0.928040706589444));
#57546=CARTESIAN_POINT('Ctrl Pts',(0.403795788817704,0.667773227361877,
-0.917606743986965));
#57547=CARTESIAN_POINT('Ctrl Pts',(0.041700488092816,0.779251686898005,
-0.907172781384485));
#57548=CARTESIAN_POINT('Ctrl Pts',(-0.330224009781218,0.707053198590566,
-0.896738818782003));
#57549=CARTESIAN_POINT('Ctrl Pts',(-0.624311604253704,0.468195624755375,
-0.886304856179523));
#57550=CARTESIAN_POINT('Ctrl Pts',(-0.771243084840893,0.118979940943888,
-0.875870893577043));
#57551=CARTESIAN_POINT('Ctrl Pts',(-0.736385320310805,-0.258280433415595,
-0.865436930974561));
#57552=CARTESIAN_POINT('Ctrl Pts',(-0.527954613461228,-0.574661681671944,
-0.855002968372082));
#57553=CARTESIAN_POINT('Ctrl Pts',(-0.195080041221754,-0.755589769500391,
-0.8445690057696));
#57554=CARTESIAN_POINT('Ctrl Pts',(0.183776730565653,-0.758418245797769,
-0.834135043167121));
#57555=CARTESIAN_POINT('Ctrl Pts',(0.519315599381726,-0.582480412113204,
-0.823701080564639));
#57556=CARTESIAN_POINT('Ctrl Pts',(0.732446899639829,-0.269246469734522,
-0.813267117962159));
#57557=CARTESIAN_POINT('Ctrl Pts',(0.772933580346711,0.107451396589593,
-0.802833155359677));
#57558=CARTESIAN_POINT('Ctrl Pts',(0.631232550267713,0.458821958649652,
-0.792399192757198));
#57559=CARTESIAN_POINT('Ctrl Pts',(0.340744074241427,0.702043871938179,
-0.781965230154717));
#57560=CARTESIAN_POINT('Ctrl Pts',(-0.0300609832200139,0.779787445105682,
-0.771531267552236));
#57561=CARTESIAN_POINT('Ctrl Pts',(-0.393780384350699,0.673727787134543,
-0.761097304949755));
#57562=CARTESIAN_POINT('Ctrl Pts',(-0.664682047190082,0.408864156413596,
-0.750663342347275));
#57563=CARTESIAN_POINT('Ctrl Pts',(-0.778911903218282,0.0476274005323591,
-0.740229379744795));
#57564=CARTESIAN_POINT('Ctrl Pts',(-0.709544901561172,-0.324835581371784,
-0.729795417142313));
#57565=CARTESIAN_POINT('Ctrl Pts',(-0.472931496588076,-0.620731763156647,
-0.719361454539834));
#57566=CARTESIAN_POINT('Ctrl Pts',(-0.124843692115848,-0.770315633228018,
-0.708927491937352));
#57567=CARTESIAN_POINT('Ctrl Pts',(0.252670944170862,-0.7383288672593,-0.698493529334872));
#57568=CARTESIAN_POINT('Ctrl Pts',(0.570628663704239,-0.532311046678268,
-0.688059566732391));
#57569=CARTESIAN_POINT('Ctrl Pts',(0.754083843055084,-0.200822508449306,
-0.67762560412991));
#57570=CARTESIAN_POINT('Ctrl Pts',(0.759794371895204,0.178001782836496,
-0.667191641527431));
#57571=CARTESIAN_POINT('Ctrl Pts',(0.586414224895624,0.514869380616735,
-0.656757678924949));
#57572=CARTESIAN_POINT('Ctrl Pts',(0.274810732549848,0.730377425398687,
-0.64632371632247));
#57573=CARTESIAN_POINT('Ctrl Pts',(-0.101568232793435,0.773728645161736,
-0.635889753719988));
#57574=CARTESIAN_POINT('Ctrl Pts',(-0.454006610883554,0.634704749888187,
-0.625455791117508));
#57575=CARTESIAN_POINT('Ctrl Pts',(-0.699431362936916,0.346074978576616,
-0.615021828515027));
#57576=CARTESIAN_POINT('Ctrl Pts',(-0.779993567799511,-0.0241279184346039,
-0.604587865912547));
#57577=CARTESIAN_POINT('Ctrl Pts',(-0.6767039564669,-0.388643638258292,
-0.594153903310066));
#57578=CARTESIAN_POINT('Ctrl Pts',(-0.413908861295605,-0.661552399132201,
-0.583719940707586));
#57579=CARTESIAN_POINT('Ctrl Pts',(-0.0535515566010041,-0.778527040662178,
-0.573285978105104));
#57580=CARTESIAN_POINT('Ctrl Pts',(0.319428353391424,-0.711995540229179,
-0.562852015502625));
#57581=CARTESIAN_POINT('Ctrl Pts',(0.617115997729737,-0.477639997909124,
-0.552418052900143));
#57582=CARTESIAN_POINT('Ctrl Pts',(0.769343600255385,-0.130700218066689,
-0.541984090297664));
#57583=CARTESIAN_POINT('Ctrl Pts',(0.740229684050112,0.247046831810626,
-0.531550127695182));
#57584=CARTESIAN_POINT('Ctrl Pts',(0.536636672846458,0.566562621086921,
-0.521116165092702));
#57585=CARTESIAN_POINT('Ctrl Pts',(0.206553353244344,0.752534274648081,
-0.510682202490221));
#57586=CARTESIAN_POINT('Ctrl Pts',(-0.172216533405134,0.761126525538638,
-0.500248239887741));
#57587=CARTESIAN_POINT('Ctrl Pts',(-0.510393364223778,0.590314099452934,
-0.48981427728526));
#57588=CARTESIAN_POINT('Ctrl Pts',(-0.728265681184375,0.280359090927436,
-0.479380314682779));
#57589=CARTESIAN_POINT('Ctrl Pts',(-0.77447893108866,-0.0956791908220655,
-0.468946352080299));
#57590=CARTESIAN_POINT('Ctrl Pts',(-0.638140216510372,-0.449164987870472,
-0.458512389477818));
#57591=CARTESIAN_POINT('Ctrl Pts',(-0.351385854116387,-0.696778374939647,
-0.448078426875338));
#57592=CARTESIAN_POINT('Ctrl Pts',(0.0181934572664038,-0.780154549028074,
-0.437644464272857));
#57593=CARTESIAN_POINT('Ctrl Pts',(0.383484399745446,-0.679640962132688,
-0.427210501670377));
#57594=CARTESIAN_POINT('Ctrl Pts',(0.658384464291122,-0.418929611553607,
-0.416776539067895));
#57595=CARTESIAN_POINT('Ctrl Pts',(0.778097121514929,-0.0594726134192606,
-0.406342576465415));
#57596=CARTESIAN_POINT('Ctrl Pts',(0.714404972759966,0.31400263876734,-0.395908613862935));
#57597=CARTESIAN_POINT('Ctrl Pts',(0.482320856221208,0.613464517236846,
-0.385474651260454));
#57598=CARTESIAN_POINT('Ctrl Pts',(0.136549179853022,0.768327042178899,
-0.375040688657973));
#57599=CARTESIAN_POINT('Ctrl Pts',(-0.241408421824054,0.742087660669768,
-0.364606726055493));
#57600=CARTESIAN_POINT('Ctrl Pts',(-0.562463789140712,0.540931241636688,
-0.354172763453012));
#57601=CARTESIAN_POINT('Ctrl Pts',(-0.750941153956067,0.212272243912615,
-0.343738800850532));
#57602=CARTESIAN_POINT('Ctrl Pts',(-0.762414629636954,-0.166421317035277,
-0.333304838248051));
#57603=CARTESIAN_POINT('Ctrl Pts',(-0.594179810071251,-0.505887809352516,
-0.32287087564557));
#57604=CARTESIAN_POINT('Ctrl Pts',(-0.285891223784188,-0.726111789007474,
-0.31243691304309));
#57605=CARTESIAN_POINT('Ctrl Pts',(0.0897846115448724,-0.775184395108459,
-0.302002950440609));
#57606=CARTESIAN_POINT('Ctrl Pts',(0.444297369724572,-0.641538750516211,
-0.291568987838128));
#57607=CARTESIAN_POINT('Ctrl Pts',(0.694085061664188,-0.356676395059477,
-0.281135025235648));
#57608=CARTESIAN_POINT('Ctrl Pts',(0.780270379123696,0.0122579462393565,
-0.270701062633167));
#57609=CARTESIAN_POINT('Ctrl Pts',(0.682538634845942,0.378302961353548,
-0.260267100030687));
#57610=CARTESIAN_POINT('Ctrl Pts',(0.423926115256713,0.655178437904013,
-0.249833137428206));
#57611=CARTESIAN_POINT('Ctrl Pts',(0.065390230985686,0.777622147249572,
-0.239399174825725));
#57612=CARTESIAN_POINT('Ctrl Pts',(-0.308558756771416,0.716773105772149,
-0.228965212223245));
#57613=CARTESIAN_POINT('Ctrl Pts',(-0.609777522647318,0.4869737099821,-0.218531249620764));
#57614=CARTESIAN_POINT('Ctrl Pts',(-0.767266038211424,0.142390417335102,
-0.208097287018283));
#57615=CARTESIAN_POINT('Ctrl Pts',(-0.743902649484962,-0.235756391513143,
-0.197663324415803));
#57616=CARTESIAN_POINT('Ctrl Pts',(-0.545194583421667,-0.558331714416415,
-0.187229361813322));
#57617=CARTESIAN_POINT('Ctrl Pts',(-0.217978694187369,-0.749305932283903,
-0.176795399210842));
#57618=CARTESIAN_POINT('Ctrl Pts',(0.160616163563419,-0.763655935021632,
-0.166361436608361));
#57619=CARTESIAN_POINT('Ctrl Pts',(0.501353577761121,-0.59801639819481,
-0.155927474005881));
#57620=CARTESIAN_POINT('Ctrl Pts',(0.723914693935945,-0.291396426753052,
-0.1454935114034));
#57621=CARTESIAN_POINT('Ctrl Pts',(0.775847282725172,0.0838641360470794,
-0.135059548800919));
#57622=CARTESIAN_POINT('Ctrl Pts',(0.644896041046773,0.439447767297564,
-0.124625586198439));
#57623=CARTESIAN_POINT('Ctrl Pts',(0.456264301675177,0.607301174227483,
-0.117669611130118));
#57624=CARTESIAN_POINT('Ctrl Pts',(0.347699381636247,0.664138637705498,
-0.114191623595958));
#57625=CARTESIAN_POINT('Ctrl Pts',(-0.738728321778979,-0.114178441930225,
-1.13006310830201));
#57626=CARTESIAN_POINT('Ctrl Pts',(-0.720064366806756,-0.234933217536761,
-1.12658512076785));
#57627=CARTESIAN_POINT('Ctrl Pts',(-0.622428042508289,-0.467013310191969,
-1.11962914569953));
#57628=CARTESIAN_POINT('Ctrl Pts',(-0.329058258071172,-0.705126571760283,
-1.10919518309705));
#57629=CARTESIAN_POINT('Ctrl Pts',(0.0417919924060011,-0.777000845426074,
-1.09876122049457));
#57630=CARTESIAN_POINT('Ctrl Pts',(0.402831247473451,-0.665745739445225,
-1.08832725789209));
#57631=CARTESIAN_POINT('Ctrl Pts',(0.668899333621664,-0.397559476691646,
-1.0778932952896));
#57632=CARTESIAN_POINT('Ctrl Pts',(0.777311738081327,-0.0356690904367969,
-1.06745933268712));
#57633=CARTESIAN_POINT('Ctrl Pts',(0.702499287124515,0.334631062607011,
-1.05702537008464));
#57634=CARTESIAN_POINT('Ctrl Pts',(0.462103778469499,0.626054396882009,
-1.04659140748216));
#57635=CARTESIAN_POINT('Ctrl Pts',(0.112784729733045,0.769911399718676,
-1.03615744487968));
#57636=CARTESIAN_POINT('Ctrl Pts',(-0.263118061333196,0.732292755908012,
-1.0257234822772));
#57637=CARTESIAN_POINT('Ctrl Pts',(-0.577001796823254,0.522065974186611,
-1.01528951967472));
#57638=CARTESIAN_POINT('Ctrl Pts',(-0.754880609472422,0.18878325923917,
-1.00485555707224));
#57639=CARTESIAN_POINT('Ctrl Pts',(-0.754827055346663,-0.188997406198552,
-0.994421594469759));
#57640=CARTESIAN_POINT('Ctrl Pts',(-0.57685362332253,-0.522229625831563,
-0.98398763186728));
#57641=CARTESIAN_POINT('Ctrl Pts',(-0.262910392619023,-0.732367403574914,
-0.973553669264798));
#57642=CARTESIAN_POINT('Ctrl Pts',(0.113003300781565,-0.769879304770087,
-0.963119706662318));
#57643=CARTESIAN_POINT('Ctrl Pts',(0.462281047969407,-0.625923414086448,
-0.952685744059838));
#57644=CARTESIAN_POINT('Ctrl Pts',(0.702594809534995,-0.334431492061374,
-0.942251781457356));
#57645=CARTESIAN_POINT('Ctrl Pts',(0.777300368274831,0.035889077098665,
-0.931817818854877));
#57646=CARTESIAN_POINT('Ctrl Pts',(0.668788924044229,0.397750253078557,
-0.921383856252395));
#57647=CARTESIAN_POINT('Ctrl Pts',(0.40263764312539,0.665857955560153,-0.910949893649916));
#57648=CARTESIAN_POINT('Ctrl Pts',(0.0415808849614484,0.777016678487024,
-0.900515931047433));
#57649=CARTESIAN_POINT('Ctrl Pts',(-0.329276878767881,0.705025266057697,
-0.890081968444955));
#57650=CARTESIAN_POINT('Ctrl Pts',(-0.62252098677963,0.466852770864623,
-0.879648005842472));
#57651=CARTESIAN_POINT('Ctrl Pts',(-0.769031046276919,0.118638688979372,
-0.869214043239994));
#57652=CARTESIAN_POINT('Ctrl Pts',(-0.734273258940724,-0.257539647157259,
-0.858780080637511));
#57653=CARTESIAN_POINT('Ctrl Pts',(-0.526440362004134,-0.573013467475886,
-0.848346118035032));
#57654=CARTESIAN_POINT('Ctrl Pts',(-0.194520522980727,-0.753422626946348,
-0.837912155432552));
#57655=CARTESIAN_POINT('Ctrl Pts',(0.183249631881523,-0.756242990757862,
-0.82747819283007));
#57656=CARTESIAN_POINT('Ctrl Pts',(0.517826125887222,-0.5808097726486,-0.81704423022759));
#57657=CARTESIAN_POINT('Ctrl Pts',(0.730346134239288,-0.268474231271757,
-0.806610267625109));
#57658=CARTESIAN_POINT('Ctrl Pts',(0.770716693193102,0.107143210185493,
-0.796176305022629));
#57659=CARTESIAN_POINT('Ctrl Pts',(0.629422082502814,0.457505989811208,
-0.785742342420148));
#57660=CARTESIAN_POINT('Ctrl Pts',(0.33976677013657,0.700030306891271,-0.775308379817668));
#57661=CARTESIAN_POINT('Ctrl Pts',(-0.0299747639002427,0.777550900060216,
-0.764874417215187));
#57662=CARTESIAN_POINT('Ctrl Pts',(-0.392650964310472,0.671795436782193,
-0.754440454612706));
#57663=CARTESIAN_POINT('Ctrl Pts',(-0.662775641349895,0.40769147389731,
-0.744006492010226));
#57664=CARTESIAN_POINT('Ctrl Pts',(-0.776677869355681,0.0474907981449293,
-0.733572529407746));
#57665=CARTESIAN_POINT('Ctrl Pts',(-0.70750982245842,-0.323903905163519,
-0.723138566805264));
#57666=CARTESIAN_POINT('Ctrl Pts',(-0.471575059520285,-0.618951413193122,
-0.712704604202784));
#57667=CARTESIAN_POINT('Ctrl Pts',(-0.124485622050971,-0.768106254731666,
-0.702270641600303));
#57668=CARTESIAN_POINT('Ctrl Pts',(0.251946246752527,-0.736211231510793,
-0.691836678997822));
#57669=CARTESIAN_POINT('Ctrl Pts',(0.56899201679665,-0.530784300330185,
-0.681402716395342));
#57670=CARTESIAN_POINT('Ctrl Pts',(0.751921019719525,-0.200246519967946,
-0.670968753792861));
#57671=CARTESIAN_POINT('Ctrl Pts',(0.757615169923306,0.177491247551546,
-0.66053479119038));
#57672=CARTESIAN_POINT('Ctrl Pts',(0.584732302677573,0.513392659531383,
-0.6501008285879));
#57673=CARTESIAN_POINT('Ctrl Pts',(0.274022534963207,0.728282595554542,
-0.639666865985419));
#57674=CARTESIAN_POINT('Ctrl Pts',(-0.101276920168108,0.771509477645341,
-0.629232903382939));
#57675=CARTESIAN_POINT('Ctrl Pts',(-0.452704453170509,0.632884323344254,
-0.618798940780458));
#57676=CARTESIAN_POINT('Ctrl Pts',(-0.697425290949942,0.345082384654319,
-0.608364978177977));
#57677=CARTESIAN_POINT('Ctrl Pts',(-0.777756431563853,-0.0240587160169824,
-0.597931015575497));
#57678=CARTESIAN_POINT('Ctrl Pts',(-0.674763070023314,-0.387528951161117,
-0.587497052973016));
#57679=CARTESIAN_POINT('Ctrl Pts',(-0.412721709823989,-0.659654969582801,
-0.577063090370536));
#57680=CARTESIAN_POINT('Ctrl Pts',(-0.0533979628629348,-0.776294110641974,
-0.566629127768055));
#57681=CARTESIAN_POINT('Ctrl Pts',(0.318512185908037,-0.709953432334409,
-0.556195165165575));
#57682=CARTESIAN_POINT('Ctrl Pts',(0.615346018313085,-0.476270056167249,
-0.545761202563094));
#57683=CARTESIAN_POINT('Ctrl Pts',(0.767137009692519,-0.130325350624294,
-0.535327239960614));
#57684=CARTESIAN_POINT('Ctrl Pts',(0.738106596479569,0.246338265173458,
-0.524893277358132));
#57685=CARTESIAN_POINT('Ctrl Pts',(0.535097519966525,0.564937636187393,
-0.514459314755653));
#57686=CARTESIAN_POINT('Ctrl Pts',(0.205960927857499,0.750375895702547,
-0.504025352153171));
#57687=CARTESIAN_POINT('Ctrl Pts',(-0.171722591066164,0.758943502754222,
-0.493591389550691));
#57688=CARTESIAN_POINT('Ctrl Pts',(-0.508929481011554,0.58862099182125,
-0.48315742694821));
#57689=CARTESIAN_POINT('Ctrl Pts',(-0.726176908133129,0.279554979833187,
-0.47272346434573));
#57690=CARTESIAN_POINT('Ctrl Pts',(-0.772257611641911,-0.0954047688349832,
-0.462289501743249));
#57691=CARTESIAN_POINT('Ctrl Pts',(-0.636309936543045,-0.447876716644097,
-0.451855539140768));
#57692=CARTESIAN_POINT('Ctrl Pts',(-0.35037802782218,-0.69477991211232,
-0.441421576538288));
#57693=CARTESIAN_POINT('Ctrl Pts',(0.0181412757559645,-0.777916951074585,
-0.430987613935807));
#57694=CARTESIAN_POINT('Ctrl Pts',(0.382384510102889,-0.677691651925019,
-0.420553651333326));
#57695=CARTESIAN_POINT('Ctrl Pts',(0.65649612084464,-0.41772805983205,-0.410119688730846));
#57696=CARTESIAN_POINT('Ctrl Pts',(0.775865424566032,-0.0593020372196476,
-0.399685726128365));
#57697=CARTESIAN_POINT('Ctrl Pts',(0.712355954258471,0.313102033031223,
-0.389251763525885));
#57698=CARTESIAN_POINT('Ctrl Pts',(0.480937489089394,0.61170501080317,-0.378817800923404));
#57699=CARTESIAN_POINT('Ctrl Pts',(0.13615753672838,0.766123367253981,-0.368383838320923));
#57700=CARTESIAN_POINT('Ctrl Pts',(-0.240716026976013,0.739959244149259,
-0.357949875718443));
#57701=CARTESIAN_POINT('Ctrl Pts',(-0.56085056029334,0.539379771301716,
-0.347515913115962));
#57702=CARTESIAN_POINT('Ctrl Pts',(-0.748787344315943,0.2116634159071,-0.337081950513482));
#57703=CARTESIAN_POINT('Ctrl Pts',(-0.760227912378572,-0.165943996230152,
-0.326647987911001));
#57704=CARTESIAN_POINT('Ctrl Pts',(-0.592475615017111,-0.504436848731719,
-0.31621402530852));
#57705=CARTESIAN_POINT('Ctrl Pts',(-0.285071245711685,-0.724029193640402,
-0.30578006270604));
#57706=CARTESIAN_POINT('Ctrl Pts',(0.0895270960624426,-0.772961052277887,
-0.295346100103559));
#57707=CARTESIAN_POINT('Ctrl Pts',(0.443023059573035,-0.639698723071945,
-0.284912137501079));
#57708=CARTESIAN_POINT('Ctrl Pts',(0.692094323595702,-0.355653394680001,
-0.274478174898598));
#57709=CARTESIAN_POINT('Ctrl Pts',(0.778032449069809,0.0122227885764639,
-0.264044212296118));
#57710=CARTESIAN_POINT('Ctrl Pts',(0.680581013455967,0.377217932977417,
-0.253610249693637));
#57711=CARTESIAN_POINT('Ctrl Pts',(0.422710233282295,0.653299289538508,
-0.243176287091156));
#57712=CARTESIAN_POINT('Ctrl Pts',(0.0652026812946528,0.775391813136049,
-0.232742324488676));
#57713=CARTESIAN_POINT('Ctrl Pts',(-0.307673763129744,0.714717294055671,
-0.222308361886195));
#57714=CARTESIAN_POINT('Ctrl Pts',(-0.608028594518636,0.485576999870035,
-0.211874399283715));
#57715=CARTESIAN_POINT('Ctrl Pts',(-0.765065399588575,0.141982016572882,
-0.201440436681234));
#57716=CARTESIAN_POINT('Ctrl Pts',(-0.741769040716875,-0.235080199432132,
-0.191006474078753));
#57717=CARTESIAN_POINT('Ctrl Pts',(-0.543630858812925,-0.556730352880343,
-0.180572511476273));
#57718=CARTESIAN_POINT('Ctrl Pts',(-0.217353551159851,-0.747156781385142,
-0.170138548873792));
#57719=CARTESIAN_POINT('Ctrl Pts',(0.160155594960686,-0.761465719142779,
-0.159704586271311));
#57720=CARTESIAN_POINT('Ctrl Pts',(0.49991542084712,-0.596301077920988,
-0.149270623668831));
#57721=CARTESIAN_POINT('Ctrl Pts',(0.72183879696572,-0.290560898293592,
-0.13883666106635));
#57722=CARTESIAN_POINT('Ctrl Pts',(0.773621246330563,0.0836240792666318,
-0.12840269846387));
#57723=CARTESIAN_POINT('Ctrl Pts',(0.643048073335987,0.438186347774592,
-0.117968735861389));
#57724=CARTESIAN_POINT('Ctrl Pts',(0.454952994195824,0.605560964824554,
-0.111012760793069));
#57725=CARTESIAN_POINT('Ctrl Pts',(0.346702218893402,0.662233962746091,
-0.107534773258908));
#57726=CARTESIAN_POINT('Ctrl Pts',(-0.738728321778979,-0.114178441930225,
-1.12625));
#57727=CARTESIAN_POINT('Ctrl Pts',(-0.720064014057808,-0.234935499803312,
-1.12277201246584));
#57728=CARTESIAN_POINT('Ctrl Pts',(-0.622428467720147,-0.467011987146758,
-1.11581603739752));
#57729=CARTESIAN_POINT('Ctrl Pts',(-0.329058176975973,-0.705127368582215,
-1.10538207479504));
#57730=CARTESIAN_POINT('Ctrl Pts',(0.0417919283474016,-0.77700066177415,
-1.09494811219256));
#57731=CARTESIAN_POINT('Ctrl Pts',(0.402831360764571,-0.66574603450436,
-1.08451414959008));
#57732=CARTESIAN_POINT('Ctrl Pts',(0.66889944257465,-0.397559467050142,
-1.0740801869876));
#57733=CARTESIAN_POINT('Ctrl Pts',(0.77731189566657,-0.0356691406410475,
-1.06364622438512));
#57734=CARTESIAN_POINT('Ctrl Pts',(0.70249941623784,0.334631148448006,-1.05321226178264));
#57735=CARTESIAN_POINT('Ctrl Pts',(0.462103868983754,0.626054505003761,
-1.04277829918016));
#57736=CARTESIAN_POINT('Ctrl Pts',(0.112784749994043,0.769911552166373,
-1.03234433657767));
#57737=CARTESIAN_POINT('Ctrl Pts',(-0.263118110857165,0.732292892594137,
-1.02191037397519));
#57738=CARTESIAN_POINT('Ctrl Pts',(-0.577001907123833,0.522066075167691,
-1.01147641137271));
#57739=CARTESIAN_POINT('Ctrl Pts',(-0.754880753196469,0.188783294475205,
-1.00104244877023));
#57740=CARTESIAN_POINT('Ctrl Pts',(-0.754827199305279,-0.188997441843078,
-0.990608486167753));
#57741=CARTESIAN_POINT('Ctrl Pts',(-0.576853733233579,-0.522229725565813,
-0.980174523565272));
#57742=CARTESIAN_POINT('Ctrl Pts',(-0.262910442753169,-0.732367543071951,
-0.969740560962791));
#57743=CARTESIAN_POINT('Ctrl Pts',(0.113003322331731,-0.769879451565163,
-0.95930659836031));
#57744=CARTESIAN_POINT('Ctrl Pts',(0.462281136078411,-0.625923533367173,
-0.948872635757831));
#57745=CARTESIAN_POINT('Ctrl Pts',(0.70259494345804,-0.334431555819595,
-0.938438673155348));
#57746=CARTESIAN_POINT('Ctrl Pts',(0.777300516433144,0.0358890839459567,
-0.928004710552869));
#57747=CARTESIAN_POINT('Ctrl Pts',(0.668789051521525,0.397750328889645,
-0.917570747950388));
#57748=CARTESIAN_POINT('Ctrl Pts',(0.402637719871012,0.665858082479752,
-0.907136785347908));
#57749=CARTESIAN_POINT('Ctrl Pts',(0.0415808928872875,0.777016826591824,
-0.896702822745427));
#57750=CARTESIAN_POINT('Ctrl Pts',(-0.32927694153081,0.705025400441648,
-0.886268860142946));
#57751=CARTESIAN_POINT('Ctrl Pts',(-0.622521105437113,0.466852859850313,
-0.875834897540466));
#57752=CARTESIAN_POINT('Ctrl Pts',(-0.769031192860477,0.118638711592977,
-0.865400934937984));
#57753=CARTESIAN_POINT('Ctrl Pts',(-0.73427339889913,-0.257539696246454,
-0.854966972335505));
#57754=CARTESIAN_POINT('Ctrl Pts',(-0.526440462347929,-0.573013576696856,
-0.844533009733024));
#57755=CARTESIAN_POINT('Ctrl Pts',(-0.194520560057908,-0.753422770554805,
-0.834099047130543));
#57756=CARTESIAN_POINT('Ctrl Pts',(0.183249666810382,-0.756243134903882,
-0.823665084528063));
#57757=CARTESIAN_POINT('Ctrl Pts',(0.517826224589069,-0.580809883355641,
-0.813231121925582));
#57758=CARTESIAN_POINT('Ctrl Pts',(0.730346273449163,-0.268474282445114,
-0.802797159323102));
#57759=CARTESIAN_POINT('Ctrl Pts',(0.770716840097935,0.107143230607854,
-0.79236319672062));
#57760=CARTESIAN_POINT('Ctrl Pts',(0.62942220247575,0.457506077015547,-0.781929234118141));
#57761=CARTESIAN_POINT('Ctrl Pts',(0.339766834898864,0.700030440322706,
-0.77149527151566));
#57762=CARTESIAN_POINT('Ctrl Pts',(-0.0299747696136753,0.777551048267701,
-0.761061308913179));
#57763=CARTESIAN_POINT('Ctrl Pts',(-0.392651039152919,0.671795564831833,
-0.750627346310698));
#57764=CARTESIAN_POINT('Ctrl Pts',(-0.66277576768029,0.4076915516066,-0.740193383708219));
#57765=CARTESIAN_POINT('Ctrl Pts',(-0.776678017396761,0.0474908071970595,
-0.729759421105736));
#57766=CARTESIAN_POINT('Ctrl Pts',(-0.707509957315512,-0.323903966902222,
-0.719325458503257));
#57767=CARTESIAN_POINT('Ctrl Pts',(-0.471575149406303,-0.618951531170264,
-0.708891495900775));
#57768=CARTESIAN_POINT('Ctrl Pts',(-0.124485645778937,-0.768106401138926,
-0.698457533298296));
#57769=CARTESIAN_POINT('Ctrl Pts',(0.251946294775518,-0.736211371838604,
-0.688023570695814));
#57770=CARTESIAN_POINT('Ctrl Pts',(0.568992125251127,-0.530784401501963,
-0.677589608093334));
#57771=CARTESIAN_POINT('Ctrl Pts',(0.751921163041749,-0.200246558136551,
-0.667155645490854));
#57772=CARTESIAN_POINT('Ctrl Pts',(0.757615314330881,0.177491281382813,
-0.656721682888373));
#57773=CARTESIAN_POINT('Ctrl Pts',(0.584732414132277,0.513392757388173,
-0.646287720285892));
#57774=CARTESIAN_POINT('Ctrl Pts',(0.274022587194117,0.728282734371093,
-0.635853757683412));
#57775=CARTESIAN_POINT('Ctrl Pts',(-0.101276939472307,0.771509624701283,
-0.625419795080931));
#57776=CARTESIAN_POINT('Ctrl Pts',(-0.452704539459636,0.632884443977122,
-0.61498583247845));
#57777=CARTESIAN_POINT('Ctrl Pts',(-0.69742542388484,0.345082450429811,
-0.60455186987597));
#57778=CARTESIAN_POINT('Ctrl Pts',(-0.777756579810515,-0.0240587206027681,
-0.594117907273489));
#57779=CARTESIAN_POINT('Ctrl Pts',(-0.674763198638609,-0.387529025027267,
-0.583683944671009));
#57780=CARTESIAN_POINT('Ctrl Pts',(-0.412721788492083,-0.659655095318369,
-0.573249982068528));
#57781=CARTESIAN_POINT('Ctrl Pts',(-0.0533979730410179,-0.776294258609907,
-0.562816019466048));
#57782=CARTESIAN_POINT('Ctrl Pts',(0.318512246619034,-0.709953567657271,
-0.552382056863567));
#57783=CARTESIAN_POINT('Ctrl Pts',(0.615346135603011,-0.476270146948171,
-0.541948094261087));
#57784=CARTESIAN_POINT('Ctrl Pts',(0.767137155915032,-0.130325375465359,
-0.531514131658606));
#57785=CARTESIAN_POINT('Ctrl Pts',(0.738106737168653,0.246338312127523,
-0.521080169056125));
#57786=CARTESIAN_POINT('Ctrl Pts',(0.535097621960437,0.564937743869073,
-0.510646206453644));
#57787=CARTESIAN_POINT('Ctrl Pts',(0.205960967115317,0.750376038730258,
-0.500212243851164));
#57788=CARTESIAN_POINT('Ctrl Pts',(-0.171722623797879,0.758943647414989,
-0.489778281248683));
#57789=CARTESIAN_POINT('Ctrl Pts',(-0.508929578017626,0.588621104017168,
-0.479344318646203));
#57790=CARTESIAN_POINT('Ctrl Pts',(-0.726177046548319,0.279555033118626,
-0.468910356043722));
#57791=CARTESIAN_POINT('Ctrl Pts',(-0.772257758840452,-0.0954047870199036,
-0.458476393441242));
#57792=CARTESIAN_POINT('Ctrl Pts',(-0.636310057828864,-0.447876802013019,
-0.448042430838761));
#57793=CARTESIAN_POINT('Ctrl Pts',(-0.350378094607062,-0.694780044542988,
-0.43760846823628));
#57794=CARTESIAN_POINT('Ctrl Pts',(0.018141279213836,-0.777917099351843,
-0.4271745056338));
#57795=CARTESIAN_POINT('Ctrl Pts',(0.382384582988471,-0.677691781098527,
-0.416740543031318));
#57796=CARTESIAN_POINT('Ctrl Pts',(0.656496245978099,-0.417728139454391,
-0.406306580428839));
#57797=CARTESIAN_POINT('Ctrl Pts',(0.775865572452268,-0.0593020485231031,
-0.395872617826358));
#57798=CARTESIAN_POINT('Ctrl Pts',(0.712356090039248,0.313102092711016,
-0.385438655223878));
#57799=CARTESIAN_POINT('Ctrl Pts',(0.480937580760017,0.611705127399059,
-0.375004692621396));
#57800=CARTESIAN_POINT('Ctrl Pts',(0.136157562681009,0.766123513283346,
-0.364570730018916));
#57801=CARTESIAN_POINT('Ctrl Pts',(-0.240716072858239,0.739959385191355,
-0.354136767416435));
#57802=CARTESIAN_POINT('Ctrl Pts',(-0.560850667196372,0.539379874112091,
-0.343702804813955));
#57803=CARTESIAN_POINT('Ctrl Pts',(-0.74878748704011,0.211663456251404,
-0.333268842211474));
#57804=CARTESIAN_POINT('Ctrl Pts',(-0.760228057285639,-0.165944027859526,
-0.322834879608993));
#57805=CARTESIAN_POINT('Ctrl Pts',(-0.592475727944838,-0.504436944883217,
-0.312400917006513));
#57806=CARTESIAN_POINT('Ctrl Pts',(-0.285071300054302,-0.724029331642761,
-0.301966954404033));
#57807=CARTESIAN_POINT('Ctrl Pts',(0.0895271131383138,-0.772961199617316,
-0.291532991801552));
#57808=CARTESIAN_POINT('Ctrl Pts',(0.443023143994609,-0.639698844990302,
-0.281099029199071));
#57809=CARTESIAN_POINT('Ctrl Pts',(0.692094455558162,-0.355653462496763,
-0.270665066596591));
#57810=CARTESIAN_POINT('Ctrl Pts',(0.778032597283113,0.0122227909580791,
-0.26023110399411));
#57811=CARTESIAN_POINT('Ctrl Pts',(0.68058114334938,0.377218004776167,-0.249797141391629));
#57812=CARTESIAN_POINT('Ctrl Pts',(0.42271031352139,0.65329941426342,-0.239363178789149));
#57813=CARTESIAN_POINT('Ctrl Pts',(0.0652026943778764,0.775391960536891,
-0.228929216186668));
#57814=CARTESIAN_POINT('Ctrl Pts',(-0.307673823063886,0.714717431064047,
-0.218495253584187));
#57815=CARTESIAN_POINT('Ctrl Pts',(-0.608028707877244,0.485577090895009,
-0.208061290981707));
#57816=CARTESIAN_POINT('Ctrl Pts',(-0.765065550407648,0.141982046646383,
-0.197627328379226));
#57817=CARTESIAN_POINT('Ctrl Pts',(-0.741769172281945,-0.235080250164528,
-0.187193365776746));
#57818=CARTESIAN_POINT('Ctrl Pts',(-0.543630981761295,-0.556730447339991,
-0.176759403174265));
#57819=CARTESIAN_POINT('Ctrl Pts',(-0.217353554555276,-0.747156946739449,
-0.166325440571785));
#57820=CARTESIAN_POINT('Ctrl Pts',(0.160155550638935,-0.76146581913925,
-0.155891477969304));
#57821=CARTESIAN_POINT('Ctrl Pts',(0.499915663487163,-0.596301280456369,
-0.145457515366823));
#57822=CARTESIAN_POINT('Ctrl Pts',(0.721838643854927,-0.290560778341026,
-0.135023552764342));
#57823=CARTESIAN_POINT('Ctrl Pts',(0.7736219742308,0.0836237451066917,-0.124589590161862));
#57824=CARTESIAN_POINT('Ctrl Pts',(0.643046958594169,0.43818717759652,-0.114155627559381));
#57825=CARTESIAN_POINT('Ctrl Pts',(0.454955040136635,0.605559893704287,
-0.107199652491061));
#57826=CARTESIAN_POINT('Ctrl Pts',(0.346702218893402,0.662233962746091,
-0.103721664956901));
#57827=CARTESIAN_POINT('',(0.351283760559806,0.670985139773179,-0.12));
#57828=CARTESIAN_POINT('Ctrl Pts',(0.70874660020474,0.237559480337499,-0.12));
#57829=CARTESIAN_POINT('Ctrl Pts',(0.677871308579866,0.329674339059915,
-0.12));
#57830=CARTESIAN_POINT('Ctrl Pts',(0.630004482514656,0.41492357712479,-0.12));
#57831=CARTESIAN_POINT('Ctrl Pts',(0.488745407170175,0.583538685988193,
-0.12));
#57832=CARTESIAN_POINT('Ctrl Pts',(0.40457236631853,0.63931629107315,-0.12));
#57833=CARTESIAN_POINT('Ctrl Pts',(0.351283760559796,0.670985139773185,
-0.12));
#57834=CARTESIAN_POINT('Ctrl Pts',(-0.459745842892912,-0.601806928197387,
-1.12625));
#57835=CARTESIAN_POINT('Ctrl Pts',(-0.416468302643136,-0.634888226084004,
-1.12472013661271));
#57836=CARTESIAN_POINT('Ctrl Pts',(-0.263250172568355,-0.728042154867829,
-1.11971228569127));
#57837=CARTESIAN_POINT('Ctrl Pts',(0.0423441932323904,-0.787268438306116,
-1.11122644723566));
#57838=CARTESIAN_POINT('Ctrl Pts',(0.40815462829301,-0.674543622261523,
-1.10079248463318));
#57839=CARTESIAN_POINT('Ctrl Pts',(0.677738701453825,-0.402813068451867,
-1.0903585220307));
#57840=CARTESIAN_POINT('Ctrl Pts',(0.787583785039378,-0.0361404951497466,
-1.07992455942822));
#57841=CARTESIAN_POINT('Ctrl Pts',(0.711782686348956,0.339053175380459,
-1.06949059682573));
#57842=CARTESIAN_POINT('Ctrl Pts',(0.468210400798602,0.634327583870298,
-1.05905663422325));
#57843=CARTESIAN_POINT('Ctrl Pts',(0.114275158775044,0.780085648735315,
-1.04862267162077));
#57844=CARTESIAN_POINT('Ctrl Pts',(-0.266595119432196,0.741969872482332,
-1.03818870901829));
#57845=CARTESIAN_POINT('Ctrl Pts',(-0.584626774041369,0.528964985372609,
-1.02775474641581));
#57846=CARTESIAN_POINT('Ctrl Pts',(-0.764856223313064,0.191277995929144,
-1.01732078381333));
#57847=CARTESIAN_POINT('Ctrl Pts',(-0.764801961726998,-0.191494973175325,
-1.00688682121085));
#57848=CARTESIAN_POINT('Ctrl Pts',(-0.584476642087926,-0.529130798350251,
-0.996452858608371));
#57849=CARTESIAN_POINT('Ctrl Pts',(-0.26638470707097,-0.742045509438615,
-0.98601889600589));
#57850=CARTESIAN_POINT('Ctrl Pts',(0.114496619465382,-0.780053123936527,
-0.975584933403409));
#57851=CARTESIAN_POINT('Ctrl Pts',(0.468390010412389,-0.634194881491945,
-0.965150970800929));
#57852=CARTESIAN_POINT('Ctrl Pts',(0.711879475926061,-0.338850945209242,
-0.954717008198449));
#57853=CARTESIAN_POINT('Ctrl Pts',(0.787572255433586,0.0363633449241294,
-0.944283045595967));
#57854=CARTESIAN_POINT('Ctrl Pts',(0.67762685162374,0.403006452460029,-0.933849082993488));
#57855=CARTESIAN_POINT('Ctrl Pts',(0.40795842850662,0.674657150909492,-0.923415120391005));
#57856=CARTESIAN_POINT('Ctrl Pts',(0.0421303690166799,0.78728481673588,
-0.912981157788527));
#57857=CARTESIAN_POINT('Ctrl Pts',(-0.333628214598002,0.714342050500303,
-0.902547195186044));
#57858=CARTESIAN_POINT('Ctrl Pts',(-0.630747491734475,0.473022147824028,
-0.892113232583565));
#57859=CARTESIAN_POINT('Ctrl Pts',(-0.779193655806612,0.120206478312629,
-0.881679269981084));
#57860=CARTESIAN_POINT('Ctrl Pts',(-0.743976550446063,-0.260942988134431,
-0.871245307378603));
#57861=CARTESIAN_POINT('Ctrl Pts',(-0.53339717846247,-0.58058573930206,
-0.860811344776123));
#57862=CARTESIAN_POINT('Ctrl Pts',(-0.197091077355778,-0.763378973969725,
-0.850377382173642));
#57863=CARTESIAN_POINT('Ctrl Pts',(0.1856712434202,-0.766236608391143,-0.839943419571162));
#57864=CARTESIAN_POINT('Ctrl Pts',(0.524669106735824,-0.588485071271487,
-0.829509456968681));
#57865=CARTESIAN_POINT('Ctrl Pts',(0.739997529484913,-0.272022070847804,
-0.8190754943662));
#57866=CARTESIAN_POINT('Ctrl Pts',(0.780901578249223,0.108559088795519,
-0.80864153176372));
#57867=CARTESIAN_POINT('Ctrl Pts',(0.63773978421953,0.463551850709081,-0.798207569161239));
#57868=CARTESIAN_POINT('Ctrl Pts',(0.34425672802939,0.709281083829745,-0.787773606558759));
#57869=CARTESIAN_POINT('Ctrl Pts',(-0.0303708751141361,0.787826097953732,
-0.777339643956278));
#57870=CARTESIAN_POINT('Ctrl Pts',(-0.397839777494351,0.680673094896104,
-0.766905681353797));
#57871=CARTESIAN_POINT('Ctrl Pts',(-0.671534104459314,0.413079044760477,
-0.756471718751318));
#57872=CARTESIAN_POINT('Ctrl Pts',(-0.786941530302541,0.0481183806594918,
-0.746037756148836));
#57873=CARTESIAN_POINT('Ctrl Pts',(-0.716859439874856,-0.328184238095781,
-0.735603793546357));
#57874=CARTESIAN_POINT('Ctrl Pts',(-0.477806840690935,-0.627130746863161,
-0.725169830943874));
#57875=CARTESIAN_POINT('Ctrl Pts',(-0.126130677572574,-0.778256643304304,
-0.714735868341395));
#57876=CARTESIAN_POINT('Ctrl Pts',(0.255275671930622,-0.745940132981574,
-0.704301905738913));
#57877=CARTESIAN_POINT('Ctrl Pts',(0.576511145861981,-0.537798521166715,
-0.693867943136434));
#57878=CARTESIAN_POINT('Ctrl Pts',(0.761857523268443,-0.202892742382452,
-0.683433980533952));
#57879=CARTESIAN_POINT('Ctrl Pts',(0.767626920662054,0.179836763057757,
-0.673000017931472));
#57880=CARTESIAN_POINT('Ctrl Pts',(0.592459436842396,0.520177052904672,
-0.662566055328991));
#57881=CARTESIAN_POINT('Ctrl Pts',(0.277643694393171,0.7379067215007,-0.652132092726511));
#57882=CARTESIAN_POINT('Ctrl Pts',(-0.102615276791054,0.781704839208057,
-0.64169813012403));
#57883=CARTESIAN_POINT('Ctrl Pts',(-0.458686862609225,0.641247777962548,
-0.63126416752155));
#57884=CARTESIAN_POINT('Ctrl Pts',(-0.706641643062582,0.349642587454695,
-0.620830204919068));
#57885=CARTESIAN_POINT('Ctrl Pts',(-0.788034345519909,-0.0243766477023798,
-0.610396242316589));
#57886=CARTESIAN_POINT('Ctrl Pts',(-0.683679944886671,-0.392650077845349,
-0.599962279714108));
#57887=CARTESIAN_POINT('Ctrl Pts',(-0.418175754367006,-0.668372193565669,
-0.589528317111627));
#57888=CARTESIAN_POINT('Ctrl Pts',(-0.0541036075165322,-0.786552700285172,
-0.579094354509147));
#57889=CARTESIAN_POINT('Ctrl Pts',(0.322721268222067,-0.719335341624016,
-0.568660391906666));
#57890=CARTESIAN_POINT('Ctrl Pts',(0.623477707326197,-0.482563880889843,
-0.558226429304186));
#57891=CARTESIAN_POINT('Ctrl Pts',(0.777274589863052,-0.132047577128183,
-0.547792466701705));
#57892=CARTESIAN_POINT('Ctrl Pts',(0.747860544863849,0.249593581864889,
-0.537358504099224));
#57893=CARTESIAN_POINT('Ctrl Pts',(0.542168739239193,0.572403187328638,
-0.526924541496743));
#57894=CARTESIAN_POINT('Ctrl Pts',(0.208682665163577,0.760291980710321,
-0.516490578894263));
#57895=CARTESIAN_POINT('Ctrl Pts',(-0.173991874795186,0.768972807176858,
-0.506056616291782));
#57896=CARTESIAN_POINT('Ctrl Pts',(-0.515654894268529,0.596399514326687,
-0.495622653689302));
#57897=CARTESIAN_POINT('Ctrl Pts',(-0.735773207791702,0.283249249545539,
-0.485188691086821));
#57898=CARTESIAN_POINT('Ctrl Pts',(-0.782462859663332,-0.0966655260145957,
-0.47475472848434));
#57899=CARTESIAN_POINT('Ctrl Pts',(-0.644718660035084,-0.453795328396793,
-0.46432076588186));
#57900=CARTESIAN_POINT('Ctrl Pts',(-0.355008211612248,-0.703961306010574,
-0.453886803279379));
#57901=CARTESIAN_POINT('Ctrl Pts',(0.018381009512838,-0.788196986267641,
-0.443452840676898));
#57902=CARTESIAN_POINT('Ctrl Pts',(0.387437653906621,-0.686647227481264,
-0.433018878074418));
#57903=CARTESIAN_POINT('Ctrl Pts',(0.665171601199015,-0.423248262406717,
-0.422584915471937));
#57904=CARTESIAN_POINT('Ctrl Pts',(0.786118349198422,-0.0600857031737081,
-0.412150952869458));
#57905=CARTESIAN_POINT('Ctrl Pts',(0.721769612451193,0.317239621129983,
-0.401716990266976));
#57906=CARTESIAN_POINT('Ctrl Pts',(0.487292993114226,0.619788584544707,
-0.391283027664496));
#57907=CARTESIAN_POINT('Ctrl Pts',(0.137956834542056,0.776247552318673,
-0.380849065062015));
#57908=CARTESIAN_POINT('Ctrl Pts',(-0.243897046781887,0.749737674945353,
-0.370415102459534));
#57909=CARTESIAN_POINT('Ctrl Pts',(-0.56826210144847,0.546507579770122,
-0.359981139857054));
#57910=CARTESIAN_POINT('Ctrl Pts',(-0.758682436896786,0.214460510585709,
-0.349547177254573));
#57911=CARTESIAN_POINT('Ctrl Pts',(-0.770274190049176,-0.168136916847529,
-0.339113214652093));
#57912=CARTESIAN_POINT('Ctrl Pts',(-0.600305075684723,-0.511102892647924,
-0.328679252049612));
#57913=CARTESIAN_POINT('Ctrl Pts',(-0.288838411909716,-0.733597111627555,
-0.318245289447132));
#57914=CARTESIAN_POINT('Ctrl Pts',(0.0907101808453047,-0.783175596150041,
-0.307811326844651));
#57915=CARTESIAN_POINT('Ctrl Pts',(0.448877531081795,-0.648152228766215,
-0.29737736424217));
#57916=CARTESIAN_POINT('Ctrl Pts',(0.701240227960024,-0.360353291538606,
-0.28694340163969));
#57917=CARTESIAN_POINT('Ctrl Pts',(0.788314010461381,0.0123843106225132,
-0.276509439037209));
#57918=CARTESIAN_POINT('Ctrl Pts',(0.689574771586226,0.382202801273034,
-0.266075476434728));
#57919=CARTESIAN_POINT('Ctrl Pts',(0.428296274062381,0.661932524534914,
-0.255641513832248));
#57920=CARTESIAN_POINT('Ctrl Pts',(0.0660643238823166,0.785638478676652,
-0.245207551229767));
#57921=CARTESIAN_POINT('Ctrl Pts',(-0.311739618905992,0.72416215772478,
-0.234773588627286));
#57922=CARTESIAN_POINT('Ctrl Pts',(-0.616063582497875,0.491993812660686,
-0.224339626024806));
#57923=CARTESIAN_POINT('Ctrl Pts',(-0.775175608854643,0.14385828691005,
-0.213905663422325));
#57924=CARTESIAN_POINT('Ctrl Pts',(-0.751571377703367,-0.238186748774525,
-0.203471700819845));
#57925=CARTESIAN_POINT('Ctrl Pts',(-0.550814864235516,-0.5640874344097,
-0.193037738217364));
#57926=CARTESIAN_POINT('Ctrl Pts',(-0.220225801435357,-0.757030349608771,
-0.182603775614884));
#57927=CARTESIAN_POINT('Ctrl Pts',(0.162271947040142,-0.771528308468151,
-0.172169813012403));
#57928=CARTESIAN_POINT('Ctrl Pts',(0.506521864189483,-0.604181181458603,
-0.161735850409922));
#57929=CARTESIAN_POINT('Ctrl Pts',(0.73137747471038,-0.294400431622848,
-0.151301887807442));
#57930=CARTESIAN_POINT('Ctrl Pts',(0.78384510265579,0.0847288019872882,
-0.140867925204961));
#57931=CARTESIAN_POINT('Ctrl Pts',(0.651544586453749,0.443977659175339,
-0.13043396260248));
#57932=CARTESIAN_POINT('Ctrl Pts',(0.460967102820788,0.613562143858204,
-0.12347798753416));
#57933=CARTESIAN_POINT('Ctrl Pts',(0.351283760559796,0.670985139773185,
-0.12));
#57934=CARTESIAN_POINT('Ctrl Pts',(-0.49595640971927,-0.649207665313752,
-1.15727273924394));
#57935=CARTESIAN_POINT('Ctrl Pts',(-0.388302693694886,-0.73144876218464,
-1.15374460067508));
#57936=CARTESIAN_POINT('Ctrl Pts',(-0.131404556932686,-0.841265750467437,
-1.14668832353737));
#57937=CARTESIAN_POINT('Ctrl Pts',(0.286034174319597,-0.801958781222047,
-1.1361039078308));
#57938=CARTESIAN_POINT('Ctrl Pts',(0.634034477218431,-0.568280999134348,
-1.12551949212423));
#57939=CARTESIAN_POINT('Ctrl Pts',(0.828384689818385,-0.196826841568892,
-1.11493507641766));
#57940=CARTESIAN_POINT('Ctrl Pts',(0.821897829369208,0.222332451391623,
-1.10435066071109));
#57941=CARTESIAN_POINT('Ctrl Pts',(0.616183750099592,0.587599496275829,
-1.09376624500452));
#57942=CARTESIAN_POINT('Ctrl Pts',(0.261091496307321,0.810421806269904,
-1.08318182929794));
#57943=CARTESIAN_POINT('Ctrl Pts',(-0.157289815040408,0.836787381022574,
-1.07259741359137));
#57944=CARTESIAN_POINT('Ctrl Pts',(-0.537543482173718,0.66030313786295,
-1.0620129978848));
#57945=CARTESIAN_POINT('Ctrl Pts',(-0.787488063987499,0.323752245535049,
-1.05142858217823));
#57946=CARTESIAN_POINT('Ctrl Pts',(-0.846534688677586,-0.0912809764781274,
-1.04084416647166));
#57947=CARTESIAN_POINT('Ctrl Pts',(-0.700368959446378,-0.484186307032685,
-1.03025975076509));
#57948=CARTESIAN_POINT('Ctrl Pts',(-0.384423873291054,-0.759717979177559,
-1.01967533505852));
#57949=CARTESIAN_POINT('Ctrl Pts',(0.0247111232736737,-0.851083110906004,
-1.00909091935195));
#57950=CARTESIAN_POINT('Ctrl Pts',(0.427855760691938,-0.736133514901143,
-0.998506503645379));
#57951=CARTESIAN_POINT('Ctrl Pts',(0.727282047487867,-0.442734604895684,
-0.987922087938806));
#57952=CARTESIAN_POINT('Ctrl Pts',(0.850404740342968,-0.0420104871635237,
-0.977337672232236));
#57953=CARTESIAN_POINT('Ctrl Pts',(0.767377146099822,0.368897575755565,
-0.966753256525666));
#57954=CARTESIAN_POINT('Ctrl Pts',(0.498326337204488,0.690379581274125,
-0.956168840819094));
#57955=CARTESIAN_POINT('Ctrl Pts',(0.108474086749782,0.844503687104732,
-0.945584425112523));
#57956=CARTESIAN_POINT('Ctrl Pts',(-0.307673836701549,0.793908001690771,
-0.935000009405954));
#57957=CARTESIAN_POINT('Ctrl Pts',(-0.649237214524838,0.550857644208326,
-0.92441559369938));
#57958=CARTESIAN_POINT('Ctrl Pts',(-0.833416191506256,0.174271502818133,
-0.913831177992813));
#57959=CARTESIAN_POINT('Ctrl Pts',(-0.815563145108209,-0.244560547230943,
-0.90324676228624));
#57960=CARTESIAN_POINT('Ctrl Pts',(-0.600005909618339,-0.604107617370173,
-0.892662346579669));
#57961=CARTESIAN_POINT('Ctrl Pts',(-0.238998646675456,-0.817210347352623,
-0.882077930873099));
#57962=CARTESIAN_POINT('Ctrl Pts',(0.179945311812538,-0.832209582792671,
-0.871493515166528));
#57963=CARTESIAN_POINT('Ctrl Pts',(0.555267949047112,-0.645469294154581,
-0.860909099459957));
#57964=CARTESIAN_POINT('Ctrl Pts',(0.795985681346874,-0.302258002417496,
-0.850324683753386));
#57965=CARTESIAN_POINT('Ctrl Pts',(0.843745082180559,0.114224958881187,
-0.839740268046816));
#57966=CARTESIAN_POINT('Ctrl Pts',(0.686968588642089,0.503018153901045,
-0.829155852340245));
#57967=CARTESIAN_POINT('Ctrl Pts',(0.363661068552688,0.769872542797965,
-0.818571436633674));
#57968=CARTESIAN_POINT('Ctrl Pts',(-0.0478031039138072,0.850098799076459,
-0.807987020927103));
#57969=CARTESIAN_POINT('Ctrl Pts',(-0.447679119223231,0.724248928992339,
-0.797402605220533));
#57970=CARTESIAN_POINT('Ctrl Pts',(-0.739031303134287,0.422830743823914,
-0.786818189513961));
#57971=CARTESIAN_POINT('Ctrl Pts',(-0.851231712714971,0.0189123294010497,
-0.776233773807391));
#57972=CARTESIAN_POINT('Ctrl Pts',(-0.757081361438326,-0.389590704583328,
-0.76564935810082));
#57973=CARTESIAN_POINT('Ctrl Pts',(-0.47940364313556,-0.703651370980966,
-0.755064942394249));
#57974=CARTESIAN_POINT('Ctrl Pts',(-0.0855116143916544,-0.847136865411472,
-0.744480526687677));
#57975=CARTESIAN_POINT('Ctrl Pts',(0.32910965461467,-0.785264248628736,
-0.733896110981108));
#57976=CARTESIAN_POINT('Ctrl Pts',(0.663950028923554,-0.533032329251662,
-0.723311695274536));
#57977=CARTESIAN_POINT('Ctrl Pts',(0.837839405292465,-0.151585737700515,
-0.712727279567966));
#57978=CARTESIAN_POINT('Ctrl Pts',(0.808624507964924,0.266607408099483,
-0.702142863861395));
#57979=CARTESIAN_POINT('Ctrl Pts',(0.583387446549701,0.620171099087391,
-0.691558448154824));
#57980=CARTESIAN_POINT('Ctrl Pts',(0.216728911202076,0.823396431850541,
-0.680974032448253));
#57981=CARTESIAN_POINT('Ctrl Pts',(-0.202467816811901,0.82701867457178,
-0.670389616741682));
#57982=CARTESIAN_POINT('Ctrl Pts',(-0.572583445726546,0.630159743727697,
-0.659805201035112));
#57983=CARTESIAN_POINT('Ctrl Pts',(-0.803896645273109,0.28054106411305,
-0.64922078532854));
#57984=CARTESIAN_POINT('Ctrl Pts',(-0.840333782374011,-0.13708478812774,
-0.63863636962197));
#57985=CARTESIAN_POINT('Ctrl Pts',(-0.67306197304253,-0.521479324018831,
-0.628051953915399));
#57986=CARTESIAN_POINT('Ctrl Pts',(-0.342630299990165,-0.779459801698389,
-0.617467538208829));
#57987=CARTESIAN_POINT('Ctrl Pts',(0.0708598658787425,-0.848488057866866,
-0.606883122502257));
#57988=CARTESIAN_POINT('Ctrl Pts',(0.467172585207633,-0.711830654415401,
-0.596298706795688));
#57989=CARTESIAN_POINT('Ctrl Pts',(0.750235977744157,-0.402615303525972,
-0.585714291089115));
#57990=CARTESIAN_POINT('Ctrl Pts',(0.851431422320549,0.00419976430822538,
-0.575129875382545));
#57991=CARTESIAN_POINT('Ctrl Pts',(0.746227693570421,0.409996749113468,
-0.564545459675974));
#57992=CARTESIAN_POINT('Ctrl Pts',(0.460127682361608,0.71640464882605,-0.553961043969404));
#57993=CARTESIAN_POINT('Ctrl Pts',(0.0624861297268915,0.849145799334127,
-0.543376628262832));
#57994=CARTESIAN_POINT('Ctrl Pts',(-0.350302955852823,0.776041844268604,
-0.532792212556262));
#57995=CARTESIAN_POINT('Ctrl Pts',(-0.678173586925882,0.514814229534424,
-0.522207796849691));
#57996=CARTESIAN_POINT('Ctrl Pts',(-0.841645225850066,0.128788270967645,
-0.51162338114312));
#57997=CARTESIAN_POINT('Ctrl Pts',(-0.801090005657138,-0.288457809343555,
-0.501038965436549));
#57998=CARTESIAN_POINT('Ctrl Pts',(-0.56633909266593,-0.635777584579214,
-0.490454549729979));
#57999=CARTESIAN_POINT('Ctrl Pts',(-0.19429947093741,-0.828975765947642,
-0.479870134023407));
#58000=CARTESIAN_POINT('Ctrl Pts',(0.224841125840782,-0.821218346766365,
-0.469285718316837));
#58001=CARTESIAN_POINT('Ctrl Pts',(0.5894770129187,-0.61438583656814,-0.458701302610266));
#58002=CARTESIAN_POINT('Ctrl Pts',(0.811215227944599,-0.258617398652356,
-0.448116886903695));
#58003=CARTESIAN_POINT('Ctrl Pts',(0.836303251248599,0.159843601330512,
-0.437532471197125));
#58004=CARTESIAN_POINT('Ctrl Pts',(0.65865938660081,0.539556222628661,-0.426948055490553));
#58005=CARTESIAN_POINT('Ctrl Pts',(0.321347051500512,0.788472686544896,
-0.416363639783983));
#58006=CARTESIAN_POINT('Ctrl Pts',(-0.0938644121072754,0.84625207655581,
-0.405779224077412));
#58007=CARTESIAN_POINT('Ctrl Pts',(-0.486321797629799,0.698887840846451,
-0.395194808370841));
#58008=CARTESIAN_POINT('Ctrl Pts',(-0.760887812970074,0.382103181111091,
-0.38461039266427));
#58009=CARTESIAN_POINT('Ctrl Pts',(-0.851003722888248,-0.0273087632644477,
-0.374025976957699));
#58010=CARTESIAN_POINT('Ctrl Pts',(-0.734824139984661,-0.430100672232773,
-0.363441561251129));
#58011=CARTESIAN_POINT('Ctrl Pts',(-0.440512659294734,-0.728630017160838,
-0.352857145544558));
#58012=CARTESIAN_POINT('Ctrl Pts',(-0.0394145998886097,-0.850529008473493,
-0.342272729837987));
#58013=CARTESIAN_POINT('Ctrl Pts',(0.37123812340591,-0.766247584504999,
-0.331688314131417));
#58014=CARTESIAN_POINT('Ctrl Pts',(0.691897407156199,-0.496216769731138,
-0.321103898424845));
#58015=CARTESIAN_POINT('Ctrl Pts',(0.844830849187049,-0.105895901792893,
-0.310519482718275));
#58016=CARTESIAN_POINT('Ctrl Pts',(0.792965189320112,0.310095649688973,
-0.299935067011704));
#58017=CARTESIAN_POINT('Ctrl Pts',(0.5488734125492,0.650915573609111,-0.289350651305133));
#58018=CARTESIAN_POINT('Ctrl Pts',(0.17172685017993,0.833944238330878,-0.278766235598562));
#58019=CARTESIAN_POINT('Ctrl Pts',(-0.247048745074766,0.814812873511378,
-0.268181819891991));
#58020=CARTESIAN_POINT('Ctrl Pts',(-0.605936216145875,0.598159196372129,
-0.257597404185421));
#58021=CARTESIAN_POINT('Ctrl Pts',(-0.81793600853748,0.236503161103032,
-0.24701298847885));
#58022=CARTESIAN_POINT('Ctrl Pts',(-0.831656513568511,-0.182484627408247,
-0.236428572772279));
#58023=CARTESIAN_POINT('Ctrl Pts',(-0.643771334910437,-0.557235529878883,
-0.225844157065708));
#58024=CARTESIAN_POINT('Ctrl Pts',(-0.299827217601208,-0.796904554312887,
-0.215259741359137));
#58025=CARTESIAN_POINT('Ctrl Pts',(0.116800205661499,-0.843392505842621,
-0.204675325652566));
#58026=CARTESIAN_POINT('Ctrl Pts',(0.50511183077168,-0.685430019722108,
-0.194090909945995));
#58027=CARTESIAN_POINT('Ctrl Pts',(0.770980560490101,-0.361309503413311,
-0.183506494239425));
#58028=CARTESIAN_POINT('Ctrl Pts',(0.849945784476039,0.0503976618012852,
-0.172922078532854));
#58029=CARTESIAN_POINT('Ctrl Pts',(0.722885284777076,0.449887613677294,
-0.162337662826283));
#58030=CARTESIAN_POINT('Ctrl Pts',(0.420560857927933,0.74031856457724,-0.151753247119713));
#58031=CARTESIAN_POINT('Ctrl Pts',(0.0163382438423926,0.851285203351961,
-0.141168831413141));
#58032=CARTESIAN_POINT('Ctrl Pts',(-0.391950752487257,0.755890089971345,
-0.130584415706571));
#58033=CARTESIAN_POINT('Ctrl Pts',(-0.600629835243716,0.570122859256891,
-0.123528138568857));
#58034=CARTESIAN_POINT('Ctrl Pts',(-0.676565692095429,0.457932546695683,
-0.12));
#58035=CARTESIAN_POINT('Ctrl Pts',(-0.483897209295843,-0.633422154331296,
-1.14693182616263));
#58036=CARTESIAN_POINT('Ctrl Pts',(-0.378861097787549,-0.713663555562057,
-1.14340368759377));
#58037=CARTESIAN_POINT('Ctrl Pts',(-0.128209449746755,-0.820810339275165,
-1.13634741045605));
#58038=CARTESIAN_POINT('Ctrl Pts',(0.279079241651177,-0.782459120597522,
-1.12576299474949));
#58039=CARTESIAN_POINT('Ctrl Pts',(0.618617902926213,-0.554463223355898,
-1.11517857904291));
#58040=CARTESIAN_POINT('Ctrl Pts',(0.808242482143576,-0.192040988851446,
-1.10459416333634));
#58041=CARTESIAN_POINT('Ctrl Pts',(0.801913349972012,0.216926428726283,
-1.09400974762977));
#58042=CARTESIAN_POINT('Ctrl Pts',(0.601201216968675,0.573311990447837,
-1.0834253319232));
#58043=CARTESIAN_POINT('Ctrl Pts',(0.254743045876759,0.79071636684458,-1.07284091621663));
#58044=CARTESIAN_POINT('Ctrl Pts',(-0.153465306742976,0.816440861566848,
-1.06225650051006));
#58045=CARTESIAN_POINT('Ctrl Pts',(-0.524473090379592,0.644247840010839,
-1.05167208480349));
#58046=CARTESIAN_POINT('Ctrl Pts',(-0.768340259445449,0.31588019641958,
-1.04108766909692));
#58047=CARTESIAN_POINT('Ctrl Pts',(-0.825951163036847,-0.0890614757949546,
-1.03050325339035));
#58048=CARTESIAN_POINT('Ctrl Pts',(-0.683339459500826,-0.472413297138347,
-1.01991883768378));
#58049=CARTESIAN_POINT('Ctrl Pts',(-0.375076591060765,-0.741245405385502,
-1.00933442197721));
#58050=CARTESIAN_POINT('Ctrl Pts',(0.0241102712987718,-0.830388990192416,
-0.998750006270636));
#58051=CARTESIAN_POINT('Ctrl Pts',(0.417452430339938,-0.718234398324307,
-0.988165590564064));
#58052=CARTESIAN_POINT('Ctrl Pts',(0.709598154703862,-0.431969494837231,
-0.977581174857494));
#58053=CARTESIAN_POINT('Ctrl Pts',(0.829727114237415,-0.0409890004468223,
-0.966996759150922));
#58054=CARTESIAN_POINT('Ctrl Pts',(0.748718339350227,0.35992781608602,-0.956412343444353));
#58055=CARTESIAN_POINT('Ctrl Pts',(0.486209511897154,0.673592973468133,
-0.94582792773778));
#58056=CARTESIAN_POINT('Ctrl Pts',(0.105836534885891,0.823969545350454,
-0.935243512031211));
#58057=CARTESIAN_POINT('Ctrl Pts',(-0.300192734755657,0.77460409610042,
-0.924659096324639));
#58058=CARTESIAN_POINT('Ctrl Pts',(-0.633450985052105,0.537463518018798,
-0.914074680618068));
#58059=CARTESIAN_POINT('Ctrl Pts',(-0.813151642661748,0.170034084086585,
-0.903490264911498));
#58060=CARTESIAN_POINT('Ctrl Pts',(-0.795732693818375,-0.238614047504506,
-0.892905849204928));
#58061=CARTESIAN_POINT('Ctrl Pts',(-0.585416741341587,-0.589418715901375,
-0.882321433498355));
#58062=CARTESIAN_POINT('Ctrl Pts',(-0.233187384788915,-0.797339844272722,
-0.871737017791786));
#58063=CARTESIAN_POINT('Ctrl Pts',(0.175569934182816,-0.811974372688474,
-0.861152602085214));
#58064=CARTESIAN_POINT('Ctrl Pts',(0.541766586114726,-0.629774681820034,
-0.850568186378644));
#58065=CARTESIAN_POINT('Ctrl Pts',(0.776631256890553,-0.294908586704127,
-0.839983770672073));
#58066=CARTESIAN_POINT('Ctrl Pts',(0.823229385936095,0.111447574325788,
-0.829399354965502));
#58067=CARTESIAN_POINT('Ctrl Pts',(0.670264919261704,0.490787246878494,
-0.818814939258932));
#58068=CARTESIAN_POINT('Ctrl Pts',(0.354818634770339,0.75115306037541,-0.80823052355236));
#58069=CARTESIAN_POINT('Ctrl Pts',(-0.04664076948348,0.829428611945336,
-0.797646107845791));
#58070=CARTESIAN_POINT('Ctrl Pts',(-0.436793783096309,0.706638786608829,
-0.787061692139218));
#58071=CARTESIAN_POINT('Ctrl Pts',(-0.721061726717831,0.412549596962952,
-0.776477276432649));
#58072=CARTESIAN_POINT('Ctrl Pts',(-0.830533978742308,0.0184524753367573,
-0.765892860726077));
#58073=CARTESIAN_POINT('Ctrl Pts',(-0.73867289711463,-0.380117790638465,
-0.755308445019506));
#58074=CARTESIAN_POINT('Ctrl Pts',(-0.467746923909842,-0.686542059064459,
-0.744724029312936));
#58075=CARTESIAN_POINT('Ctrl Pts',(-0.0834323959840052,-0.826538697818775,
-0.734139613606364));
#58076=CARTESIAN_POINT('Ctrl Pts',(0.321107339877919,-0.766170516248253,
-0.723555197899794));
#58077=CARTESIAN_POINT('Ctrl Pts',(0.647806056765878,-0.520071626325673,
-0.712970782193223));
#58078=CARTESIAN_POINT('Ctrl Pts',(0.817467305823513,-0.147899924277319,
-0.702386366486652));
#58079=CARTESIAN_POINT('Ctrl Pts',(0.788962769921528,0.260124838047689,
-0.691801950780082));
#58080=CARTESIAN_POINT('Ctrl Pts',(0.569202356883381,0.60509161340246,-0.681217535073511));
#58081=CARTESIAN_POINT('Ctrl Pts',(0.211459138846042,0.803375513872609,
-0.67063311936694));
#58082=CARTESIAN_POINT('Ctrl Pts',(-0.197544803550293,0.806909681613663,
-0.660048703660368));
#58083=CARTESIAN_POINT('Ctrl Pts',(-0.55866105578292,0.614837383739067,
-0.649464287953799));
#58084=CARTESIAN_POINT('Ctrl Pts',(-0.784349865404783,0.273719696644373,
-0.638879872247227));
#58085=CARTESIAN_POINT('Ctrl Pts',(-0.819901032024116,-0.133751565887562,
-0.628295456540657));
#58086=CARTESIAN_POINT('Ctrl Pts',(-0.656696443590252,-0.508799532888447,
-0.617711040834086));
#58087=CARTESIAN_POINT('Ctrl Pts',(-0.334299230207119,-0.760507204682846,
-0.607126625127515));
#58088=CARTESIAN_POINT('Ctrl Pts',(0.0691369053365199,-0.827857035974253,
-0.596542209420944));
#58089=CARTESIAN_POINT('Ctrl Pts',(0.455813264656584,-0.694522462887051,
-0.585957793714374));
#58090=CARTESIAN_POINT('Ctrl Pts',(0.731993959205465,-0.392825695924154,
-0.575373378007802));
#58091=CARTESIAN_POINT('Ctrl Pts',(0.830728832400647,0.00409764686699242,
-0.564788962301232));
#58092=CARTESIAN_POINT('Ctrl Pts',(0.728083136625646,0.400027661359745,
-0.554204546594661));
#58093=CARTESIAN_POINT('Ctrl Pts',(0.448939658911915,0.698985240436193,
-0.54362013088809));
#58094=CARTESIAN_POINT('Ctrl Pts',(0.0609667769223016,0.828498784430788,
-0.533035715181519));
#58095=CARTESIAN_POINT('Ctrl Pts',(-0.3417853251281,0.757172355028012,-0.522451299474948));
#58096=CARTESIAN_POINT('Ctrl Pts',(-0.661683768372591,0.50229650044952,
-0.511866883768378));
#58097=CARTESIAN_POINT('Ctrl Pts',(-0.821180587698315,0.125656778882152,
-0.501282468061807));
#58098=CARTESIAN_POINT('Ctrl Pts',(-0.781611469346072,-0.281443945890222,
-0.490698052355236));
#58099=CARTESIAN_POINT('Ctrl Pts',(-0.552568534422826,-0.620318626560096,
-0.480113636648666));
#58100=CARTESIAN_POINT('Ctrl Pts',(-0.189575071340425,-0.808819186232532,
-0.469529220942094));
#58101=CARTESIAN_POINT('Ctrl Pts',(0.219374104653422,-0.801250389016498,
-0.458944805235524));
#58102=CARTESIAN_POINT('Ctrl Pts',(0.575143855196607,-0.599447019778407,
-0.448360389528952));
#58103=CARTESIAN_POINT('Ctrl Pts',(0.791490496438746,-0.252329106007648,
-0.437775973822382));
#58104=CARTESIAN_POINT('Ctrl Pts',(0.815968503428164,0.1559569976148,-0.427191558115811));
#58105=CARTESIAN_POINT('Ctrl Pts',(0.642644056627987,0.526436890967903,
-0.416607142409241));
#58106=CARTESIAN_POINT('Ctrl Pts',(0.313533484776543,0.76930094086502,-0.40602272670267));
#58107=CARTESIAN_POINT('Ctrl Pts',(-0.0915820950809284,0.825675422640391,
-0.395438310996099));
#58108=CARTESIAN_POINT('Ctrl Pts',(-0.474496863194093,0.681894354360343,
-0.384853895289528));
#58109=CARTESIAN_POINT('Ctrl Pts',(-0.742386794621422,0.372812326606244,
-0.374269479582957));
#58110=CARTESIAN_POINT('Ctrl Pts',(-0.830311532497563,-0.0266447495667352,
-0.363685063876386));
#58111=CARTESIAN_POINT('Ctrl Pts',(-0.71695686091257,-0.419642756764676,
-0.353100648169815));
#58112=CARTESIAN_POINT('Ctrl Pts',(-0.429801575934607,-0.710913348439002,
-0.342516232463245));
#58113=CARTESIAN_POINT('Ctrl Pts',(-0.0384562322773608,-0.829848360783256,
-0.331931816756673));
#58114=CARTESIAN_POINT('Ctrl Pts',(0.362211453224346,-0.747616243091864,
-0.321347401050103));
#58115=CARTESIAN_POINT('Ctrl Pts',(0.675073893351694,-0.484151238643356,
-0.310762985343532));
#58116=CARTESIAN_POINT('Ctrl Pts',(0.824288752473333,-0.103321038601866,
-0.300178569636962));
#58117=CARTESIAN_POINT('Ctrl Pts',(0.773684208251183,0.302555661261062,
-0.28959415393039));
#58118=CARTESIAN_POINT('Ctrl Pts',(0.535527533033765,0.635088534766474,
-0.27900973822382));
#58119=CARTESIAN_POINT('Ctrl Pts',(0.167551304781544,0.813666850006195,
-0.268425322517249));
#58120=CARTESIAN_POINT('Ctrl Pts',(-0.241041744715806,0.795000665106161,
-0.257840906810678));
#58121=CARTESIAN_POINT('Ctrl Pts',(-0.591202852222921,0.583614931003625,
-0.247256491104108));
#58122=CARTESIAN_POINT('Ctrl Pts',(-0.798047860976137,0.230752577050434,
-0.236672075397536));
#58123=CARTESIAN_POINT('Ctrl Pts',(-0.811434751365161,-0.17804750621577,
-0.226087659690966));
#58124=CARTESIAN_POINT('Ctrl Pts',(-0.628118008524482,-0.543686325137952,
-0.215503243984395));
#58125=CARTESIAN_POINT('Ctrl Pts',(-0.292536906520245,-0.77752778742275,
-0.204918828277824));
#58126=CARTESIAN_POINT('Ctrl Pts',(0.11396020387512,-0.822885382506259,
-0.194334412571253));
#58127=CARTESIAN_POINT('Ctrl Pts',(0.492830015910234,-0.668763760708055,
-0.183749996864683));
#58128=CARTESIAN_POINT('Ctrl Pts',(0.752234136571964,-0.352524248033677,
-0.173165581158112));
#58129=CARTESIAN_POINT('Ctrl Pts',(0.829279317901194,0.0491722405896154,
-0.162581165451541));
#58130=CARTESIAN_POINT('Ctrl Pts',(0.705308299458534,0.438948577917231,
-0.15199674974497));
#58131=CARTESIAN_POINT('Ctrl Pts',(0.410334903435537,0.722317688346055,
-0.1414123340384));
#58132=CARTESIAN_POINT('Ctrl Pts',(0.0159409787739283,0.830586168752267,
-0.130827918331828));
#58133=CARTESIAN_POINT('Ctrl Pts',(-0.38242045388091,0.737510591462181,
-0.120243502625258));
#58134=CARTESIAN_POINT('Ctrl Pts',(-0.58602549618982,0.556260298574094,
-0.113187225487544));
#58135=CARTESIAN_POINT('Ctrl Pts',(-0.660114969570821,0.446797898059648,
-0.109659086918687));
#58136=CARTESIAN_POINT('Ctrl Pts',(-0.471838008872417,-0.61763664334884,
-1.13659091308131));
#58137=CARTESIAN_POINT('Ctrl Pts',(-0.369419501880212,-0.695878348939475,
-1.13306277451246));
#58138=CARTESIAN_POINT('Ctrl Pts',(-0.125014342560822,-0.800354928082892,
-1.12600649737474));
#58139=CARTESIAN_POINT('Ctrl Pts',(0.272124308982756,-0.762959459972999,
-1.11542208166817));
#58140=CARTESIAN_POINT('Ctrl Pts',(0.603201328633994,-0.540645447577447,
-1.1048376659616));
#58141=CARTESIAN_POINT('Ctrl Pts',(0.788100274468769,-0.187255136134001,
-1.09425325025503));
#58142=CARTESIAN_POINT('Ctrl Pts',(0.781928870574815,0.211520406060943,
-1.08366883454846));
#58143=CARTESIAN_POINT('Ctrl Pts',(0.586218683837759,0.559024484619844,
-1.07308441884189));
#58144=CARTESIAN_POINT('Ctrl Pts',(0.248394595446197,0.771010927419258,
-1.06250000313532));
#58145=CARTESIAN_POINT('Ctrl Pts',(-0.149640798445545,0.796094342111123,
-1.05191558742875));
#58146=CARTESIAN_POINT('Ctrl Pts',(-0.511402698585466,0.628192542158727,
-1.04133117172218));
#58147=CARTESIAN_POINT('Ctrl Pts',(-0.749192454903401,0.308008147304111,
-1.0307467560156));
#58148=CARTESIAN_POINT('Ctrl Pts',(-0.805367637396107,-0.0868419751117828,
-1.02016234030903));
#58149=CARTESIAN_POINT('Ctrl Pts',(-0.666309959555275,-0.460640287244008,
-1.00957792460246));
#58150=CARTESIAN_POINT('Ctrl Pts',(-0.365729308830476,-0.722772831593447,
-0.998993508895893));
#58151=CARTESIAN_POINT('Ctrl Pts',(0.0235094193238699,-0.809694869478828,
-0.988409093189323));
#58152=CARTESIAN_POINT('Ctrl Pts',(0.407049099987939,-0.700335281747471,
-0.977824677482751));
#58153=CARTESIAN_POINT('Ctrl Pts',(0.691914261919856,-0.421204384778777,
-0.96724026177618));
#58154=CARTESIAN_POINT('Ctrl Pts',(0.809049488131863,-0.0399675137301213,
-0.95665584606961));
#58155=CARTESIAN_POINT('Ctrl Pts',(0.730059532600632,0.350958056416475,
-0.94607143036304));
#58156=CARTESIAN_POINT('Ctrl Pts',(0.474092686589821,0.65680636566214,-0.935487014656467));
#58157=CARTESIAN_POINT('Ctrl Pts',(0.103198983021999,0.803435403596176,
-0.924902598949898));
#58158=CARTESIAN_POINT('Ctrl Pts',(-0.292711632809765,0.755300190510067,
-0.914318183243327));
#58159=CARTESIAN_POINT('Ctrl Pts',(-0.61766475557937,0.524069391829271,
-0.903733767536755));
#58160=CARTESIAN_POINT('Ctrl Pts',(-0.792887093817242,0.165796665355037,
-0.893149351830184));
#58161=CARTESIAN_POINT('Ctrl Pts',(-0.775902242528539,-0.232667547778068,
-0.882564936123614));
#58162=CARTESIAN_POINT('Ctrl Pts',(-0.570827573064836,-0.574729814432577,
-0.871980520417042));
#58163=CARTESIAN_POINT('Ctrl Pts',(-0.227376122902374,-0.777469341192823,
-0.861396104710473));
#58164=CARTESIAN_POINT('Ctrl Pts',(0.171194556553094,-0.791739162584277,
-0.850811689003901));
#58165=CARTESIAN_POINT('Ctrl Pts',(0.528265223182337,-0.614080069485487,
-0.840227273297331));
#58166=CARTESIAN_POINT('Ctrl Pts',(0.757276832434234,-0.287559170990757,
-0.829642857590759));
#58167=CARTESIAN_POINT('Ctrl Pts',(0.80271368969163,0.108670189770389,-0.819058441884189));
#58168=CARTESIAN_POINT('Ctrl Pts',(0.65356124988132,0.478556339855944,-0.808474026177618));
#58169=CARTESIAN_POINT('Ctrl Pts',(0.345976200987988,0.732433577952855,
-0.797889610471048));
#58170=CARTESIAN_POINT('Ctrl Pts',(-0.0454784350531522,0.808758424814215,
-0.787305194764476));
#58171=CARTESIAN_POINT('Ctrl Pts',(-0.425908446969388,0.689028644225319,
-0.776720779057906));
#58172=CARTESIAN_POINT('Ctrl Pts',(-0.703092150301373,0.402268450101991,
-0.766136363351335));
#58173=CARTESIAN_POINT('Ctrl Pts',(-0.809836244769647,0.0179926212724646,
-0.755551947644764));
#58174=CARTESIAN_POINT('Ctrl Pts',(-0.720264432790935,-0.370644876693602,
-0.744967531938193));
#58175=CARTESIAN_POINT('Ctrl Pts',(-0.456090204684125,-0.669432747147952,
-0.734383116231623));
#58176=CARTESIAN_POINT('Ctrl Pts',(-0.0813531775763558,-0.805940530226078,
-0.723798700525051));
#58177=CARTESIAN_POINT('Ctrl Pts',(0.313105025141168,-0.747076783867769,
-0.713214284818481));
#58178=CARTESIAN_POINT('Ctrl Pts',(0.631662084608203,-0.507110923399684,
-0.702629869111909));
#58179=CARTESIAN_POINT('Ctrl Pts',(0.797095206354558,-0.144214110854122,
-0.69204545340534));
#58180=CARTESIAN_POINT('Ctrl Pts',(0.769301031878133,0.253642267995895,
-0.681461037698768));
#58181=CARTESIAN_POINT('Ctrl Pts',(0.55501726721706,0.59001212771753,-0.670876621992198));
#58182=CARTESIAN_POINT('Ctrl Pts',(0.206189366490007,0.783354595894676,
-0.660292206285626));
#58183=CARTESIAN_POINT('Ctrl Pts',(-0.192621790288684,0.786800688655547,
-0.649707790579056));
#58184=CARTESIAN_POINT('Ctrl Pts',(-0.544738665839294,0.599515023750437,
-0.639123374872485));
#58185=CARTESIAN_POINT('Ctrl Pts',(-0.764803085536455,0.266898329175697,
-0.628538959165915));
#58186=CARTESIAN_POINT('Ctrl Pts',(-0.799468281674222,-0.130418343647384,
-0.617954543459343));
#58187=CARTESIAN_POINT('Ctrl Pts',(-0.640330914137974,-0.496119741758062,
-0.607370127752773));
#58188=CARTESIAN_POINT('Ctrl Pts',(-0.325968160424073,-0.741554607667304,
-0.596785712046202));
#58189=CARTESIAN_POINT('Ctrl Pts',(0.0674139447942975,-0.807226014081639,
-0.586201296339631));
#58190=CARTESIAN_POINT('Ctrl Pts',(0.444453944105535,-0.677214271358701,
-0.57561688063306));
#58191=CARTESIAN_POINT('Ctrl Pts',(0.713751940666774,-0.383036088322335,
-0.565032464926489));
#58192=CARTESIAN_POINT('Ctrl Pts',(0.810026242480741,0.00399552942575872,
-0.554448049219919));
#58193=CARTESIAN_POINT('Ctrl Pts',(0.709938579680872,0.390058573606024,
-0.543863633513348));
#58194=CARTESIAN_POINT('Ctrl Pts',(0.43775163546222,0.681565832046335,-0.533279217806777));
#58195=CARTESIAN_POINT('Ctrl Pts',(0.0594474241177121,0.807851769527448,
-0.522694802100205));
#58196=CARTESIAN_POINT('Ctrl Pts',(-0.333267694403378,0.73830286578742,
-0.512110386393635));
#58197=CARTESIAN_POINT('Ctrl Pts',(-0.645193949819299,0.489778771364616,
-0.501525970687064));
#58198=CARTESIAN_POINT('Ctrl Pts',(-0.800715949546566,0.122525286796658,
-0.490941554980494));
#58199=CARTESIAN_POINT('Ctrl Pts',(-0.762132933035005,-0.274430082436889,
-0.480357139273922));
#58200=CARTESIAN_POINT('Ctrl Pts',(-0.538797976179722,-0.604859668540979,
-0.469772723567353));
#58201=CARTESIAN_POINT('Ctrl Pts',(-0.184850671743438,-0.788662606517423,
-0.459188307860781));
#58202=CARTESIAN_POINT('Ctrl Pts',(0.21390708346606,-0.78128243126663,-0.44860389215421));
#58203=CARTESIAN_POINT('Ctrl Pts',(0.560810697474516,-0.584508202988675,
-0.438019476447639));
#58204=CARTESIAN_POINT('Ctrl Pts',(0.771765764932894,-0.246040813362938,
-0.427435060741069));
#58205=CARTESIAN_POINT('Ctrl Pts',(0.795633755607728,0.152070393899087,
-0.416850645034498));
#58206=CARTESIAN_POINT('Ctrl Pts',(0.626628726655166,0.513317559307146,
-0.406266229327927));
#58207=CARTESIAN_POINT('Ctrl Pts',(0.305719918052573,0.750129195185145,
-0.395681813621356));
#58208=CARTESIAN_POINT('Ctrl Pts',(-0.0892997780545805,0.805098768724972,
-0.385097397914785));
#58209=CARTESIAN_POINT('Ctrl Pts',(-0.462671928758388,0.664900867874235,
-0.374512982208215));
#58210=CARTESIAN_POINT('Ctrl Pts',(-0.723885776272768,0.363521472101399,
-0.363928566501644));
#58211=CARTESIAN_POINT('Ctrl Pts',(-0.80961934210688,-0.0259807358690237,
-0.353344150795073));
#58212=CARTESIAN_POINT('Ctrl Pts',(-0.699089581840477,-0.409184841296579,
-0.342759735088502));
#58213=CARTESIAN_POINT('Ctrl Pts',(-0.419090492574482,-0.693196679717168,
-0.332175319381931));
#58214=CARTESIAN_POINT('Ctrl Pts',(-0.0374978646661122,-0.809167713093017,
-0.321590903675361));
#58215=CARTESIAN_POINT('Ctrl Pts',(0.353184783042783,-0.72898490167873,
-0.31100648796879));
#58216=CARTESIAN_POINT('Ctrl Pts',(0.658250379547188,-0.472085707555573,
-0.300422072262219));
#58217=CARTESIAN_POINT('Ctrl Pts',(0.803746655759619,-0.100746175410839,
-0.289837656555648));
#58218=CARTESIAN_POINT('Ctrl Pts',(0.754403227182254,0.295015672833151,
-0.279253240849077));
#58219=CARTESIAN_POINT('Ctrl Pts',(0.522181653518331,0.619261495923837,
-0.268668825142507));
#58220=CARTESIAN_POINT('Ctrl Pts',(0.163375759383157,0.793389461681513,
-0.258084409435936));
#58221=CARTESIAN_POINT('Ctrl Pts',(-0.235034744356846,0.775188456700942,
-0.247499993729365));
#58222=CARTESIAN_POINT('Ctrl Pts',(-0.576469488299967,0.569070665635123,
-0.236915578022794));
#58223=CARTESIAN_POINT('Ctrl Pts',(-0.778159713414795,0.225001992997835,
-0.226331162316223));
#58224=CARTESIAN_POINT('Ctrl Pts',(-0.79121298916181,-0.173610385023293,
-0.215746746609652));
#58225=CARTESIAN_POINT('Ctrl Pts',(-0.612464682138529,-0.530137120397022,
-0.205162330903082));
#58226=CARTESIAN_POINT('Ctrl Pts',(-0.285246595439281,-0.758151020532611,
-0.194577915196511));
#58227=CARTESIAN_POINT('Ctrl Pts',(0.11112020208874,-0.802378259169899,
-0.18399349948994));
#58228=CARTESIAN_POINT('Ctrl Pts',(0.480548201048789,-0.652097501693999,
-0.173409083783369));
#58229=CARTESIAN_POINT('Ctrl Pts',(0.733487712653825,-0.343738992654043,
-0.162824668076799));
#58230=CARTESIAN_POINT('Ctrl Pts',(0.808612851326351,0.0479468193779454,
-0.152240252370227));
#58231=CARTESIAN_POINT('Ctrl Pts',(0.687731314139993,0.42800954215717,-0.141655836663657));
#58232=CARTESIAN_POINT('Ctrl Pts',(0.400108948943141,0.704316812114868,
-0.131071420957086));
#58233=CARTESIAN_POINT('Ctrl Pts',(0.0155437137054643,0.809887134152576,
-0.120487005250515));
#58234=CARTESIAN_POINT('Ctrl Pts',(-0.372890155274564,0.719131092953015,
-0.109902589543944));
#58235=CARTESIAN_POINT('Ctrl Pts',(-0.571421157135923,0.542397737891296,
-0.10284631240623));
#58236=CARTESIAN_POINT('Ctrl Pts',(-0.643664247046212,0.435663249423613,
-0.0993181738373734));
#58237=CARTESIAN_POINT('Ctrl Pts',(-0.45977880844899,-0.601851132366384,
-1.12625));
#58238=CARTESIAN_POINT('Ctrl Pts',(-0.359977905972875,-0.678093142316892,
-1.12272186143114));
#58239=CARTESIAN_POINT('Ctrl Pts',(-0.12181923537489,-0.77989951689062,
-1.11566558429343));
#58240=CARTESIAN_POINT('Ctrl Pts',(0.265169376314336,-0.743459799348474,
-1.10508116858686));
#58241=CARTESIAN_POINT('Ctrl Pts',(0.587784754341776,-0.526827671798997,
-1.09449675288029));
#58242=CARTESIAN_POINT('Ctrl Pts',(0.767958066793961,-0.182469283416555,
-1.08391233717372));
#58243=CARTESIAN_POINT('Ctrl Pts',(0.761944391177619,0.206114383395603,
-1.07332792146715));
#58244=CARTESIAN_POINT('Ctrl Pts',(0.571236150706841,0.544736978791852,
-1.06274350576058));
#58245=CARTESIAN_POINT('Ctrl Pts',(0.242046145015635,0.751305487993935,
-1.052159090054));
#58246=CARTESIAN_POINT('Ctrl Pts',(-0.145816290148113,0.775747822655397,
-1.04157467434743));
#58247=CARTESIAN_POINT('Ctrl Pts',(-0.49833230679134,0.612137244306616,
-1.03099025864086));
#58248=CARTESIAN_POINT('Ctrl Pts',(-0.730044650361351,0.300136098188643,
-1.02040584293429));
#58249=CARTESIAN_POINT('Ctrl Pts',(-0.784784111755368,-0.0846224744286107,
-1.00982142722772));
#58250=CARTESIAN_POINT('Ctrl Pts',(-0.649280459609723,-0.44886727734967,
-0.999237011521151));
#58251=CARTESIAN_POINT('Ctrl Pts',(-0.356382026600188,-0.704300257801391,
-0.988652595814579));
#58252=CARTESIAN_POINT('Ctrl Pts',(0.0229085673489686,-0.789000748765239,
-0.978068180108009));
#58253=CARTESIAN_POINT('Ctrl Pts',(0.396645769635938,-0.682436165170636,
-0.967483764401438));
#58254=CARTESIAN_POINT('Ctrl Pts',(0.674230369135851,-0.410439274720323,
-0.956899348694867));
#58255=CARTESIAN_POINT('Ctrl Pts',(0.788371862026309,-0.0389460270134203,
-0.946314932988296));
#58256=CARTESIAN_POINT('Ctrl Pts',(0.711400725851038,0.34198829674693,-0.935730517281726));
#58257=CARTESIAN_POINT('Ctrl Pts',(0.461975861282486,0.640019757856148,
-0.925146101575154));
#58258=CARTESIAN_POINT('Ctrl Pts',(0.100561431158108,0.782901261841898,
-0.914561685868584));
#58259=CARTESIAN_POINT('Ctrl Pts',(-0.285230530863874,0.735996284919716,
-0.903977270162013));
#58260=CARTESIAN_POINT('Ctrl Pts',(-0.601878526106636,0.510675265639743,
-0.893392854455441));
#58261=CARTESIAN_POINT('Ctrl Pts',(-0.772622544972735,0.161559246623488,
-0.882808438748872));
#58262=CARTESIAN_POINT('Ctrl Pts',(-0.756071791238703,-0.226721048051631,
-0.8722240230423));
#58263=CARTESIAN_POINT('Ctrl Pts',(-0.556238404788085,-0.56004091296378,
-0.86163960733573));
#58264=CARTESIAN_POINT('Ctrl Pts',(-0.221564861015834,-0.757598838112922,
-0.851055191629159));
#58265=CARTESIAN_POINT('Ctrl Pts',(0.166819178923372,-0.77150395248008,
-0.840470775922587));
#58266=CARTESIAN_POINT('Ctrl Pts',(0.514763860249949,-0.598385457150939,
-0.829886360216018));
#58267=CARTESIAN_POINT('Ctrl Pts',(0.737922407977915,-0.280209755277388,
-0.819301944509446));
#58268=CARTESIAN_POINT('Ctrl Pts',(0.782197993447165,0.10589280521499,-0.808717528802876));
#58269=CARTESIAN_POINT('Ctrl Pts',(0.636857580500936,0.466325432833393,
-0.798133113096305));
#58270=CARTESIAN_POINT('Ctrl Pts',(0.337133767205639,0.7137140955303,-0.787548697389734));
#58271=CARTESIAN_POINT('Ctrl Pts',(-0.0443161006228249,0.788088237683092,
-0.776964281683163));
#58272=CARTESIAN_POINT('Ctrl Pts',(-0.415023110842465,0.67141850184181,
-0.766379865976593));
#58273=CARTESIAN_POINT('Ctrl Pts',(-0.685122573884916,0.391987303241029,
-0.755795450270022));
#58274=CARTESIAN_POINT('Ctrl Pts',(-0.789138510796985,0.017532767208172,
-0.745211034563451));
#58275=CARTESIAN_POINT('Ctrl Pts',(-0.70185596846724,-0.361171962748739,
-0.73462661885688));
#58276=CARTESIAN_POINT('Ctrl Pts',(-0.444433485458407,-0.652323435231446,
-0.724042203150309));
#58277=CARTESIAN_POINT('Ctrl Pts',(-0.0792739591687064,-0.78534236263338,
-0.713457787443738));
#58278=CARTESIAN_POINT('Ctrl Pts',(0.305102710404417,-0.727983051487286,
-0.702873371737167));
#58279=CARTESIAN_POINT('Ctrl Pts',(0.615518112450528,-0.494150220473694,
-0.692288956030597));
#58280=CARTESIAN_POINT('Ctrl Pts',(0.776723106885605,-0.140528297430926,
-0.681704540324026));
#58281=CARTESIAN_POINT('Ctrl Pts',(0.749639293834737,0.2471596979441,-0.671120124617455));
#58282=CARTESIAN_POINT('Ctrl Pts',(0.540832177550741,0.5749326420326,-0.660535708910885));
#58283=CARTESIAN_POINT('Ctrl Pts',(0.200919594133972,0.763333677916743,
-0.649951293204313));
#58284=CARTESIAN_POINT('Ctrl Pts',(-0.187698777027075,0.76669169569743,
-0.639366877497742));
#58285=CARTESIAN_POINT('Ctrl Pts',(-0.530816275895669,0.584192663761806,
-0.628782461791172));
#58286=CARTESIAN_POINT('Ctrl Pts',(-0.74525630566813,0.26007696170702,-0.618198046084601));
#58287=CARTESIAN_POINT('Ctrl Pts',(-0.779035531324326,-0.127085121407205,
-0.60761363037803));
#58288=CARTESIAN_POINT('Ctrl Pts',(-0.623965384685697,-0.483439950627679,
-0.59702921467146));
#58289=CARTESIAN_POINT('Ctrl Pts',(-0.317637090641027,-0.72260201065176,
-0.586444798964888));
#58290=CARTESIAN_POINT('Ctrl Pts',(0.0656909842520751,-0.786594992189027,
-0.575860383258318));
#58291=CARTESIAN_POINT('Ctrl Pts',(0.433094623554485,-0.65990607983035,
-0.565275967551747));
#58292=CARTESIAN_POINT('Ctrl Pts',(0.695509922128082,-0.373246480720517,
-0.554691551845176));
#58293=CARTESIAN_POINT('Ctrl Pts',(0.789323652560837,0.00389341198452537,
-0.544107136138605));
#58294=CARTESIAN_POINT('Ctrl Pts',(0.691794022736099,0.380089485852302,
-0.533522720432034));
#58295=CARTESIAN_POINT('Ctrl Pts',(0.426563612012526,0.664146423656478,
-0.522938304725464));
#58296=CARTESIAN_POINT('Ctrl Pts',(0.0579280713131231,0.787204754624109,
-0.512353889018892));
#58297=CARTESIAN_POINT('Ctrl Pts',(-0.324750063678657,0.719433376546828,
-0.501769473312322));
#58298=CARTESIAN_POINT('Ctrl Pts',(-0.628704131266007,0.477261042279711,
-0.491185057605751));
#58299=CARTESIAN_POINT('Ctrl Pts',(-0.780251311394817,0.119393794711166,
-0.480600641899181));
#58300=CARTESIAN_POINT('Ctrl Pts',(-0.742654396723938,-0.267416218983557,
-0.470016226192609));
#58301=CARTESIAN_POINT('Ctrl Pts',(-0.525027417936618,-0.589400710521861,
-0.45943181048604));
#58302=CARTESIAN_POINT('Ctrl Pts',(-0.180126272146453,-0.768506026802316,
-0.448847394779467));
#58303=CARTESIAN_POINT('Ctrl Pts',(0.2084400622787,-0.761314473516762,-0.438262979072897));
#58304=CARTESIAN_POINT('Ctrl Pts',(0.546477539752423,-0.569569386198943,
-0.427678563366326));
#58305=CARTESIAN_POINT('Ctrl Pts',(0.752041033427042,-0.239752520718229,
-0.417094147659756));
#58306=CARTESIAN_POINT('Ctrl Pts',(0.775299007787293,0.148183790183373,
-0.406509731953185));
#58307=CARTESIAN_POINT('Ctrl Pts',(0.610613396682344,0.500198227646389,
-0.395925316246614));
#58308=CARTESIAN_POINT('Ctrl Pts',(0.297906351328603,0.730957449505269,
-0.385340900540043));
#58309=CARTESIAN_POINT('Ctrl Pts',(-0.0870174610282331,0.784522114809553,
-0.374756484833472));
#58310=CARTESIAN_POINT('Ctrl Pts',(-0.450846994322682,0.647907381388128,
-0.364172069126901));
#58311=CARTESIAN_POINT('Ctrl Pts',(-0.705384757924115,0.354230617596552,
-0.353587653420331));
#58312=CARTESIAN_POINT('Ctrl Pts',(-0.788927151716196,-0.0253167221713116,
-0.34300323771376));
#58313=CARTESIAN_POINT('Ctrl Pts',(-0.681222302768386,-0.398726925828482,
-0.332418822007189));
#58314=CARTESIAN_POINT('Ctrl Pts',(-0.408379409214356,-0.675480010995333,
-0.321834406300618));
#58315=CARTESIAN_POINT('Ctrl Pts',(-0.0365394970548637,-0.78848706540278,
-0.311249990594048));
#58316=CARTESIAN_POINT('Ctrl Pts',(0.34415811286122,-0.710353560265595,
-0.300665574887476));
#58317=CARTESIAN_POINT('Ctrl Pts',(0.641426865742682,-0.46002017646779,
-0.290081159180906));
#58318=CARTESIAN_POINT('Ctrl Pts',(0.783204559045905,-0.0981713122198112,
-0.279496743474335));
#58319=CARTESIAN_POINT('Ctrl Pts',(0.735122246113324,0.28747568440524,-0.268912327767764));
#58320=CARTESIAN_POINT('Ctrl Pts',(0.508835774002897,0.603434457081201,
-0.258327912061193));
#58321=CARTESIAN_POINT('Ctrl Pts',(0.15920021398477,0.773112073356828,-0.247743496354623));
#58322=CARTESIAN_POINT('Ctrl Pts',(-0.229027743997885,0.755376248295727,
-0.237159080648052));
#58323=CARTESIAN_POINT('Ctrl Pts',(-0.561736124377014,0.554526400266618,
-0.226574664941481));
#58324=CARTESIAN_POINT('Ctrl Pts',(-0.758271565853453,0.219251408945238,
-0.21599024923491));
#58325=CARTESIAN_POINT('Ctrl Pts',(-0.77099122695846,-0.169173263830817,
-0.205405833528339));
#58326=CARTESIAN_POINT('Ctrl Pts',(-0.596811355752575,-0.516587915656091,
-0.194821417821768));
#58327=CARTESIAN_POINT('Ctrl Pts',(-0.277956284358317,-0.738774253642473,
-0.184237002115198));
#58328=CARTESIAN_POINT('Ctrl Pts',(0.10828020030236,-0.781871135833539,
-0.173652586408627));
#58329=CARTESIAN_POINT('Ctrl Pts',(0.468266386187344,-0.635431242679944,
-0.163068170702056));
#58330=CARTESIAN_POINT('Ctrl Pts',(0.714741288735686,-0.33495373727441,
-0.152483754995485));
#58331=CARTESIAN_POINT('Ctrl Pts',(0.787946384751507,0.0467213981662761,
-0.141899339288914));
#58332=CARTESIAN_POINT('Ctrl Pts',(0.670154328821452,0.417070506397107,
-0.131314923582344));
#58333=CARTESIAN_POINT('Ctrl Pts',(0.389882994450745,0.686315935883682,
-0.120730507875773));
#58334=CARTESIAN_POINT('Ctrl Pts',(0.0151464486370003,0.789188099552884,
-0.110146092169202));
#58335=CARTESIAN_POINT('Ctrl Pts',(-0.363359856668217,0.70075159444385,
-0.0995616764626311));
#58336=CARTESIAN_POINT('Ctrl Pts',(-0.556816818082027,0.528535177208499,
-0.0925053993249171));
#58337=CARTESIAN_POINT('Ctrl Pts',(-0.627213524521604,0.424528600787578,
-0.0889772607560602));
#58338=CARTESIAN_POINT('',(-0.676565692095432,0.457932546695678,-0.12));
#58339=CARTESIAN_POINT('Ctrl Pts',(0.351315334519652,0.671030718912572,
-0.12));
#58340=CARTESIAN_POINT('Ctrl Pts',(0.320499669985717,0.689321131271763,
-0.12));
#58341=CARTESIAN_POINT('Ctrl Pts',(0.288470314380493,0.705335580148948,
-0.12));
#58342=CARTESIAN_POINT('Ctrl Pts',(0.255512129576956,0.71904543011569,-0.12));
#58343=CARTESIAN_POINT('Ctrl Pts',(0.222147796814793,0.732924228330349,
-0.12));
#58344=CARTESIAN_POINT('Ctrl Pts',(0.187830516461056,0.744441808855746,
-0.12));
#58345=CARTESIAN_POINT('Ctrl Pts',(0.152824268659072,0.753525280825666,
-0.12));
#58346=CARTESIAN_POINT('Ctrl Pts',(0.126989719984155,0.760228866998956,
-0.12));
#58347=CARTESIAN_POINT('Ctrl Pts',(0.100779187651715,0.765605880524341,
-0.12));
#58348=CARTESIAN_POINT('Ctrl Pts',(0.0742933277386271,0.769609591773371,
-0.12));
#58349=CARTESIAN_POINT('Ctrl Pts',(0.0666757152808372,0.770761101325565,
-0.12));
#58350=CARTESIAN_POINT('Ctrl Pts',(0.05904330606438,0.771797653690265,-0.12));
#58351=CARTESIAN_POINT('Ctrl Pts',(0.0514033585107013,0.772718183814432,
-0.12));
#58352=CARTESIAN_POINT('Ctrl Pts',(0.0392486607748846,0.774182691958939,
-0.12));
#58353=CARTESIAN_POINT('Ctrl Pts',(0.0270711318452966,0.77535414067244,
-0.12));
#58354=CARTESIAN_POINT('Ctrl Pts',(0.0148810082990253,0.776230637396705,
-0.12));
#58355=CARTESIAN_POINT('Ctrl Pts',(-0.0215690645836386,0.77885147789595,
-0.12));
#58356=CARTESIAN_POINT('Ctrl Pts',(-0.0581308241831653,0.778839173851118,
-0.12));
#58357=CARTESIAN_POINT('Ctrl Pts',(-0.0945366085253862,0.77628931721492,
-0.12));
#58358=CARTESIAN_POINT('Ctrl Pts',(-0.121214846926866,0.774420776694254,
-0.12));
#58359=CARTESIAN_POINT('Ctrl Pts',(-0.147809835066177,0.771188449071339,
-0.12));
#58360=CARTESIAN_POINT('Ctrl Pts',(-0.174217694473098,0.766612275855449,
-0.12));
#58361=CARTESIAN_POINT('Ctrl Pts',(-0.190197279887772,0.76384320057188,
-0.12));
#58362=CARTESIAN_POINT('Ctrl Pts',(-0.206108346384988,0.760581783987262,
-0.12));
#58363=CARTESIAN_POINT('Ctrl Pts',(-0.221927418748357,0.75682985953972,
-0.12));
#58364=CARTESIAN_POINT('Ctrl Pts',(-0.229467360157552,0.755041556796273,
-0.12));
#58365=CARTESIAN_POINT('Ctrl Pts',(-0.236985877665914,0.753141777077181,
-0.12));
#58366=CARTESIAN_POINT('Ctrl Pts',(-0.244467321365349,0.751134526253216,
-0.12));
#58367=CARTESIAN_POINT('Ctrl Pts',(-0.28053587885935,0.741457431208775,
-0.12));
#58368=CARTESIAN_POINT('Ctrl Pts',(-0.315822129989096,0.729268499602105,
-0.12));
#58369=CARTESIAN_POINT('Ctrl Pts',(-0.350052129478668,0.714644278113597,
-0.12));
#58370=CARTESIAN_POINT('Ctrl Pts',(-0.355634194410513,0.712259429876851,
-0.12));
#58371=CARTESIAN_POINT('Ctrl Pts',(-0.361188160013049,0.709809706700498,
-0.12));
#58372=CARTESIAN_POINT('Ctrl Pts',(-0.366712818974203,0.707295310693252,
-0.12));
#58373=CARTESIAN_POINT('Ctrl Pts',(-0.397138122868592,0.693448073575234,
-0.12));
#58374=CARTESIAN_POINT('Ctrl Pts',(-0.426675742611679,0.677641907045331,
-0.12));
#58375=CARTESIAN_POINT('Ctrl Pts',(-0.455180005223254,0.660007879054353,
-0.12));
#58376=CARTESIAN_POINT('Ctrl Pts',(-0.46186601449095,0.655871610869445,
-0.12));
#58377=CARTESIAN_POINT('Ctrl Pts',(-0.468495101204548,0.651634643117698,
-0.12));
#58378=CARTESIAN_POINT('Ctrl Pts',(-0.47506524617052,0.647298434033082,
-0.12));
#58379=CARTESIAN_POINT('Ctrl Pts',(-0.481997163210447,0.642723460147725,
-0.12));
#58380=CARTESIAN_POINT('Ctrl Pts',(-0.488856348608865,0.638042668269532,
-0.12));
#58381=CARTESIAN_POINT('Ctrl Pts',(-0.49563768528437,0.633260662340094,
-0.12));
#58382=CARTESIAN_POINT('Ctrl Pts',(-0.526421712148936,0.611552641334433,
-0.12));
#58383=CARTESIAN_POINT('Ctrl Pts',(-0.55562415886581,0.587748863931158,
-0.12));
#58384=CARTESIAN_POINT('Ctrl Pts',(-0.583051806458648,0.562054023958938,
-0.12));
#58385=CARTESIAN_POINT('Ctrl Pts',(-0.610463295427848,0.536374321750432,
-0.12));
#58386=CARTESIAN_POINT('Ctrl Pts',(-0.636103059525297,0.508805062795953,
-0.12));
#58387=CARTESIAN_POINT('Ctrl Pts',(-0.659749387735623,0.479508356571552,
-0.12));
#58388=CARTESIAN_POINT('Ctrl Pts',(-0.665472951291048,0.472417126231326,
-0.12));
#58389=CARTESIAN_POINT('Ctrl Pts',(-0.67107955278444,0.465224522951303,
-0.12));
#58390=CARTESIAN_POINT('Ctrl Pts',(-0.676565692095429,0.457932546695683,
-0.12));
#58391=CARTESIAN_POINT('Ctrl Pts',(0.589349009255739,-0.565869316348666,
-1.12625));
#58392=CARTESIAN_POINT('Ctrl Pts',(0.595826955511013,-0.559130415243387,
-1.12600649737474));
#58393=CARTESIAN_POINT('Ctrl Pts',(0.694346705276111,-0.453008535243734,
-1.12223485618063));
#58394=CARTESIAN_POINT('Ctrl Pts',(0.828384689818385,-0.196826841568892,
-1.11493507641766));
#58395=CARTESIAN_POINT('Ctrl Pts',(0.821897829369208,0.222332451391623,
-1.10435066071109));
#58396=CARTESIAN_POINT('Ctrl Pts',(0.616183750099592,0.587599496275829,
-1.09376624500452));
#58397=CARTESIAN_POINT('Ctrl Pts',(0.261091496307321,0.810421806269904,
-1.08318182929794));
#58398=CARTESIAN_POINT('Ctrl Pts',(-0.157289815040408,0.836787381022574,
-1.07259741359137));
#58399=CARTESIAN_POINT('Ctrl Pts',(-0.537543482173718,0.66030313786295,
-1.0620129978848));
#58400=CARTESIAN_POINT('Ctrl Pts',(-0.787488063987499,0.323752245535049,
-1.05142858217823));
#58401=CARTESIAN_POINT('Ctrl Pts',(-0.846534688677586,-0.0912809764781274,
-1.04084416647166));
#58402=CARTESIAN_POINT('Ctrl Pts',(-0.700368959446378,-0.484186307032685,
-1.03025975076509));
#58403=CARTESIAN_POINT('Ctrl Pts',(-0.384423873291054,-0.759717979177559,
-1.01967533505852));
#58404=CARTESIAN_POINT('Ctrl Pts',(0.0247111232736737,-0.851083110906004,
-1.00909091935195));
#58405=CARTESIAN_POINT('Ctrl Pts',(0.427855760691938,-0.736133514901143,
-0.998506503645379));
#58406=CARTESIAN_POINT('Ctrl Pts',(0.727282047487867,-0.442734604895684,
-0.987922087938806));
#58407=CARTESIAN_POINT('Ctrl Pts',(0.850404740342968,-0.0420104871635237,
-0.977337672232236));
#58408=CARTESIAN_POINT('Ctrl Pts',(0.767377146099822,0.368897575755565,
-0.966753256525666));
#58409=CARTESIAN_POINT('Ctrl Pts',(0.498326337204488,0.690379581274125,
-0.956168840819094));
#58410=CARTESIAN_POINT('Ctrl Pts',(0.108474086749782,0.844503687104732,
-0.945584425112523));
#58411=CARTESIAN_POINT('Ctrl Pts',(-0.307673836701549,0.793908001690771,
-0.935000009405954));
#58412=CARTESIAN_POINT('Ctrl Pts',(-0.649237214524838,0.550857644208326,
-0.92441559369938));
#58413=CARTESIAN_POINT('Ctrl Pts',(-0.833416191506256,0.174271502818133,
-0.913831177992813));
#58414=CARTESIAN_POINT('Ctrl Pts',(-0.815563145108209,-0.244560547230943,
-0.90324676228624));
#58415=CARTESIAN_POINT('Ctrl Pts',(-0.600005909618339,-0.604107617370173,
-0.892662346579669));
#58416=CARTESIAN_POINT('Ctrl Pts',(-0.238998646675456,-0.817210347352623,
-0.882077930873099));
#58417=CARTESIAN_POINT('Ctrl Pts',(0.179945311812538,-0.832209582792671,
-0.871493515166528));
#58418=CARTESIAN_POINT('Ctrl Pts',(0.555267949047112,-0.645469294154581,
-0.860909099459957));
#58419=CARTESIAN_POINT('Ctrl Pts',(0.795985681346874,-0.302258002417496,
-0.850324683753386));
#58420=CARTESIAN_POINT('Ctrl Pts',(0.843745082180559,0.114224958881187,
-0.839740268046816));
#58421=CARTESIAN_POINT('Ctrl Pts',(0.686968588642089,0.503018153901045,
-0.829155852340245));
#58422=CARTESIAN_POINT('Ctrl Pts',(0.363661068552688,0.769872542797965,
-0.818571436633674));
#58423=CARTESIAN_POINT('Ctrl Pts',(-0.0478031039138072,0.850098799076459,
-0.807987020927103));
#58424=CARTESIAN_POINT('Ctrl Pts',(-0.447679119223231,0.724248928992339,
-0.797402605220533));
#58425=CARTESIAN_POINT('Ctrl Pts',(-0.739031303134287,0.422830743823914,
-0.786818189513961));
#58426=CARTESIAN_POINT('Ctrl Pts',(-0.851231712714971,0.0189123294010497,
-0.776233773807391));
#58427=CARTESIAN_POINT('Ctrl Pts',(-0.757081361438326,-0.389590704583328,
-0.76564935810082));
#58428=CARTESIAN_POINT('Ctrl Pts',(-0.47940364313556,-0.703651370980966,
-0.755064942394249));
#58429=CARTESIAN_POINT('Ctrl Pts',(-0.0855116143916544,-0.847136865411472,
-0.744480526687677));
#58430=CARTESIAN_POINT('Ctrl Pts',(0.32910965461467,-0.785264248628736,
-0.733896110981108));
#58431=CARTESIAN_POINT('Ctrl Pts',(0.663950028923554,-0.533032329251662,
-0.723311695274536));
#58432=CARTESIAN_POINT('Ctrl Pts',(0.837839405292465,-0.151585737700515,
-0.712727279567966));
#58433=CARTESIAN_POINT('Ctrl Pts',(0.808624507964924,0.266607408099483,
-0.702142863861395));
#58434=CARTESIAN_POINT('Ctrl Pts',(0.583387446549701,0.620171099087391,
-0.691558448154824));
#58435=CARTESIAN_POINT('Ctrl Pts',(0.216728911202076,0.823396431850541,
-0.680974032448253));
#58436=CARTESIAN_POINT('Ctrl Pts',(-0.202467816811901,0.82701867457178,
-0.670389616741682));
#58437=CARTESIAN_POINT('Ctrl Pts',(-0.572583445726546,0.630159743727697,
-0.659805201035112));
#58438=CARTESIAN_POINT('Ctrl Pts',(-0.803896645273109,0.28054106411305,
-0.64922078532854));
#58439=CARTESIAN_POINT('Ctrl Pts',(-0.840333782374011,-0.13708478812774,
-0.63863636962197));
#58440=CARTESIAN_POINT('Ctrl Pts',(-0.67306197304253,-0.521479324018831,
-0.628051953915399));
#58441=CARTESIAN_POINT('Ctrl Pts',(-0.342630299990165,-0.779459801698389,
-0.617467538208829));
#58442=CARTESIAN_POINT('Ctrl Pts',(0.0708598658787425,-0.848488057866866,
-0.606883122502257));
#58443=CARTESIAN_POINT('Ctrl Pts',(0.467172585207633,-0.711830654415401,
-0.596298706795688));
#58444=CARTESIAN_POINT('Ctrl Pts',(0.750235977744157,-0.402615303525972,
-0.585714291089115));
#58445=CARTESIAN_POINT('Ctrl Pts',(0.851431422320549,0.00419976430822538,
-0.575129875382545));
#58446=CARTESIAN_POINT('Ctrl Pts',(0.746227693570421,0.409996749113468,
-0.564545459675974));
#58447=CARTESIAN_POINT('Ctrl Pts',(0.460127682361608,0.71640464882605,-0.553961043969404));
#58448=CARTESIAN_POINT('Ctrl Pts',(0.0624861297268915,0.849145799334127,
-0.543376628262832));
#58449=CARTESIAN_POINT('Ctrl Pts',(-0.350302955852823,0.776041844268604,
-0.532792212556262));
#58450=CARTESIAN_POINT('Ctrl Pts',(-0.678173586925882,0.514814229534424,
-0.522207796849691));
#58451=CARTESIAN_POINT('Ctrl Pts',(-0.841645225850066,0.128788270967645,
-0.51162338114312));
#58452=CARTESIAN_POINT('Ctrl Pts',(-0.801090005657138,-0.288457809343555,
-0.501038965436549));
#58453=CARTESIAN_POINT('Ctrl Pts',(-0.56633909266593,-0.635777584579214,
-0.490454549729979));
#58454=CARTESIAN_POINT('Ctrl Pts',(-0.19429947093741,-0.828975765947642,
-0.479870134023407));
#58455=CARTESIAN_POINT('Ctrl Pts',(0.224841125840782,-0.821218346766365,
-0.469285718316837));
#58456=CARTESIAN_POINT('Ctrl Pts',(0.5894770129187,-0.61438583656814,-0.458701302610266));
#58457=CARTESIAN_POINT('Ctrl Pts',(0.811215227944599,-0.258617398652356,
-0.448116886903695));
#58458=CARTESIAN_POINT('Ctrl Pts',(0.836303251248599,0.159843601330512,
-0.437532471197125));
#58459=CARTESIAN_POINT('Ctrl Pts',(0.65865938660081,0.539556222628661,-0.426948055490553));
#58460=CARTESIAN_POINT('Ctrl Pts',(0.321347051500512,0.788472686544896,
-0.416363639783983));
#58461=CARTESIAN_POINT('Ctrl Pts',(-0.0938644121072754,0.84625207655581,
-0.405779224077412));
#58462=CARTESIAN_POINT('Ctrl Pts',(-0.486321797629799,0.698887840846451,
-0.395194808370841));
#58463=CARTESIAN_POINT('Ctrl Pts',(-0.760887812970074,0.382103181111091,
-0.38461039266427));
#58464=CARTESIAN_POINT('Ctrl Pts',(-0.851003722888248,-0.0273087632644477,
-0.374025976957699));
#58465=CARTESIAN_POINT('Ctrl Pts',(-0.734824139984661,-0.430100672232773,
-0.363441561251129));
#58466=CARTESIAN_POINT('Ctrl Pts',(-0.440512659294734,-0.728630017160838,
-0.352857145544558));
#58467=CARTESIAN_POINT('Ctrl Pts',(-0.0394145998886097,-0.850529008473493,
-0.342272729837987));
#58468=CARTESIAN_POINT('Ctrl Pts',(0.37123812340591,-0.766247584504999,
-0.331688314131417));
#58469=CARTESIAN_POINT('Ctrl Pts',(0.691897407156199,-0.496216769731138,
-0.321103898424845));
#58470=CARTESIAN_POINT('Ctrl Pts',(0.844830849187049,-0.105895901792893,
-0.310519482718275));
#58471=CARTESIAN_POINT('Ctrl Pts',(0.792965189320112,0.310095649688973,
-0.299935067011704));
#58472=CARTESIAN_POINT('Ctrl Pts',(0.5488734125492,0.650915573609111,-0.289350651305133));
#58473=CARTESIAN_POINT('Ctrl Pts',(0.17172685017993,0.833944238330878,-0.278766235598562));
#58474=CARTESIAN_POINT('Ctrl Pts',(-0.247048745074766,0.814812873511378,
-0.268181819891991));
#58475=CARTESIAN_POINT('Ctrl Pts',(-0.605936216145875,0.598159196372129,
-0.257597404185421));
#58476=CARTESIAN_POINT('Ctrl Pts',(-0.81793600853748,0.236503161103032,
-0.24701298847885));
#58477=CARTESIAN_POINT('Ctrl Pts',(-0.831656513568511,-0.182484627408247,
-0.236428572772279));
#58478=CARTESIAN_POINT('Ctrl Pts',(-0.643771334910437,-0.557235529878883,
-0.225844157065708));
#58479=CARTESIAN_POINT('Ctrl Pts',(-0.299827217601208,-0.796904554312887,
-0.215259741359137));
#58480=CARTESIAN_POINT('Ctrl Pts',(0.116800205661499,-0.843392505842621,
-0.204675325652566));
#58481=CARTESIAN_POINT('Ctrl Pts',(0.50511183077168,-0.685430019722108,
-0.194090909945995));
#58482=CARTESIAN_POINT('Ctrl Pts',(0.770980560490101,-0.361309503413311,
-0.183506494239425));
#58483=CARTESIAN_POINT('Ctrl Pts',(0.849945784476039,0.0503976618012852,
-0.172922078532854));
#58484=CARTESIAN_POINT('Ctrl Pts',(0.722885284777076,0.449887613677294,
-0.162337662826283));
#58485=CARTESIAN_POINT('Ctrl Pts',(0.420560857927933,0.74031856457724,-0.151753247119713));
#58486=CARTESIAN_POINT('Ctrl Pts',(0.0163382438423926,0.851285203351961,
-0.141168831413141));
#58487=CARTESIAN_POINT('Ctrl Pts',(-0.391950752487257,0.755890089971345,
-0.130584415706571));
#58488=CARTESIAN_POINT('Ctrl Pts',(-0.600629835243716,0.570122859256891,
-0.123528138568857));
#58489=CARTESIAN_POINT('Ctrl Pts',(-0.676565692095429,0.457932546695683,
-0.12));
#58490=CARTESIAN_POINT('Ctrl Pts',(0.589301091561365,-0.565833523687263,
-1.12625));
#58491=CARTESIAN_POINT('Ctrl Pts',(0.681795706363583,-0.469502756447991,
-1.12277201246584));
#58492=CARTESIAN_POINT('Ctrl Pts',(0.818575647567586,-0.230726286157603,
-1.11581603739752));
#58493=CARTESIAN_POINT('Ctrl Pts',(0.830732477917423,0.18205408312639,-1.10538207479504));
#58494=CARTESIAN_POINT('Ctrl Pts',(0.647100797261757,0.551826151980974,
-1.09494811219256));
#58495=CARTESIAN_POINT('Ctrl Pts',(0.310930583933843,0.791574909217227,
-1.08451414959008));
#58496=CARTESIAN_POINT('Ctrl Pts',(-0.0985234799625261,0.844718114599206,
-1.0740801869876));
#58497=CARTESIAN_POINT('Ctrl Pts',(-0.484757379072011,0.698765466281204,
-1.06364622438512));
#58498=CARTESIAN_POINT('Ctrl Pts',(-0.756728010910764,0.388101050966172,
-1.05321226178264));
#58499=CARTESIAN_POINT('Ctrl Pts',(-0.850331447180054,-0.0140392876955686,
-1.04277829918015));
#58500=CARTESIAN_POINT('Ctrl Pts',(-0.743503406614725,-0.412872032986837,
-1.03234433657768));
#58501=CARTESIAN_POINT('Ctrl Pts',(-0.461424807647823,-0.714386145646098,
-1.02191037397519));
#58502=CARTESIAN_POINT('Ctrl Pts',(-0.070583950441432,-0.847513141979658,
-1.01147641137271));
#58503=CARTESIAN_POINT('Ctrl Pts',(0.336894159842268,-0.780873113300912,
-1.00104244877023));
#58504=CARTESIAN_POINT('Ctrl Pts',(0.664963173900127,-0.530174058353579,
-0.990608486167752));
#58505=CARTESIAN_POINT('Ctrl Pts',(0.836294104630411,-0.154507939527322,
-0.980174523565272));
#58506=CARTESIAN_POINT('Ctrl Pts',(0.810502659647238,0.25757712537611,-0.969740560962791));
#58507=CARTESIAN_POINT('Ctrl Pts',(0.593668115536935,0.608948854591682,
-0.959306598360311));
#58508=CARTESIAN_POINT('Ctrl Pts',(0.236900417487047,0.816785607236095,
-0.948872635757829));
#58509=CARTESIAN_POINT('Ctrl Pts',(-0.175706936751575,0.832098317777406,
-0.93843867315535));
#58510=CARTESIAN_POINT('Ctrl Pts',(-0.546898513860023,0.651277630891637,
-0.928004710552868));
#58511=CARTESIAN_POINT('Ctrl Pts',(-0.789180970390852,0.316944685067363,
-0.917570747950388));
#58512=CARTESIAN_POINT('Ctrl Pts',(-0.845446053461758,-0.0920951029197594,
-0.907136785347908));
#58513=CARTESIAN_POINT('Ctrl Pts',(-0.702431554241408,-0.479427209172013,
-0.896702822745426));
#58514=CARTESIAN_POINT('Ctrl Pts',(-0.393847334508687,-0.753753815530975,
-0.886268860142947));
#58515=CARTESIAN_POINT('Ctrl Pts',(0.0075704042826582,-0.850413561905815,
-0.875834897540465));
#58516=CARTESIAN_POINT('Ctrl Pts',(0.40720372762689,-0.746622837529438,
-0.865400934937985));
#58517=CARTESIAN_POINT('Ctrl Pts',(0.710855304480888,-0.46684609176493,
-0.854966972335505));
#58518=CARTESIAN_POINT('Ctrl Pts',(0.84695160373427,-0.0770293336317737,
-0.844533009733024));
#58519=CARTESIAN_POINT('Ctrl Pts',(0.783413448288198,0.330943962550491,
-0.834099047130544));
#58520=CARTESIAN_POINT('Ctrl Pts',(0.53521737866792,0.660910655746168,-0.823665084528062));
#58521=CARTESIAN_POINT('Ctrl Pts',(0.160865541628774,0.835094494547749,
-0.813231121925583));
#58522=CARTESIAN_POINT('Ctrl Pts',(-0.251403815775333,0.812438710747313,
-0.802797159323102));
#58523=CARTESIAN_POINT('Ctrl Pts',(-0.604414930500534,0.59828348556128,
-0.792363196720621));
#58524=CARTESIAN_POINT('Ctrl Pts',(-0.814959764354287,0.243107218714007,
-0.781929234118141));
#58525=CARTESIAN_POINT('Ctrl Pts',(-0.833410920788056,-0.169371704893337,
-0.771495271515659));
#58526=CARTESIAN_POINT('Ctrl Pts',(-0.65541928878181,-0.541928125492689,
-0.76106130891318));
#58527=CARTESIAN_POINT('Ctrl Pts',(-0.322939169195014,-0.786746992562985,
-0.750627346310698));
#58528=CARTESIAN_POINT('Ctrl Pts',(0.0856607483339347,-0.846122197736321,
-0.740193383708218));
#58529=CARTESIAN_POINT('Ctrl Pts',(0.474069622233808,-0.706058447001636,
-0.729759421105737));
#58530=CARTESIAN_POINT('Ctrl Pts',(0.750735829720999,-0.399570083064779,
-0.719325458503258));
#58531=CARTESIAN_POINT('Ctrl Pts',(0.850446544913026,0.00110070557588335,
-0.708891495900775));
#58532=CARTESIAN_POINT('Ctrl Pts',(0.749699014916824,0.401512047565219,
-0.698457533298296));
#58533=CARTESIAN_POINT('Ctrl Pts',(0.472240379621293,0.707283225562721,
-0.688023570695814));
#58534=CARTESIAN_POINT('Ctrl Pts',(0.0834702475924911,0.84634109853777,
-0.677589608093335));
#58535=CARTESIAN_POINT('Ctrl Pts',(-0.324974606449005,0.78590841862814,
-0.667155645490853));
#58536=CARTESIAN_POINT('Ctrl Pts',(-0.656819890853624,0.540229736580931,
-0.656721682888373));
#58537=CARTESIAN_POINT('Ctrl Pts',(-0.833846552603121,0.167213827236748,
-0.646287720285892));
#58538=CARTESIAN_POINT('Ctrl Pts',(-0.814327743398679,-0.245215953066854,
-0.635853757683411));
#58539=CARTESIAN_POINT('Ctrl Pts',(-0.602864230054735,-0.599846028100363,
-0.625419795080931));
#58540=CARTESIAN_POINT('Ctrl Pts',(-0.249299950511681,-0.813086755507764,
-0.61498583247845));
#58541=CARTESIAN_POINT('Ctrl Pts',(0.163026670890489,-0.834675291287356,
-0.604551869875971));
#58542=CARTESIAN_POINT('Ctrl Pts',(0.536926373445071,-0.659523014614649,
-0.594117907273488));
#58543=CARTESIAN_POINT('Ctrl Pts',(0.784267482446793,-0.328914963605851,
-0.58368394467101));
#58544=CARTESIAN_POINT('Ctrl Pts',(0.846749373394363,0.07922143626269,-0.573249982068528));
#58545=CARTESIAN_POINT('Ctrl Pts',(0.709644477235602,0.468684598889571,
-0.562816019466048));
#58546=CARTESIAN_POINT('Ctrl Pts',(0.405269706838339,0.74767439572747,-0.552382056863567));
#58547=CARTESIAN_POINT('Ctrl Pts',(0.00536905683500304,0.850430309041236,
-0.541948094261086));
#58548=CARTESIAN_POINT('Ctrl Pts',(-0.395797130335716,0.752731804114374,
-0.531514131658606));
#58549=CARTESIAN_POINT('Ctrl Pts',(-0.703670213228199,0.477607336964844,
-0.521080169056125));
#58550=CARTESIAN_POINT('Ctrl Pts',(-0.845681612069302,0.0899063307845272,
-0.510646206453645));
#58551=CARTESIAN_POINT('Ctrl Pts',(-0.788357905185793,-0.318986442718711,
-0.500212243851163));
#58552=CARTESIAN_POINT('Ctrl Pts',(-0.54521082915687,-0.652691113067544,
-0.489778281248684));
#58553=CARTESIAN_POINT('Ctrl Pts',(-0.173552435486475,-0.832550352497661,
-0.479344318646203));
#58554=CARTESIAN_POINT('Ctrl Pts',(0.239013898693356,-0.816169647523525,
-0.468910356043722));
#58555=CARTESIAN_POINT('Ctrl Pts',(0.595242410120839,-0.60741008429298,
-0.458476393441241));
#58556=CARTESIAN_POINT('Ctrl Pts',(0.811166689955888,-0.25547825428647,
-0.448042430838761));
#58557=CARTESIAN_POINT('Ctrl Pts',(0.835891355663177,0.15667220185756,-0.43760846823628));
#58558=CARTESIAN_POINT('Ctrl Pts',(0.663588571113163,0.531893547239619,
-0.4271745056338));
#58559=CARTESIAN_POINT('Ctrl Pts',(0.334871722342646,0.781742583516306,
-0.416740543031319));
#58560=CARTESIAN_POINT('Ctrl Pts',(-0.0727775393183082,0.84732754415147,
-0.406306580428839));
#58561=CARTESIAN_POINT('Ctrl Pts',(-0.463272450821895,0.713189437398579,
-0.395872617826358));
#58562=CARTESIAN_POINT('Ctrl Pts',(-0.74456969071411,0.410945875971156,
-0.385438655223877));
#58563=CARTESIAN_POINT('Ctrl Pts',(-0.8503648552362,0.0118385085176673,
-0.375004692621397));
#58564=CARTESIAN_POINT('Ctrl Pts',(-0.755721029601023,-0.390059306686192,
-0.364570730018916));
#58565=CARTESIAN_POINT('Ctrl Pts',(-0.482946653183773,-0.700016476572467,
-0.354136767416436));
#58566=CARTESIAN_POINT('Ctrl Pts',(-0.0963372107351823,-0.844973182506324,
-0.343702804813954));
#58567=CARTESIAN_POINT('Ctrl Pts',(0.312979817940922,-0.790761766178747,
-0.333268842211475));
#58568=CARTESIAN_POINT('Ctrl Pts',(0.648524561294601,-0.550160368159601,
-0.322834879608993));
#58569=CARTESIAN_POINT('Ctrl Pts',(0.831205969332432,-0.17988099945694,
-0.312400917006513));
#58570=CARTESIAN_POINT('Ctrl Pts',(0.817964316356759,0.232798011437269,
-0.301966954404032));
#58571=CARTESIAN_POINT('Ctrl Pts',(0.611920785515868,0.590604343299518,
-0.291532991801552));
#58572=CARTESIAN_POINT('Ctrl Pts',(0.261641771830845,0.809199678217181,
-0.281099029199071));
#58573=CARTESIAN_POINT('Ctrl Pts',(-0.150308664289158,0.837059044723433,
-0.270665066596591));
#58574=CARTESIAN_POINT('Ctrl Pts',(-0.526829940633299,0.667615720654165,
-0.26023110399411));
#58575=CARTESIAN_POINT('Ctrl Pts',(-0.779172437010211,0.340809105248274,
-0.249797141391629));
#58576=CARTESIAN_POINT('Ctrl Pts',(-0.847856686154441,-0.0663294394492073,
-0.239363178789149));
#58577=CARTESIAN_POINT('Ctrl Pts',(-0.716693103442289,-0.457833473536335,
-0.228929216186668));
#58578=CARTESIAN_POINT('Ctrl Pts',(-0.416598299086144,-0.741421929191927,
-0.218495253584188));
#58579=CARTESIAN_POINT('Ctrl Pts',(-0.0183072020772284,-0.850250118821529,
-0.208061290981707));
#58580=CARTESIAN_POINT('Ctrl Pts',(0.384298765226859,-0.758666652961295,
-0.197627328379227));
#58581=CARTESIAN_POINT('Ctrl Pts',(0.696322509060594,-0.488257754713517,
-0.187193365776746));
#58582=CARTESIAN_POINT('Ctrl Pts',(0.844215296492181,-0.102763035312441,
-0.176759403174265));
#58583=CARTESIAN_POINT('Ctrl Pts',(0.793120952222842,0.306956102035922,
-0.166325440571785));
#58584=CARTESIAN_POINT('Ctrl Pts',(0.555075924815356,0.644318467007069,
-0.155891477969304));
#58585=CARTESIAN_POINT('Ctrl Pts',(0.186203366191301,0.829817432539671,
-0.145457515366824));
#58586=CARTESIAN_POINT('Ctrl Pts',(-0.226576956355173,0.81970386523168,
-0.135023552764342));
#58587=CARTESIAN_POINT('Ctrl Pts',(-0.585915510641066,0.616411513065771,
-0.124589590161862));
#58588=CARTESIAN_POINT('Ctrl Pts',(-0.807221329288043,0.267758165995395,
-0.114155627559382));
#58589=CARTESIAN_POINT('Ctrl Pts',(-0.827788619517399,-0.00665018237018827,
-0.107199652491061));
#58590=CARTESIAN_POINT('Ctrl Pts',(-0.805186023504941,-0.13827082337233,
-0.103721664956901));
#58591=CARTESIAN_POINT('Ctrl Pts',(0.59113087362967,-0.567590438870545,
-1.12757052310293));
#58592=CARTESIAN_POINT('Ctrl Pts',(0.683912652131218,-0.470960598009107,
-1.12409253556877));
#58593=CARTESIAN_POINT('Ctrl Pts',(0.82111734424875,-0.231442668990131,
-1.11713656050045));
#58594=CARTESIAN_POINT('Ctrl Pts',(0.833311893543815,0.182619350617622,
-1.10670259789796));
#58595=CARTESIAN_POINT('Ctrl Pts',(0.649110049900926,0.553539577591918,
-1.09626863529548));
#58596=CARTESIAN_POINT('Ctrl Pts',(0.311896021207629,0.794032746862487,
-1.085834672693));
#58597=CARTESIAN_POINT('Ctrl Pts',(-0.0988293942380879,0.847340965934938,
-1.07540071009052));
#58598=CARTESIAN_POINT('Ctrl Pts',(-0.486262551456734,0.700935132557606,
-1.06496674748804));
#58599=CARTESIAN_POINT('Ctrl Pts',(-0.759077651294704,0.389306105187754,
-1.05453278488556));
#58600=CARTESIAN_POINT('Ctrl Pts',(-0.852971726711211,-0.014082879866262,
-1.04409882228308));
#58601=CARTESIAN_POINT('Ctrl Pts',(-0.745811984820576,-0.414154000672726,
-1.0336648596806));
#58602=CARTESIAN_POINT('Ctrl Pts',(-0.4628575318427,-0.716604314872258,
-1.02323089707812));
#58603=CARTESIAN_POINT('Ctrl Pts',(-0.0708031136070384,-0.850144670496582,
-1.01279693447564));
#58604=CARTESIAN_POINT('Ctrl Pts',(0.337940216291625,-0.7832977245458,-1.00236297187316));
#58605=CARTESIAN_POINT('Ctrl Pts',(0.667027884744328,-0.531820248945429,
-0.991929009270678));
#58606=CARTESIAN_POINT('Ctrl Pts',(0.838890798054124,-0.154987686725414,
-0.981495046668197));
#58607=CARTESIAN_POINT('Ctrl Pts',(0.813019270631118,0.258376902423271,
-0.971061084065717));
#58608=CARTESIAN_POINT('Ctrl Pts',(0.595511455199314,0.610839640952936,
-0.960627121463234));
#58609=CARTESIAN_POINT('Ctrl Pts',(0.237635993349262,0.819321726773045,
-0.950193158860757));
#58610=CARTESIAN_POINT('Ctrl Pts',(-0.176252506838998,0.83468198328421,
-0.939759196258273));
#58611=CARTESIAN_POINT('Ctrl Pts',(-0.548596633896843,0.653299848115927,
-0.929325233655794));
#58612=CARTESIAN_POINT('Ctrl Pts',(-0.791631377522395,0.317928798402169,
-0.918891271053314));
#58613=CARTESIAN_POINT('Ctrl Pts',(-0.848071163691741,-0.092381058239788,
-0.908457308450832));
#58614=CARTESIAN_POINT('Ctrl Pts',(-0.704612604411761,-0.480915830789204,
-0.898023345848353));
#58615=CARTESIAN_POINT('Ctrl Pts',(-0.395070230591342,-0.756094221336819,
-0.887589383245871));
#58616=CARTESIAN_POINT('Ctrl Pts',(0.00759391039004866,-0.853054096250918,
-0.877155420643392));
#58617=CARTESIAN_POINT('Ctrl Pts',(0.408468095313881,-0.748941101646619,
-0.86672145804091));
#58618=CARTESIAN_POINT('Ctrl Pts',(0.713062510398055,-0.468295649009077,
-0.856287495438431));
#58619=CARTESIAN_POINT('Ctrl Pts',(0.849581388698288,-0.0772685097340202,
-0.845853532835948));
#58620=CARTESIAN_POINT('Ctrl Pts',(0.785845947261971,0.331971543645811,
-0.835419570233469));
#58621=CARTESIAN_POINT('Ctrl Pts',(0.536879228776823,0.662962783515191,
-0.824985607630987));
#58622=CARTESIAN_POINT('Ctrl Pts',(0.161365029180057,0.837687463184462,
-0.814551645028508));
#58623=CARTESIAN_POINT('Ctrl Pts',(-0.252184424692901,0.814961333169054,
-0.804117682426026));
#58624=CARTESIAN_POINT('Ctrl Pts',(-0.606291639027032,0.600141155949544,
-0.793683719823546));
#58625=CARTESIAN_POINT('Ctrl Pts',(-0.817490214648176,0.243862066695402,
-0.783249757221066));
#58626=CARTESIAN_POINT('Ctrl Pts',(-0.835998661927778,-0.16989760408391,
-0.772815794618584));
#58627=CARTESIAN_POINT('Ctrl Pts',(-0.657454365854888,-0.543610812472342,
-0.762381832016105));
#58628=CARTESIAN_POINT('Ctrl Pts',(-0.323941895404749,-0.789189842192652,
-0.751947869413623));
#58629=CARTESIAN_POINT('Ctrl Pts',(0.0859267249812208,-0.848749407394488,
-0.741513906811143));
#58630=CARTESIAN_POINT('Ctrl Pts',(0.47554160854206,-0.708250758675002,
-0.731079944208662));
#58631=CARTESIAN_POINT('Ctrl Pts',(0.753066864680074,-0.400810748283291,
-0.720645981606182));
#58632=CARTESIAN_POINT('Ctrl Pts',(0.853087181670372,0.00110412326700143,
-0.710212019003701));
#58633=CARTESIAN_POINT('Ctrl Pts',(0.752026830565646,0.402758742584041,
-0.699778056401221));
#58634=CARTESIAN_POINT('Ctrl Pts',(0.473706686130727,0.709479340173859,
-0.68934409379874));
#58635=CARTESIAN_POINT('Ctrl Pts',(0.0837294227343689,0.848968987882985,
-0.678910131196259));
#58636=CARTESIAN_POINT('Ctrl Pts',(-0.325983652691977,0.788348664485508,
-0.668476168593779));
#58637=CARTESIAN_POINT('Ctrl Pts',(-0.658859316796523,0.541907150062543,
-0.658042205991297));
#58638=CARTESIAN_POINT('Ctrl Pts',(-0.83643564637975,0.167733026216601,
-0.647608243388819));
#58639=CARTESIAN_POINT('Ctrl Pts',(-0.816856231267325,-0.245977348668999,
-0.637174280786336));
#58640=CARTESIAN_POINT('Ctrl Pts',(-0.604736123655918,-0.601708550183643,
-0.626740318183857));
#58641=CARTESIAN_POINT('Ctrl Pts',(-0.250074026927023,-0.815611390108666,
-0.616306355581375));
#58642=CARTESIAN_POINT('Ctrl Pts',(0.163532868748728,-0.837266958297831,
-0.605872392978896));
#58643=CARTESIAN_POINT('Ctrl Pts',(0.538593529983231,-0.661570833757573,
-0.595438430376415));
#58644=CARTESIAN_POINT('Ctrl Pts',(0.786702633196865,-0.329936244658886,
-0.585004467773934));
#58645=CARTESIAN_POINT('Ctrl Pts',(0.849378530433119,0.0794674188442131,
-0.574570505171454));
#58646=CARTESIAN_POINT('Ctrl Pts',(0.711847923533838,0.470139864698849,
-0.564136542568972));
#58647=CARTESIAN_POINT('Ctrl Pts',(0.406528069390245,0.749995924933148,
-0.553702579966493));
#58648=CARTESIAN_POINT('Ctrl Pts',(0.0053857277579616,0.853070895386196,
-0.543268617364011));
#58649=CARTESIAN_POINT('Ctrl Pts',(-0.397026080534959,0.755069036574495,
-0.532834654761531));
#58650=CARTESIAN_POINT('Ctrl Pts',(-0.705855109435038,0.479090307878314,
-0.52240069215905));
#58651=CARTESIAN_POINT('Ctrl Pts',(-0.84830745370885,0.0901854899664981,
-0.511966729556569));
#58652=CARTESIAN_POINT('Ctrl Pts',(-0.7908057566996,-0.319976895711644,
-0.50153276695409));
#58653=CARTESIAN_POINT('Ctrl Pts',(-0.546903708932309,-0.654717719154274,
-0.491098804351608));
#58654=CARTESIAN_POINT('Ctrl Pts',(-0.174091315846697,-0.835135421572604,
-0.480664841749129));
#58655=CARTESIAN_POINT('Ctrl Pts',(0.239756036914954,-0.818703854504989,
-0.470230879146647));
#58656=CARTESIAN_POINT('Ctrl Pts',(0.597090637969018,-0.609296092772832,
-0.459796916544167));
#58657=CARTESIAN_POINT('Ctrl Pts',(0.813685362752721,-0.256271514336742,
-0.449362953941686));
#58658=CARTESIAN_POINT('Ctrl Pts',(0.838486798553873,0.157158669087693,
-0.438928991339206));
#58659=CARTESIAN_POINT('Ctrl Pts',(0.665649013810141,0.533545076851018,
-0.428495028736725));
#58660=CARTESIAN_POINT('Ctrl Pts',(0.335911499133207,0.784169894454499,
-0.418061066134244));
#58661=CARTESIAN_POINT('Ctrl Pts',(-0.0730035135980353,0.849958496410589,
-0.407627103531764));
#58662=CARTESIAN_POINT('Ctrl Pts',(-0.464710911909924,0.715403890799101,
-0.397193140929283));
#58663=CARTESIAN_POINT('Ctrl Pts',(-0.746881579809863,0.412221863029791,
-0.386759178326802));
#58664=CARTESIAN_POINT('Ctrl Pts',(-0.853005238347077,0.01187526708989,
-0.376325215724322));
#58665=CARTESIAN_POINT('Ctrl Pts',(-0.758067543607107,-0.391270440941413,
-0.365891253121841));
#58666=CARTESIAN_POINT('Ctrl Pts',(-0.484446202675581,-0.702190027925983,
-0.355457290519361));
#58667=CARTESIAN_POINT('Ctrl Pts',(-0.0966363378011808,-0.847596824471873,
-0.34502332791688));
#58668=CARTESIAN_POINT('Ctrl Pts',(0.313951620362259,-0.793217081681621,
-0.3345893653144));
#58669=CARTESIAN_POINT('Ctrl Pts',(0.650538230236919,-0.551868616254977,
-0.324155402711919));
#58670=CARTESIAN_POINT('Ctrl Pts',(0.833786864097282,-0.180439530010112,
-0.313721440109438));
#58671=CARTESIAN_POINT('Ctrl Pts',(0.820504095785433,0.233520849327355,
-0.303287477506958));
#58672=CARTESIAN_POINT('Ctrl Pts',(0.613820799724295,0.592438169948661,
-0.292853514904477));
#58673=CARTESIAN_POINT('Ctrl Pts',(0.262454169604739,0.811712243442553,
-0.282419552301996));
#58674=CARTESIAN_POINT('Ctrl Pts',(-0.150775372733263,0.839658113287937,
-0.271985589699516));
#58675=CARTESIAN_POINT('Ctrl Pts',(-0.528465747745014,0.66968866765364,
-0.261551627097035));
#58676=CARTESIAN_POINT('Ctrl Pts',(-0.78159176764234,0.341867317610358,
-0.251117664494555));
#58677=CARTESIAN_POINT('Ctrl Pts',(-0.850489281400512,-0.0665353923691108,
-0.240683701892074));
#58678=CARTESIAN_POINT('Ctrl Pts',(-0.718918435725102,-0.459255046614004,
-0.230249739289594));
#58679=CARTESIAN_POINT('Ctrl Pts',(-0.417891836923547,-0.743724044456582,
-0.219815776687113));
#58680=CARTESIAN_POINT('Ctrl Pts',(-0.0183640459379991,-0.852890145736156,
-0.209381814084632));
#58681=CARTESIAN_POINT('Ctrl Pts',(0.385492012985996,-0.761022313010095,
-0.198947851482152));
#58682=CARTESIAN_POINT('Ctrl Pts',(0.698484590670027,-0.489773795410247,
-0.188513888879671));
#58683=CARTESIAN_POINT('Ctrl Pts',(0.846836585170214,-0.103082114107112,
-0.17807992627719));
#58684=CARTESIAN_POINT('Ctrl Pts',(0.795583593099748,0.307909199916563,
-0.16764596367471));
#58685=CARTESIAN_POINT('Ctrl Pts',(0.556799435517521,0.646319077797019,
-0.157212001072229));
#58686=CARTESIAN_POINT('Ctrl Pts',(0.186781528084307,0.83239401241337,-0.146778038469749));
#58687=CARTESIAN_POINT('Ctrl Pts',(-0.227280478634921,0.822249052826759,
-0.136344075867268));
#58688=CARTESIAN_POINT('Ctrl Pts',(-0.587734776932399,0.618325457284273,
-0.125910113264787));
#58689=CARTESIAN_POINT('Ctrl Pts',(-0.809727755002957,0.268589584372264,
-0.115476150662307));
#58690=CARTESIAN_POINT('Ctrl Pts',(-0.830358898319076,-0.00667087734731289,
-0.108520175593986));
#58691=CARTESIAN_POINT('Ctrl Pts',(-0.807686129085189,-0.138700154790173,
-0.105042188059826));
#58692=CARTESIAN_POINT('Ctrl Pts',(0.594875448103835,-0.571185894232442,
-1.13205842314276));
#58693=CARTESIAN_POINT('Ctrl Pts',(0.688244416305429,-0.473944510369919,
-1.1285804356086));
#58694=CARTESIAN_POINT('Ctrl Pts',(0.826319063393535,-0.23290837533709,
-1.12162446054028));
#58695=CARTESIAN_POINT('Ctrl Pts',(0.83859038834421,0.183775983334779,-1.1111904979378));
#58696=CARTESIAN_POINT('Ctrl Pts',(0.653221937147493,0.557046083095294,
-1.10075653533532));
#58697=CARTESIAN_POINT('Ctrl Pts',(0.313871699922475,0.799062532067006,
-1.09032257273284));
#58698=CARTESIAN_POINT('Ctrl Pts',(-0.0994554132647858,0.852708501700447,
-1.07988861013036));
#58699=CARTESIAN_POINT('Ctrl Pts',(-0.489342809626878,0.705375220702394,
-1.06945464752788));
#58700=CARTESIAN_POINT('Ctrl Pts',(-0.763886051959433,0.391772185135788,
-1.0590206849254));
#58701=CARTESIAN_POINT('Ctrl Pts',(-0.858374910495865,-0.0141720913963219,
-1.04858672232292));
#58702=CARTESIAN_POINT('Ctrl Pts',(-0.75053635735818,-0.416777473112896,
-1.03815275972044));
#58703=CARTESIAN_POINT('Ctrl Pts',(-0.465789520808082,-0.721143672414923,
-1.02771879711796));
#58704=CARTESIAN_POINT('Ctrl Pts',(-0.0712516182343091,-0.855529943231548,
-1.01728483451548));
#58705=CARTESIAN_POINT('Ctrl Pts',(0.340080911027159,-0.788259553404192,
-1.006850871913));
#58706=CARTESIAN_POINT('Ctrl Pts',(0.671253197851214,-0.53518908404983,
-0.996416909310516));
#58707=CARTESIAN_POINT('Ctrl Pts',(0.844204783065116,-0.155969462060879,
-0.985982946708035));
#58708=CARTESIAN_POINT('Ctrl Pts',(0.818169371553483,0.260013600576981,
-0.975548984105555));
#58709=CARTESIAN_POINT('Ctrl Pts',(0.599283744716546,0.614709027432673,
-0.965115021503073));
#58710=CARTESIAN_POINT('Ctrl Pts',(0.239141307420071,0.82451175082322,-0.954681058900594));
#58711=CARTESIAN_POINT('Ctrl Pts',(-0.177368984921704,0.839969307441941,
-0.944247096298111));
#58712=CARTESIAN_POINT('Ctrl Pts',(-0.552071739738338,0.657438200377167,
-0.933813133695633));
#58713=CARTESIAN_POINT('Ctrl Pts',(-0.796645996016163,0.31994273023519,
-0.923379171093151));
#58714=CARTESIAN_POINT('Ctrl Pts',(-0.853443302115344,-0.092966249499057,
-0.912945208490671));
#58715=CARTESIAN_POINT('Ctrl Pts',(-0.709075999240425,-0.483962210060304,
-0.90251124588819));
#58716=CARTESIAN_POINT('Ctrl Pts',(-0.397572817705153,-0.760883728388117,
-0.89207728328571));
#58717=CARTESIAN_POINT('Ctrl Pts',(0.00764201429865589,-0.858457799247159,
-0.881643320683229));
#58718=CARTESIAN_POINT('Ctrl Pts',(0.411055551701718,-0.753685296994478,
-0.871209358080748));
#58719=CARTESIAN_POINT('Ctrl Pts',(0.717579431471203,-0.471262085267673,
-0.860775395478267));
#58720=CARTESIAN_POINT('Ctrl Pts',(0.854963093698934,-0.077757969991451,
-0.850341432875787));
#58721=CARTESIAN_POINT('Ctrl Pts',(0.790823917731154,0.334074429773344,
-0.839907470273306));
#58722=CARTESIAN_POINT('Ctrl Pts',(0.540280110279979,0.667162345999428,
-0.829473507670825));
#58723=CARTESIAN_POINT('Ctrl Pts',(0.162387201977175,0.842993825670224,
-0.819039545068346));
#58724=CARTESIAN_POINT('Ctrl Pts',(-0.253781896338945,0.82012373613643,
-0.808605582465865));
#58725=CARTESIAN_POINT('Ctrl Pts',(-0.610132216032369,0.60394277249038,
-0.798171619863384));
#58726=CARTESIAN_POINT('Ctrl Pts',(-0.822668636909621,0.245406820054244,
-0.787737657260904));
#58727=CARTESIAN_POINT('Ctrl Pts',(-0.841294326638981,-0.170973826795068,
-0.777303694658423));
#58728=CARTESIAN_POINT('Ctrl Pts',(-0.661619035061959,-0.547054335443539,
-0.766869732055942));
#58729=CARTESIAN_POINT('Ctrl Pts',(-0.325993917425955,-0.794188994689023,
-0.756435769453461));
#58730=CARTESIAN_POINT('Ctrl Pts',(0.0864710310261406,-0.854125842178519,
-0.746001806850981));
#58731=CARTESIAN_POINT('Ctrl Pts',(0.478553944601615,-0.71273719952737,
-0.735567844248499));
#58732=CARTESIAN_POINT('Ctrl Pts',(0.757837194827812,-0.403349698920676,
-0.725133881646021));
#58733=CARTESIAN_POINT('Ctrl Pts',(0.858491094247377,0.00111111737702571,
-0.714699919043538));
#58734=CARTESIAN_POINT('Ctrl Pts',(0.756790572578487,0.405310032863995,
-0.704265956441059));
#58735=CARTESIAN_POINT('Ctrl Pts',(0.476707398805814,0.713973563521563,
-0.693831993838578));
#58736=CARTESIAN_POINT('Ctrl Pts',(0.084259809886235,0.854346813607812,
-0.683398031236097));
#58737=CARTESIAN_POINT('Ctrl Pts',(-0.328048608300887,0.793342488510314,
-0.672964068633617));
#58738=CARTESIAN_POINT('Ctrl Pts',(-0.663032885717748,0.545339881120648,
-0.662530106031136));
#58739=CARTESIAN_POINT('Ctrl Pts',(-0.841734079185264,0.168795537328509,
-0.652096143428656));
#58740=CARTESIAN_POINT('Ctrl Pts',(-0.822030637537395,-0.247535501360414,
-0.641662180826174));
#58741=CARTESIAN_POINT('Ctrl Pts',(-0.608566847191108,-0.605520095441727,
-0.631228218223695));
#58742=CARTESIAN_POINT('Ctrl Pts',(-0.251658130179691,-0.820777910885976,
-0.620794255621213));
#58743=CARTESIAN_POINT('Ctrl Pts',(0.164568773806467,-0.842570657079702,
-0.610360293018733));
#58744=CARTESIAN_POINT('Ctrl Pts',(0.542005270791329,-0.665761578884141,
-0.599926330416252));
#58745=CARTESIAN_POINT('Ctrl Pts',(0.791686030375065,-0.332026238109064,
-0.589492367813772));
#58746=CARTESIAN_POINT('Ctrl Pts',(0.85475895042051,0.0799708081734412,
-0.57905840521129));
#58747=CARTESIAN_POINT('Ctrl Pts',(0.716357150761197,0.473117983210515,
-0.568624442608811));
#58748=CARTESIAN_POINT('Ctrl Pts',(0.409103236611469,0.754746802098496,
-0.558190480006329));
#58749=CARTESIAN_POINT('Ctrl Pts',(0.00541984385136075,0.858474704797127,
-0.54775651740385));
#58750=CARTESIAN_POINT('Ctrl Pts',(-0.399541057053304,0.759852049554789,
-0.537322554801368));
#58751=CARTESIAN_POINT('Ctrl Pts',(-0.710326374957925,0.482125123306199,
-0.526888592198889));
#58752=CARTESIAN_POINT('Ctrl Pts',(-0.853681088920773,0.090756773317092,
-0.516454629596408));
#58753=CARTESIAN_POINT('Ctrl Pts',(-0.795815145266697,-0.322003801294379,
-0.506020666993927));
#58754=CARTESIAN_POINT('Ctrl Pts',(-0.550368090878974,-0.658865052970729,
-0.495586704391446));
#58755=CARTESIAN_POINT('Ctrl Pts',(-0.175194103781465,-0.840425618055573,
-0.485152741788965));
#58756=CARTESIAN_POINT('Ctrl Pts',(0.241274780474974,-0.823889964613383,
-0.474718779186485));
#58757=CARTESIAN_POINT('Ctrl Pts',(0.600872930889906,-0.613155701602504,
-0.464284816584005));
#58758=CARTESIAN_POINT('Ctrl Pts',(0.818839683037894,-0.257894875804606,
-0.453850853981524));
#58759=CARTESIAN_POINT('Ctrl Pts',(0.843798224459354,0.158154196539887,
-0.443416891379044));
#58760=CARTESIAN_POINT('Ctrl Pts',(0.669865592320389,0.536924838044416,
-0.432982928776562));
#58761=CARTESIAN_POINT('Ctrl Pts',(0.338039343055762,0.78913724790465,-0.422548966174082));
#58762=CARTESIAN_POINT('Ctrl Pts',(-0.0734659570783441,0.855342590214102,
-0.412115003571602));
#58763=CARTESIAN_POINT('Ctrl Pts',(-0.467654640517619,0.719935643433754,
-0.401681040969121));
#58764=CARTESIAN_POINT('Ctrl Pts',(-0.751612729039848,0.414833097799243,
-0.391247078366641));
#58765=CARTESIAN_POINT('Ctrl Pts',(-0.85840863185104,0.0119504914122616,
-0.380813115764159));
#58766=CARTESIAN_POINT('Ctrl Pts',(-0.762869550742065,-0.393748958145996,
-0.370379153161679));
#58767=CARTESIAN_POINT('Ctrl Pts',(-0.487514945218854,-0.706638076853403,
-0.359945190559198));
#58768=CARTESIAN_POINT('Ctrl Pts',(-0.0972484842880521,-0.852965958176228,
-0.349511227956718));
#58769=CARTESIAN_POINT('Ctrl Pts',(0.315940358613552,-0.798241744877078,
-0.339077265354237));
#58770=CARTESIAN_POINT('Ctrl Pts',(0.654659088924843,-0.555364448591695,
-0.328643302751756));
#58771=CARTESIAN_POINT('Ctrl Pts',(0.839068518092748,-0.181582530945499,
-0.318209340149276));
#58772=CARTESIAN_POINT('Ctrl Pts',(0.825701609589117,0.23500009586131,-0.307775377546795));
#58773=CARTESIAN_POINT('Ctrl Pts',(0.617709070479456,0.596190991632762,
-0.297341414944315));
#58774=CARTESIAN_POINT('Ctrl Pts',(0.264116695332044,0.816854064938795,
-0.286907452341834));
#58775=CARTESIAN_POINT('Ctrl Pts',(-0.151730464954603,0.844976958912708,
-0.276473489739354));
#58776=CARTESIAN_POINT('Ctrl Pts',(-0.531813333742569,0.673930835536438,
-0.266039527136873));
#58777=CARTESIAN_POINT('Ctrl Pts',(-0.786542789844424,0.344032888819267,
-0.255605564534393));
#58778=CARTESIAN_POINT('Ctrl Pts',(-0.855876737496279,-0.0669568631605798,
-0.245171601931911));
#58779=CARTESIAN_POINT('Ctrl Pts',(-0.723472451346344,-0.462164215102111,
-0.234737639329432));
#58780=CARTESIAN_POINT('Ctrl Pts',(-0.420538988411855,-0.748435191644752,
-0.22430367672695));
#58781=CARTESIAN_POINT('Ctrl Pts',(-0.0184803735586183,-0.858292811196645,
-0.21386971412447));
#58782=CARTESIAN_POINT('Ctrl Pts',(0.387933926300151,-0.765843035246912,
-0.203435751521989));
#58783=CARTESIAN_POINT('Ctrl Pts',(0.702909167805231,-0.492876289710399,
-0.193001788919509));
#58784=CARTESIAN_POINT('Ctrl Pts',(0.852200902248736,-0.103735083894892,
-0.182567826317028));
#58785=CARTESIAN_POINT('Ctrl Pts',(0.800623248743806,0.309859647074913,
-0.172133863714547));
#58786=CARTESIAN_POINT('Ctrl Pts',(0.560326498983083,0.650413239900031,
-0.161699901112067));
#58787=CARTESIAN_POINT('Ctrl Pts',(0.187964709191458,0.837666784744464,
-0.151265938509586));
#58788=CARTESIAN_POINT('Ctrl Pts',(-0.228720208214099,0.827457735607706,
-0.140831975907105));
#58789=CARTESIAN_POINT('Ctrl Pts',(-0.591457779048179,0.622242032554339,
-0.130398013304625));
#58790=CARTESIAN_POINT('Ctrl Pts',(-0.814857060568085,0.270291466147323,
-0.119964050702144));
#58791=CARTESIAN_POINT('Ctrl Pts',(-0.83561875211749,-0.00671391055875398,
-0.113008075633824));
#58792=CARTESIAN_POINT('Ctrl Pts',(-0.812802493323685,-0.139578764049745,
-0.109530088099664));
#58793=CARTESIAN_POINT('Ctrl Pts',(0.596426278379627,-0.572674966240212,
-1.13871522674109));
#58794=CARTESIAN_POINT('Ctrl Pts',(0.690040836764286,-0.475177806505636,
-1.13523723920693));
#58795=CARTESIAN_POINT('Ctrl Pts',(0.828472169960176,-0.233517118585343,
-1.12828126413861));
#58796=CARTESIAN_POINT('Ctrl Pts',(0.840777371648049,0.1842558308649,-1.11784730153613));
#58797=CARTESIAN_POINT('Ctrl Pts',(0.654924723121757,0.558498066470774,
-1.10741333893365));
#58798=CARTESIAN_POINT('Ctrl Pts',(0.314690182553946,0.801146035838714,
-1.09697937633117));
#58799=CARTESIAN_POINT('Ctrl Pts',(-0.0997147922563187,0.854931601464747,
-1.08654541372869));
#58800=CARTESIAN_POINT('Ctrl Pts',(-0.490618589981848,0.707214329023195,
-1.07611145112621));
#58801=CARTESIAN_POINT('Ctrl Pts',(-0.765877684119502,0.392793594264132,
-1.06567748852373));
#58802=CARTESIAN_POINT('Ctrl Pts',(-0.860612864682261,-0.0142090290307373,
-1.05524352592125));
#58803=CARTESIAN_POINT('Ctrl Pts',(-0.752493169135759,-0.417864105985997,
-1.04480956331877));
#58804=CARTESIAN_POINT('Ctrl Pts',(-0.467003929674391,-0.723023842952482,
-1.03437560071629));
#58805=CARTESIAN_POINT('Ctrl Pts',(-0.0714373875773983,-0.857760491803007,
-1.02394163811381));
#58806=CARTESIAN_POINT('Ctrl Pts',(0.340967574370286,-0.790314711499322,
-1.01350767551132));
#58807=CARTESIAN_POINT('Ctrl Pts',(0.673003296155669,-0.536584435271311,
-1.00307371290884));
#58808=CARTESIAN_POINT('Ctrl Pts',(0.846405803153587,-0.156376107134292,
-0.992639750306363));
#58809=CARTESIAN_POINT('Ctrl Pts',(0.820302511565669,0.260691510764421,
-0.982205787703882));
#58810=CARTESIAN_POINT('Ctrl Pts',(0.600846203873045,0.616311703562283,
-0.971771825101402));
#58811=CARTESIAN_POINT('Ctrl Pts',(0.239764799219732,0.826661426818634,
-0.961337862498921));
#58812=CARTESIAN_POINT('Ctrl Pts',(-0.177831423260388,0.842159284588734,
-0.950903899896442));
#58813=CARTESIAN_POINT('Ctrl Pts',(-0.553511107201048,0.659152280411276,
-0.940469937293959));
#58814=CARTESIAN_POINT('Ctrl Pts',(-0.798723020136244,0.320776888411997,
-0.930035974691481));
#58815=CARTESIAN_POINT('Ctrl Pts',(-0.855668408795538,-0.0932086321197877,
-0.919602012088999));
#58816=CARTESIAN_POINT('Ctrl Pts',(-0.710924709912798,-0.485224001607961,
-0.909168049486517));
#58817=CARTESIAN_POINT('Ctrl Pts',(-0.398609373888874,-0.762867512737827,
-0.89873408688404));
#58818=CARTESIAN_POINT('Ctrl Pts',(0.00766193864182875,-0.860695979777121,
-0.888300124281556));
#58819=CARTESIAN_POINT('Ctrl Pts',(0.412127260215948,-0.755650313515053,
-0.877866161679077));
#58820=CARTESIAN_POINT('Ctrl Pts',(0.719450312385613,-0.472490764912427,
-0.867432199076596));
#58821=CARTESIAN_POINT('Ctrl Pts',(0.857192162794717,-0.0779607014182988,
-0.856998236474115));
#58822=CARTESIAN_POINT('Ctrl Pts',(0.792885762468365,0.334945432267616,
-0.846564273871635));
#58823=CARTESIAN_POINT('Ctrl Pts',(0.541688734471801,0.668901778939057,
-0.836130311269154));
#58824=CARTESIAN_POINT('Ctrl Pts',(0.162810579659971,0.845191688359986,
-0.825696348666674));
#58825=CARTESIAN_POINT('Ctrl Pts',(-0.254443559264954,0.822261971679499,
-0.815262386064192));
#58826=CARTESIAN_POINT('Ctrl Pts',(-0.611722959395606,0.605517378668961,
-0.804828423461713));
#58827=CARTESIAN_POINT('Ctrl Pts',(-0.824813507545726,0.246046647390084,
-0.794394460859231));
#58828=CARTESIAN_POINT('Ctrl Pts',(-0.84348775837634,-0.171419591619667,
-0.783960498256752));
#58829=CARTESIAN_POINT('Ctrl Pts',(-0.663344015420907,-0.548480621469044,
-0.77352653565427));
#58830=CARTESIAN_POINT('Ctrl Pts',(-0.326843852320352,-0.79625961289154,
-0.76309257305179));
#58831=CARTESIAN_POINT('Ctrl Pts',(0.0866964792406474,-0.856352728383039,
-0.752658610449309));
#58832=CARTESIAN_POINT('Ctrl Pts',(0.479801635661557,-0.71459545572183,
-0.742224647846828));
#58833=CARTESIAN_POINT('Ctrl Pts',(0.759813036221547,-0.404401316651656,
-0.731790685244349));
#58834=CARTESIAN_POINT('Ctrl Pts',(0.860729361584666,0.00111401429436048,
-0.721356722641867));
#58835=CARTESIAN_POINT('Ctrl Pts',(0.758763685207286,0.406366761598998,
-0.710922760039387));
#58836=CARTESIAN_POINT('Ctrl Pts',(0.477950275531433,0.715835043177703,
-0.700488797436906));
#58837=CARTESIAN_POINT('Ctrl Pts',(0.0844794929808862,0.856574275931451,
-0.690054834834426));
#58838=CARTESIAN_POINT('Ctrl Pts',(-0.328903900207727,0.795410899692695,
-0.679620872231945));
#58839=CARTESIAN_POINT('Ctrl Pts',(-0.664761552283533,0.546761697202158,
-0.669186909629465));
#58840=CARTESIAN_POINT('Ctrl Pts',(-0.843928657450257,0.16923562289307,
-0.658752947026984));
#58841=CARTESIAN_POINT('Ctrl Pts',(-0.82417384477458,-0.248180878617356,
-0.648318984424504));
#58842=CARTESIAN_POINT('Ctrl Pts',(-0.610153509307644,-0.607098814033897,
-0.637885021822023));
#58843=CARTESIAN_POINT('Ctrl Pts',(-0.252314255999422,-0.822917852000584,
-0.627451059219542));
#58844=CARTESIAN_POINT('Ctrl Pts',(0.164997839307108,-0.844767416479698,
-0.617017096617061));
#58845=CARTESIAN_POINT('Ctrl Pts',(0.543418392840445,-0.667497359728489,
-0.606583134014581));
#58846=CARTESIAN_POINT('Ctrl Pts',(0.793750122821745,-0.33289190053569,
-0.596149171412101));
#58847=CARTESIAN_POINT('Ctrl Pts',(0.856987487271739,0.0801793089360829,
-0.58571520880962));
#58848=CARTESIAN_POINT('Ctrl Pts',(0.718224844931966,0.474351501572674,
-0.575281246207139));
#58849=CARTESIAN_POINT('Ctrl Pts',(0.410169855028622,0.756714586186626,
-0.564847283604659));
#58850=CARTESIAN_POINT('Ctrl Pts',(0.0054339745273192,0.860712929403662,
-0.554413321002177));
#58851=CARTESIAN_POINT('Ctrl Pts',(-0.4005827448517,0.761833144099726,-0.543979358399698));
#58852=CARTESIAN_POINT('Ctrl Pts',(-0.712178345624292,0.483382125182182,
-0.533545395797216));
#58853=CARTESIAN_POINT('Ctrl Pts',(-0.855906815559752,0.0909933953656075,
-0.523111433194736));
#58854=CARTESIAN_POINT('Ctrl Pts',(-0.797890003186724,-0.32284333311451,
-0.512677470592255));
#58855=CARTESIAN_POINT('Ctrl Pts',(-0.551803016563766,-0.660582853117555,
-0.502243507989775));
#58856=CARTESIAN_POINT('Ctrl Pts',(-0.175650871758218,-0.842616784886446,
-0.491809545387294));
#58857=CARTESIAN_POINT('Ctrl Pts',(0.24190383471219,-0.826038019508388,
-0.481375582784813));
#58858=CARTESIAN_POINT('Ctrl Pts',(0.602439533344009,-0.614754327830273,
-0.470941620182333));
#58859=CARTESIAN_POINT('Ctrl Pts',(0.820974570783732,-0.258567262135502,
-0.460507657579852));
#58860=CARTESIAN_POINT('Ctrl Pts',(0.845998184386402,0.15856653788477,-0.450073694977372));
#58861=CARTESIAN_POINT('Ctrl Pts',(0.671612073193297,0.538324714333902,
-0.439639732374891));
#58862=CARTESIAN_POINT('Ctrl Pts',(0.338920682915139,0.791194695137899,
-0.429205769772411));
#58863=CARTESIAN_POINT('Ctrl Pts',(-0.0736574983223148,0.85757264873735,
-0.41877180716993));
#58864=CARTESIAN_POINT('Ctrl Pts',(-0.468873914793169,0.72181266748964,
-0.40833784456745));
#58865=CARTESIAN_POINT('Ctrl Pts',(-0.753572341938536,0.415914655172892,
-0.397903881964969));
#58866=CARTESIAN_POINT('Ctrl Pts',(-0.860646684191481,0.0119816488637972,
-0.387469919362488));
#58867=CARTESIAN_POINT('Ctrl Pts',(-0.764858512548966,-0.394775544721155,
-0.377035956760008));
#58868=CARTESIAN_POINT('Ctrl Pts',(-0.488785999497304,-0.708480431348439,
-0.366601994157527));
#58869=CARTESIAN_POINT('Ctrl Pts',(-0.097502031596093,-0.855189820319157,
-0.356168031555046));
#58870=CARTESIAN_POINT('Ctrl Pts',(0.316764081759707,-0.800322929452836,
-0.345734068952566));
#58871=CARTESIAN_POINT('Ctrl Pts',(0.656365923236636,-0.556812400837165,
-0.335300106350085));
#58872=CARTESIAN_POINT('Ctrl Pts',(0.841256146677281,-0.182055954894471,
-0.324866143747605));
#58873=CARTESIAN_POINT('Ctrl Pts',(0.82785438782568,0.235612790663162,-0.314432181145124));
#58874=CARTESIAN_POINT('Ctrl Pts',(0.619319568298153,0.597745387301998,
-0.303998218542643));
#58875=CARTESIAN_POINT('Ctrl Pts',(0.264805303262618,0.818983775723725,
-0.293564255940163));
#58876=CARTESIAN_POINT('Ctrl Pts',(-0.152126058284342,0.847179992119361,
-0.283130293337682));
#58877=CARTESIAN_POINT('Ctrl Pts',(-0.533199883246888,0.675687915217586,
-0.272696330735201));
#58878=CARTESIAN_POINT('Ctrl Pts',(-0.788593472808699,0.344929855388104,
-0.262262368132721));
#58879=CARTESIAN_POINT('Ctrl Pts',(-0.85810818859447,-0.0671314343578934,
-0.25182840553024));
#58880=CARTESIAN_POINT('Ctrl Pts',(-0.725358696723669,-0.463369173631081,
-0.24139444292776));
#58881=CARTESIAN_POINT('Ctrl Pts',(-0.421635422015108,-0.750386522096553,
-0.230960480325279));
#58882=CARTESIAN_POINT('Ctrl Pts',(-0.0185285562433264,-0.86053055751242,
-0.220526517722799));
#58883=CARTESIAN_POINT('Ctrl Pts',(0.388945352751925,-0.767839757527659,
-0.210092555120318));
#58884=CARTESIAN_POINT('Ctrl Pts',(0.704741798496444,-0.494161306472494,
-0.199658592517837));
#58885=CARTESIAN_POINT('Ctrl Pts',(0.85442277317254,-0.104005573943575,
-0.189224629915356));
#58886=CARTESIAN_POINT('Ctrl Pts',(0.802710635634205,0.310667577083989,
-0.178790667312876));
#58887=CARTESIAN_POINT('Ctrl Pts',(0.561787401645997,0.65210888533253,-0.168356704710395));
#58888=CARTESIAN_POINT('Ctrl Pts',(0.188454746657775,0.839850992854137,
-0.157922742107915));
#58889=CARTESIAN_POINT('Ctrl Pts',(-0.229316478451303,0.82961463096934,
-0.147488779505434));
#58890=CARTESIAN_POINT('Ctrl Pts',(-0.592999937130298,0.623865269466558,
-0.137054816902954));
#58891=CARTESIAN_POINT('Ctrl Pts',(-0.816981345420961,0.270994210833144,
-0.126620854300473));
#58892=CARTESIAN_POINT('Ctrl Pts',(-0.837797728572329,-0.00672831308055416,
-0.119664879232153));
#58893=CARTESIAN_POINT('Ctrl Pts',(-0.814921455736579,-0.139942643537184,
-0.116186891697993));
#58894=CARTESIAN_POINT('Ctrl Pts',(0.596426278379627,-0.572674966240212,
-1.1425283350431));
#58895=CARTESIAN_POINT('Ctrl Pts',(0.690039237300982,-0.475179472305614,
-1.13905034750894));
#58896=CARTESIAN_POINT('Ctrl Pts',(0.828472972546818,-0.233515977058058,
-1.13209437244062));
#58897=CARTESIAN_POINT('Ctrl Pts',(0.840776790045671,0.184255282770983,
-1.12166040983814));
#58898=CARTESIAN_POINT('Ctrl Pts',(0.654924835154713,0.558498232654793,
-1.11122644723566));
#58899=CARTESIAN_POINT('Ctrl Pts',(0.31469001782895,0.801145770682762,-1.10079248463318));
#58900=CARTESIAN_POINT('Ctrl Pts',(-0.0997147185513737,0.854931525810344,
-1.0903585220307));
#58901=CARTESIAN_POINT('Ctrl Pts',(-0.490618537208114,0.707214177068778,
-1.07992455942821));
#58902=CARTESIAN_POINT('Ctrl Pts',(-0.765877541643967,0.392793546079614,
-1.06949059682574));
#58903=CARTESIAN_POINT('Ctrl Pts',(-0.860612728693632,-0.0142090354680717,
-1.05905663422325));
#58904=CARTESIAN_POINT('Ctrl Pts',(-0.752493039839581,-0.417864031829521,
-1.04862267162078));
#58905=CARTESIAN_POINT('Ctrl Pts',(-0.467003853748621,-0.723023724671482,
-1.03818870901829));
#58906=CARTESIAN_POINT('Ctrl Pts',(-0.0714373746764586,-0.857760347616996,
-1.02775474641581));
#58907=CARTESIAN_POINT('Ctrl Pts',(0.340967517012704,-0.790314580308694,
-1.01732078381333));
#58908=CARTESIAN_POINT('Ctrl Pts',(0.673003184192233,-0.53658434549891,
-1.00688682121085));
#58909=CARTESIAN_POINT('Ctrl Pts',(0.846405661890071,-0.15637608121211,
-0.99645285860837));
#58910=CARTESIAN_POINT('Ctrl Pts',(0.820302374851198,0.26069146737326,-0.986018896005891));
#58911=CARTESIAN_POINT('Ctrl Pts',(0.600846103651701,0.616311600756356,
-0.975584933403409));
#58912=CARTESIAN_POINT('Ctrl Pts',(0.239764759257477,0.826661288997697,
-0.96515097080093));
#58913=CARTESIAN_POINT('Ctrl Pts',(-0.177831393616744,0.842159144153302,
-0.954717008198447));
#58914=CARTESIAN_POINT('Ctrl Pts',(-0.553511014901823,0.65915217050663,
-0.944283045595968));
#58915=CARTESIAN_POINT('Ctrl Pts',(-0.798722886956037,0.320776834921653,
-0.933849082993487));
#58916=CARTESIAN_POINT('Ctrl Pts',(-0.855668266116612,-0.0932086165764395,
-0.923415120391007));
#58917=CARTESIAN_POINT('Ctrl Pts',(-0.710924591370782,-0.485223920700338,
-0.912981157788526));
#58918=CARTESIAN_POINT('Ctrl Pts',(-0.39860930742276,-0.762867385533715,
-0.902547195186045));
#58919=CARTESIAN_POINT('Ctrl Pts',(0.0076619373640938,-0.860695836261201,
-0.892113232583565));
#58920=CARTESIAN_POINT('Ctrl Pts',(0.412127191496178,-0.755650187514626,
-0.881679269981083));
#58921=CARTESIAN_POINT('Ctrl Pts',(0.719450192421379,-0.472490686127359,
-0.871245307378604));
#58922=CARTESIAN_POINT('Ctrl Pts',(0.857192019862881,-0.0779606884187777,
-0.860811344776123));
#58923=CARTESIAN_POINT('Ctrl Pts',(0.792885630259222,0.334945376417383,
-0.850377382173642));
#58924=CARTESIAN_POINT('Ctrl Pts',(0.54168864414833,0.668901667403545,-0.839943419571162));
#58925=CARTESIAN_POINT('Ctrl Pts',(0.162810552512241,0.845191547429137,
-0.829509456968682));
#58926=CARTESIAN_POINT('Ctrl Pts',(-0.254443516837955,0.822261834572054,
-0.8190754943662));
#58927=CARTESIAN_POINT('Ctrl Pts',(-0.611722857394327,0.605517277702424,
-0.80864153176372));
#58928=CARTESIAN_POINT('Ctrl Pts',(-0.824813370012824,0.246046606363224,
-0.798207569161239));
#58929=CARTESIAN_POINT('Ctrl Pts',(-0.843487617729615,-0.171419563036438,
-0.787773606558758));
#58930=CARTESIAN_POINT('Ctrl Pts',(-0.663343904812114,-0.54848053001306,
-0.777339643956279));
#58931=CARTESIAN_POINT('Ctrl Pts',(-0.326843797821022,-0.796259480119837,
-0.766905681353797));
#58932=CARTESIAN_POINT('Ctrl Pts',(0.0866964647845083,-0.856352585591155,
-0.756471718751317));
#58933=CARTESIAN_POINT('Ctrl Pts',(0.479801555657399,-0.714595336567154,
-0.746037756148836));
#58934=CARTESIAN_POINT('Ctrl Pts',(0.7598129095271,-0.404401249220066,-0.735603793546356));
#58935=CARTESIAN_POINT('Ctrl Pts',(0.860729218063003,0.00111401410860473,
-0.725169830943875));
#58936=CARTESIAN_POINT('Ctrl Pts',(0.758763558687812,0.406366693839682,
-0.714735868341394));
#58937=CARTESIAN_POINT('Ctrl Pts',(0.477950195835978,0.715834923816333,
-0.704301905738914));
#58938=CARTESIAN_POINT('Ctrl Pts',(0.0844794788944169,0.856574133102626,
-0.693867943136433));
#58939=CARTESIAN_POINT('Ctrl Pts',(-0.328903845364895,0.795410767062509,
-0.683433980533953));
#58940=CARTESIAN_POINT('Ctrl Pts',(-0.664761441438374,0.546761606032795,
-0.673000017931472));
#58941=CARTESIAN_POINT('Ctrl Pts',(-0.843928516730014,0.169235594674005,
-0.662566055328992));
#58942=CARTESIAN_POINT('Ctrl Pts',(-0.82417370734834,-0.248180837234624,
-0.652132092726511));
#58943=CARTESIAN_POINT('Ctrl Pts',(-0.61015340756806,-0.607098712803667,
-0.64169813012403));
#58944=CARTESIAN_POINT('Ctrl Pts',(-0.252314213927473,-0.822917714783772,
-0.63126416752155));
#58945=CARTESIAN_POINT('Ctrl Pts',(0.164997811794668,-0.844767275619598,
-0.620830204919069));
#58946=CARTESIAN_POINT('Ctrl Pts',(0.543418302228559,-0.667497248427149,
-0.610396242316589));
#58947=CARTESIAN_POINT('Ctrl Pts',(0.793749990468483,-0.332891845027883,
-0.599962279714107));
#58948=CARTESIAN_POINT('Ctrl Pts',(0.856987344374013,0.0801792955666448,
-0.589528317111628));
#58949=CARTESIAN_POINT('Ctrl Pts',(0.71822472517211,0.474351422477294,-0.579094354509146));
#58950=CARTESIAN_POINT('Ctrl Pts',(0.410169786635162,0.756714460008828,
-0.568660391906666));
#58951=CARTESIAN_POINT('Ctrl Pts',(0.00543397362123488,0.860712785884739,
-0.558226429304186));
#58952=CARTESIAN_POINT('Ctrl Pts',(-0.400582678056834,0.761833017068439,
-0.547792466701704));
#58953=CARTESIAN_POINT('Ctrl Pts',(-0.712178226872656,0.483382044580997,
-0.537358504099225));
#58954=CARTESIAN_POINT('Ctrl Pts',(-0.855906672842221,0.0909933801929833,
-0.526924541496744));
#58955=CARTESIAN_POINT('Ctrl Pts',(-0.797889870143162,-0.322843279282244,
-0.516490578894263));
#58956=CARTESIAN_POINT('Ctrl Pts',(-0.551802924553791,-0.660582742969169,
-0.506056616291783));
#58957=CARTESIAN_POINT('Ctrl Pts',(-0.175650842469447,-0.842616644384952,
-0.495622653689301));
#58958=CARTESIAN_POINT('Ctrl Pts',(0.241903794376119,-0.826037881771305,
-0.485188691086821));
#58959=CARTESIAN_POINT('Ctrl Pts',(0.602439432890687,-0.61475422532353,
-0.47475472848434));
#58960=CARTESIAN_POINT('Ctrl Pts',(0.820974433890951,-0.2585672190209,-0.46432076588186));
#58961=CARTESIAN_POINT('Ctrl Pts',(0.845998043321078,0.158566511444712,
-0.453886803279379));
#58962=CARTESIAN_POINT('Ctrl Pts',(0.671611961205852,0.53832462457136,-0.443452840676899));
#58963=CARTESIAN_POINT('Ctrl Pts',(0.338920626402068,0.791194563210737,
-0.433018878074418));
#58964=CARTESIAN_POINT('Ctrl Pts',(-0.0736574860403522,0.85757250574206,
-0.422584915471938));
#58965=CARTESIAN_POINT('Ctrl Pts',(-0.468873836611143,0.72181254713152,
-0.412150952869457));
#58966=CARTESIAN_POINT('Ctrl Pts',(-0.753572216284693,0.41591458582155,
-0.401716990266977));
#58967=CARTESIAN_POINT('Ctrl Pts',(-0.860646540683597,0.0119816468658661,
-0.391283027664496));
#58968=CARTESIAN_POINT('Ctrl Pts',(-0.764858385013229,-0.394775478894489,
-0.380849065062015));
#58969=CARTESIAN_POINT('Ctrl Pts',(-0.488785917995028,-0.70848031321364,
-0.370415102459535));
#58970=CARTESIAN_POINT('Ctrl Pts',(-0.0975020153382415,-0.855189677720726,
-0.359981139857054));
#58971=CARTESIAN_POINT('Ctrl Pts',(0.316764028941221,-0.800322796004492,
-0.349547177254573));
#58972=CARTESIAN_POINT('Ctrl Pts',(0.656365813791203,-0.556812307990146,
-0.339113214652093));
#58973=CARTESIAN_POINT('Ctrl Pts',(0.841256006403051,-0.182055924541145,
-0.328679252049612));
#58974=CARTESIAN_POINT('Ctrl Pts',(0.827854249784971,0.23561275138288,-0.318245289447132));
#58975=CARTESIAN_POINT('Ctrl Pts',(0.619319465031675,0.597745287618043,
-0.307811326844651));
#58976=CARTESIAN_POINT('Ctrl Pts',(0.264805259104926,0.818983639189149,
-0.297377364242171));
#58977=CARTESIAN_POINT('Ctrl Pts',(-0.152126032912431,0.847179850805376,
-0.286943401639689));
#58978=CARTESIAN_POINT('Ctrl Pts',(-0.533199794350217,0.675687802651953,
-0.276509439037209));
#58979=CARTESIAN_POINT('Ctrl Pts',(-0.788593341292993,0.344929797673643,
-0.266075476434728));
#58980=CARTESIAN_POINT('Ctrl Pts',(-0.858108045553684,-0.0671314227721541,
-0.255641513832248));
#58981=CARTESIAN_POINT('Ctrl Pts',(-0.72535857568816,-0.463369097137432,
-0.245207551229767));
#58982=CARTESIAN_POINT('Ctrl Pts',(-0.421635351879131,-0.750386395459336,
-0.234773588627287));
#58983=CARTESIAN_POINT('Ctrl Pts',(-0.0185285528209956,-0.860530417001193,
-0.224339626024806));
#58984=CARTESIAN_POINT('Ctrl Pts',(0.388945287243328,-0.76783962364223,
-0.213905663422326));
#58985=CARTESIAN_POINT('Ctrl Pts',(0.704741682270798,-0.494161235578589,
-0.203471700819845));
#58986=CARTESIAN_POINT('Ctrl Pts',(0.854422628174538,-0.104005533986035,
-0.193037738217364));
#58987=CARTESIAN_POINT('Ctrl Pts',(0.802710506756149,0.310667480825697,
-0.182603775614884));
#58988=CARTESIAN_POINT('Ctrl Pts',(0.561787298202008,0.652108863993638,
-0.172169813012403));
#58989=CARTESIAN_POINT('Ctrl Pts',(0.188454734446511,0.839850680936056,
-0.161735850409922));
#58990=CARTESIAN_POINT('Ctrl Pts',(-0.22931647807991,0.829614831389831,
-0.151301887807442));
#58991=CARTESIAN_POINT('Ctrl Pts',(-0.59299976270307,0.623864489566942,
-0.140867925204961));
#58992=CARTESIAN_POINT('Ctrl Pts',(-0.81698137021996,0.270995606044551,
-0.130433962602481));
#58993=CARTESIAN_POINT('Ctrl Pts',(-0.837797337716894,-0.00673058913074182,
-0.12347798753416));
#58994=CARTESIAN_POINT('Ctrl Pts',(-0.814921455736579,-0.139942643537184,
-0.12));
#58995=CARTESIAN_POINT('Ctrl Pts',(-0.676565692095429,0.457932546695683,
-0.12));
#58996=CARTESIAN_POINT('Ctrl Pts',(-0.715290549838907,0.406460878340116,
-0.12));
#58997=CARTESIAN_POINT('Ctrl Pts',(-0.761722039381193,0.328281076047502,
-0.12));
#58998=CARTESIAN_POINT('Ctrl Pts',(-0.809780868705113,0.169044693082709,
-0.12));
#58999=CARTESIAN_POINT('Ctrl Pts',(-0.820456584566055,0.110526708837243,
-0.12));
#59000=CARTESIAN_POINT('Ctrl Pts',(-0.829018965506486,-0.0125105404198994,
-0.12));
#59001=CARTESIAN_POINT('Ctrl Pts',(-0.82576831737714,-0.0767786210857246,
-0.12));
#59002=CARTESIAN_POINT('Ctrl Pts',(-0.814921455736578,-0.139942643537185,
-0.12));
#59003=CARTESIAN_POINT('Origin',(0.,0.,0.0794349077448279));
#59004=CARTESIAN_POINT('',(-1.045,-1.27975590510898E-16,-6.93889390390723E-17));
#59005=CARTESIAN_POINT('Origin',(0.,0.,0.));
#59006=CARTESIAN_POINT('',(-1.1,-9.25861368525747E-17,0.0317542648054295));
#59007=CARTESIAN_POINT('',(-1.18258529610859,-1.44824929759811E-16,0.0794349077448279));
#59008=CARTESIAN_POINT('',(-1.1,0.635085296108588,0.130002302030174));
#59009=CARTESIAN_POINT('Ctrl Pts',(-1.1,0.635085296108588,0.130002302030174));
#59010=CARTESIAN_POINT('Ctrl Pts',(-1.1,0.294744111674235,0.0317542648054296));
#59011=CARTESIAN_POINT('Ctrl Pts',(-1.1,-5.04611257989404E-17,0.0317542648054295));
#59012=CARTESIAN_POINT('',(7.77755175064932E-17,1.27017059221718,0.130002302030174));
#59013=CARTESIAN_POINT('Ctrl Pts',(7.77755175064932E-17,1.27017059221718,
0.130002302030174));
#59014=CARTESIAN_POINT('Ctrl Pts',(-0.55,0.952627944162882,-0.0533310313031589));
#59015=CARTESIAN_POINT('Ctrl Pts',(-1.1,0.635085296108588,0.130002302030174));
#59016=CARTESIAN_POINT('',(1.1,0.635085296108588,0.130002302030174));
#59017=CARTESIAN_POINT('Ctrl Pts',(1.1,0.635085296108588,0.130002302030174));
#59018=CARTESIAN_POINT('Ctrl Pts',(0.55,0.952627944162882,-0.0533310313031591));
#59019=CARTESIAN_POINT('Ctrl Pts',(7.77755175064932E-17,1.27017059221718,
0.130002302030174));
#59020=CARTESIAN_POINT('',(1.1,-0.635085296108589,0.130002302030174));
#59021=CARTESIAN_POINT('Ctrl Pts',(1.1,-0.635085296108589,0.130002302030174));
#59022=CARTESIAN_POINT('Ctrl Pts',(1.1,-3.33066907387547E-16,-0.0533310313031591));
#59023=CARTESIAN_POINT('Ctrl Pts',(1.1,0.635085296108588,0.130002302030174));
#59024=CARTESIAN_POINT('',(-2.3332655251948E-16,-1.27017059221718,0.130002302030174));
#59025=CARTESIAN_POINT('Ctrl Pts',(-2.3332655251948E-16,-1.27017059221718,
0.130002302030174));
#59026=CARTESIAN_POINT('Ctrl Pts',(0.55,-0.952627944162883,-0.0533310313031587));
#59027=CARTESIAN_POINT('Ctrl Pts',(1.1,-0.635085296108589,0.130002302030174));
#59028=CARTESIAN_POINT('',(-1.1,-0.635085296108588,0.130002302030174));
#59029=CARTESIAN_POINT('Ctrl Pts',(-1.1,-0.635085296108588,0.130002302030174));
#59030=CARTESIAN_POINT('Ctrl Pts',(-0.55,-0.952627944162882,-0.0533310313031589));
#59031=CARTESIAN_POINT('Ctrl Pts',(-2.3332655251948E-16,-1.27017059221718,
0.130002302030174));
#59032=CARTESIAN_POINT('Ctrl Pts',(-1.1,-5.04611257989404E-17,0.0317542648054295));
#59033=CARTESIAN_POINT('Ctrl Pts',(-1.1,-0.294744111674235,0.0317542648054295));
#59034=CARTESIAN_POINT('Ctrl Pts',(-1.1,-0.635085296108588,0.130002302030174));
#59035=CARTESIAN_POINT('Origin',(-2.3332655251948E-16,-1.27017059221718,
0.));
#59036=CARTESIAN_POINT('',(1.1,-0.635085296108589,0.669997697969826));
#59037=CARTESIAN_POINT('',(1.1,-0.635085296108589,0.));
#59038=CARTESIAN_POINT('',(-2.3332655251948E-16,-1.27017059221718,0.669997697969826));
#59039=CARTESIAN_POINT('Ctrl Pts',(1.1,-0.635085296108589,0.669997697969826));
#59040=CARTESIAN_POINT('Ctrl Pts',(0.55,-0.952627944162883,0.853331031303159));
#59041=CARTESIAN_POINT('Ctrl Pts',(-2.3332655251948E-16,-1.27017059221718,
0.669997697969826));
#59042=CARTESIAN_POINT('',(-2.3332655251948E-16,-1.27017059221718,0.));
#59043=CARTESIAN_POINT('Origin',(1.1,-0.635085296108589,0.));
#59044=CARTESIAN_POINT('',(1.1,0.635085296108588,0.669997697969826));
#59045=CARTESIAN_POINT('',(1.1,0.635085296108588,0.));
#59046=CARTESIAN_POINT('Ctrl Pts',(1.1,0.635085296108588,0.669997697969826));
#59047=CARTESIAN_POINT('Ctrl Pts',(1.1,-3.33066907387547E-16,0.853331031303159));
#59048=CARTESIAN_POINT('Ctrl Pts',(1.1,-0.635085296108589,0.669997697969826));
#59049=CARTESIAN_POINT('Origin',(1.1,0.635085296108588,0.));
#59050=CARTESIAN_POINT('',(7.77755175064932E-17,1.27017059221718,0.669997697969826));
#59051=CARTESIAN_POINT('',(7.77755175064932E-17,1.27017059221718,0.));
#59052=CARTESIAN_POINT('Ctrl Pts',(7.77755175064932E-17,1.27017059221718,
0.669997697969826));
#59053=CARTESIAN_POINT('Ctrl Pts',(0.55,0.952627944162882,0.853331031303159));
#59054=CARTESIAN_POINT('Ctrl Pts',(1.1,0.635085296108588,0.669997697969826));
#59055=CARTESIAN_POINT('Origin',(0.,0.,0.720565092255172));
#59056=CARTESIAN_POINT('',(-1.1,0.635085296108588,0.669997697969826));
#59057=CARTESIAN_POINT('Ctrl Pts',(-1.1,0.635085296108588,0.669997697969826));
#59058=CARTESIAN_POINT('Ctrl Pts',(-0.55,0.952627944162882,0.853331031303159));
#59059=CARTESIAN_POINT('Ctrl Pts',(7.77755175064932E-17,1.27017059221718,
0.669997697969826));
#59060=CARTESIAN_POINT('',(-1.1,-1.43047262651515E-16,0.768245735194571));
#59061=CARTESIAN_POINT('Ctrl Pts',(-1.1,-1.51383377396821E-16,0.768245735194571));
#59062=CARTESIAN_POINT('Ctrl Pts',(-1.1,0.294744111674235,0.768245735194571));
#59063=CARTESIAN_POINT('Ctrl Pts',(-1.1,0.635085296108588,0.669997697969826));
#59064=CARTESIAN_POINT('',(-1.045,-1.27975590510898E-16,0.8));
#59065=CARTESIAN_POINT('',(-1.18258529610859,-1.44824929759811E-16,0.720565092255172));
#59066=CARTESIAN_POINT('Origin',(0.,0.,0.8));
#59067=CARTESIAN_POINT('',(-1.1,-0.635085296108588,0.669997697969826));
#59068=CARTESIAN_POINT('Ctrl Pts',(-1.1,-0.635085296108588,0.669997697969826));
#59069=CARTESIAN_POINT('Ctrl Pts',(-1.1,-0.294744111674235,0.76824573519457));
#59070=CARTESIAN_POINT('Ctrl Pts',(-1.1,-1.51383377396821E-16,0.768245735194571));
#59071=CARTESIAN_POINT('Ctrl Pts',(-2.3332655251948E-16,-1.27017059221718,
0.669997697969826));
#59072=CARTESIAN_POINT('Ctrl Pts',(-0.55,-0.952627944162883,0.853331031303159));
#59073=CARTESIAN_POINT('Ctrl Pts',(-1.1,-0.635085296108588,0.669997697969826));
#59074=CARTESIAN_POINT('Origin',(7.77755175064932E-17,1.27017059221718,
0.));
#59075=CARTESIAN_POINT('',(-1.1,0.635085296108588,0.));
#59076=CARTESIAN_POINT('Origin',(0.,0.,0.8));
#59077=CARTESIAN_POINT('Origin',(0.,0.,0.8));
#59078=CARTESIAN_POINT('',(-0.4,4.89858719658941E-17,0.8));
#59079=CARTESIAN_POINT('Origin',(0.,0.,0.8));
#59080=CARTESIAN_POINT('Origin',(0.,0.,0.));
#59081=CARTESIAN_POINT('',(-0.7431,9.10035036446398E-17,0.));
#59082=CARTESIAN_POINT('Origin',(0.,0.,0.));
#59083=CARTESIAN_POINT('Origin',(0.,0.,0.));
#59084=CARTESIAN_POINT('',(-0.4,-4.89858719658941E-17,0.));
#59085=CARTESIAN_POINT('Origin',(0.,0.,0.));
#59086=CARTESIAN_POINT('Origin',(-1.1,-0.635085296108589,0.));
#59087=CARTESIAN_POINT('',(-1.1,-0.635085296108589,0.));
#59088=CARTESIAN_POINT('Origin',(-1.1,0.635085296108588,0.));
#59089=CARTESIAN_POINT('Origin',(0.,0.,0.0765832901469392));
#59090=CARTESIAN_POINT('',(-0.4,-4.89858719658941E-17,-1.2));
#59091=CARTESIAN_POINT('',(-0.4,-4.89858719658941E-17,0.0765832901469392));
#59092=CARTESIAN_POINT('Origin',(0.,0.,-1.2));
#59093=CARTESIAN_POINT('Origin',(0.,0.,0.0765832901469392));
#59094=CARTESIAN_POINT('',(-0.4,-4.89858719658941E-17,1.35316658029388));
#59095=CARTESIAN_POINT('Origin',(0.,0.,1.35316658029388));
#59096=CARTESIAN_POINT('',(-0.4,-4.89858719658941E-17,0.0765832901469392));
#59097=CARTESIAN_POINT('Origin',(0.7531,0.,-1.2));
#59098=CARTESIAN_POINT('',(-0.7531,-9.22281504437872E-17,-1.2));
#59099=CARTESIAN_POINT('Origin',(0.,0.,-1.2));
#59100=CARTESIAN_POINT('Origin',(0.,0.,-1.16));
#59101=CARTESIAN_POINT('',(-0.7931,-9.71267376403766E-17,-1.16));
#59102=CARTESIAN_POINT('Origin',(0.7431,0.,-0.12));
#59103=CARTESIAN_POINT('',(-0.7431,-9.10035036446398E-17,-0.12));
#59104=CARTESIAN_POINT('Origin',(0.,0.,-0.12));
#59105=CARTESIAN_POINT('Origin',(0.,0.,-0.0349999999999999));
#59106=CARTESIAN_POINT('',(-0.7431,-9.10035036446398E-17,-0.0349999999999999));
#59107=CARTESIAN_POINT('Origin',(0.,0.,2.17));
#59108=CARTESIAN_POINT('',(-0.74,-9.06238631369041E-17,2.2));
#59109=CARTESIAN_POINT('Origin',(0.,0.,2.2));
#59110=CARTESIAN_POINT('',(-0.77,-9.42978035343462E-17,2.17));
#59111=CARTESIAN_POINT('Origin',(0.58,0.,2.2));
#59112=CARTESIAN_POINT('',(-0.58,-7.10295143505465E-17,2.2));
#59113=CARTESIAN_POINT('Origin',(0.,0.,2.2));
#59114=CARTESIAN_POINT('Origin',(0.,0.,1.77658329014694));
#59115=CARTESIAN_POINT('',(-0.49,-6.00076931582203E-17,1.77658329014694));
#59181=UNCERTAINTY_MEASURE_WITH_UNIT(LENGTH_MEASURE(0.001),#59205,
'DISTANCE_ACCURACY_VALUE',
'Maximum model space distance between geometric entities at asserted c
onnectivities');
#59182=UNCERTAINTY_MEASURE_WITH_UNIT(LENGTH_MEASURE(0.001),#59205,
'DISTANCE_ACCURACY_VALUE',
'Maximum model space distance between geometric entities at asserted c
onnectivities');
#59203=(
GEOMETRIC_REPRESENTATION_CONTEXT(3)
GLOBAL_UNCERTAINTY_ASSIGNED_CONTEXT((#59181))
GLOBAL_UNIT_ASSIGNED_CONTEXT((#59205,#59207,#59208))
REPRESENTATION_CONTEXT('','3D')
);
#59204=(
GEOMETRIC_REPRESENTATION_CONTEXT(3)
GLOBAL_UNCERTAINTY_ASSIGNED_CONTEXT((#59182))
GLOBAL_UNIT_ASSIGNED_CONTEXT((#59205,#59207,#59208))
REPRESENTATION_CONTEXT('','3D')
);
#59205=(
LENGTH_UNIT()
NAMED_UNIT(*)
SI_UNIT(.CENTI.,.METRE.)
);
#59207=(
NAMED_UNIT(*)
PLANE_ANGLE_UNIT()
SI_UNIT($,.RADIAN.)
);
#59208=(
NAMED_UNIT(*)
SI_UNIT($,.STERADIAN.)
SOLID_ANGLE_UNIT()
);
#59229=SHAPE_DEFINITION_REPRESENTATION(#59250,#59316);
#59250=PRODUCT_DEFINITION_SHAPE('',$,#59338);
#59316=SHAPE_REPRESENTATION('',(#24996),#59203);
#59317=PRODUCT_DEFINITION_CONTEXT('part definition',#59382,'design');
#59338=PRODUCT_DEFINITION('2026-10-23-00-47-50-726',
'20_Port_Connector_DIN_2353_GE10-LR_G3-8',#59359,#59317);
#59359=PRODUCT_DEFINITION_FORMATION('',$,#59404);
#59382=APPLICATION_CONTEXT(
'Core Data for Automotive Mechanical Design Process');
#59383=PRODUCT_CONTEXT('part definition',#59382,'mechanical');
#59404=PRODUCT('2026-10-23-00-47-50-726',
'20_Port_Connector_DIN_2353_GE10-LR_G3-8',$,(#59383));
#59566=COLOUR_RGB('Light Blue',0.38,0.62,0.78);
#59567=FILL_AREA_STYLE_COLOUR('',#59566);
#59568=FILL_AREA_STYLE('',(#59567));
#59569=SURFACE_STYLE_FILL_AREA(#59568);
#59570=SURFACE_SIDE_STYLE('',(#59569));
#59571=SURFACE_STYLE_USAGE(.BOTH.,#59570);
#59572=PRESENTATION_STYLE_ASSIGNMENT((#59571));
ENDSEC;
END-ISO-10303-21;
